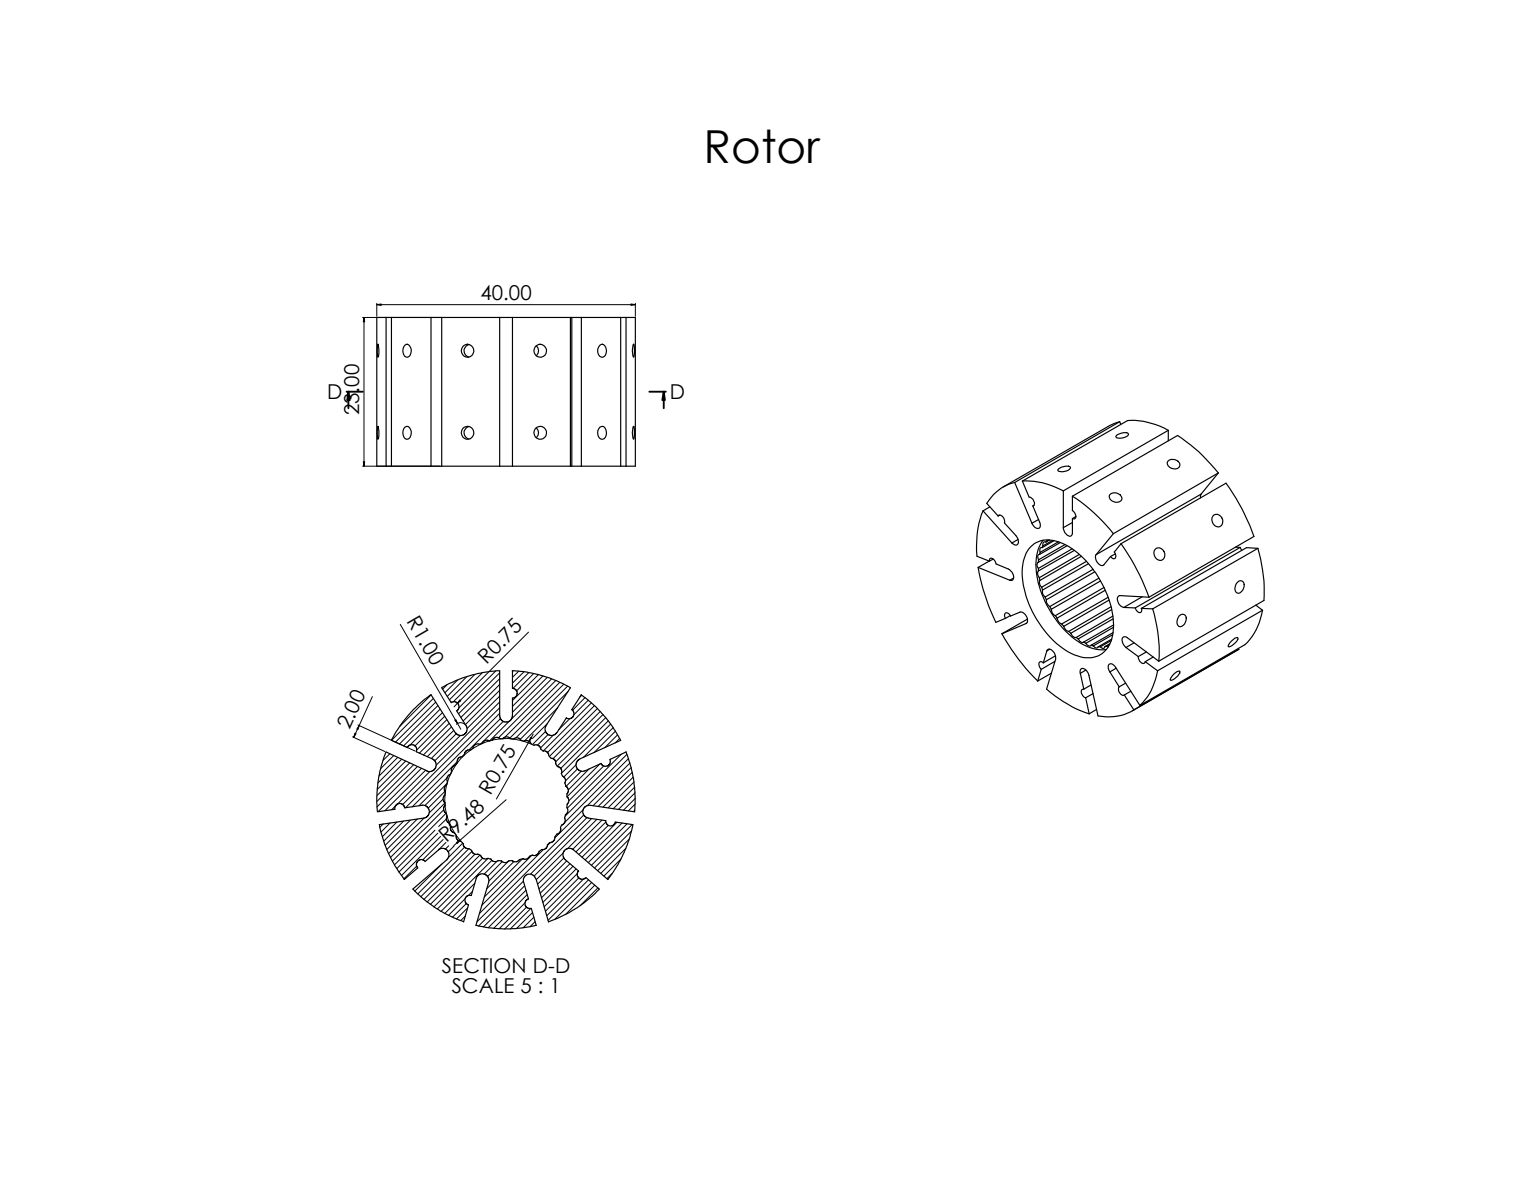
ISO-10303-21;
HEADER;
FILE_DESCRIPTION (('STEP AP214'),
    '1' );
FILE_NAME ('Rotor.step',
    '2026-10-18T20:16:25',
    ( '' ),
    ( '' ),
    'SwSTEP 2.0',
    'SolidWorks 2025',
    '' );
FILE_SCHEMA (( 'AUTOMOTIVE_DESIGN' ));
ENDSEC;

DATA;
#1=FACE_OUTER_BOUND ( 'NONE', #19385, .T. ) ;
#4=AXIS2_PLACEMENT_3D ( 'NONE', #28751, #28908, #7543 ) ;
#8=EDGE_LOOP ( 'NONE', ( #14143, #4167, #13185, #29281 ) ) ;
#11=AXIS2_PLACEMENT_3D ( 'NONE', #21550, #14547, #24043 ) ;
#13=EDGE_LOOP ( 'NONE', ( #16874, #3981 ) ) ;
#16=CARTESIAN_POINT ( 'NONE',  ( 6.437793815610356241, -6.974883619896809606, 1.500000000000001332 ) ) ;
#29=ORIENTED_EDGE ( 'NONE', *, *, #10327, .T. ) ;
#33=CARTESIAN_POINT ( 'NONE',  ( -3.912171961292007616, -8.637616862297829101, 1.500000000000001332 ) ) ;
#37=CARTESIAN_POINT ( 'NONE',  ( -14.84326473672822821, -8.425446036094903945, 20.06253562465620632 ) ) ;
#38=CARTESIAN_POINT ( 'NONE',  ( 0.000000000000000000, 0.000000000000000000, 1.500000000000001332 ) ) ;
#39=EDGE_CURVE ( 'NONE', #26631, #4645, #16306, .T. ) ;
#40=CARTESIAN_POINT ( 'NONE',  ( 4.967306913940536361, 16.28142803850090203, 6.973843882838223429 ) ) ;
#43=ORIENTED_EDGE ( 'NONE', *, *, #8838, .F. ) ;
#45=EDGE_CURVE ( 'NONE', #5916, #3823, #10340, .T. ) ;
#48=CARTESIAN_POINT ( 'NONE',  ( -6.228680293130167911, 19.00574304797303782, 5.679672709359373073 ) ) ;
#49=ORIENTED_EDGE ( 'NONE', *, *, #24996, .T. ) ;
#53=DIRECTION ( 'NONE',  ( 0.8412535328311813165, -0.5406408174555974444, 0.000000000000000000 ) ) ;
#54=DIRECTION ( 'NONE',  ( 0.000000000000000000, 0.000000000000000000, 1.000000000000000000 ) ) ;
#55=ORIENTED_EDGE ( 'NONE', *, *, #18763, .T. ) ;
#56=ORIENTED_EDGE ( 'NONE', *, *, #27505, .T. ) ;
#60=ORIENTED_EDGE ( 'NONE', *, *, #10139, .T. ) ;
#61=CARTESIAN_POINT ( 'NONE',  ( -0.02177409673011774377, -17.02558975896787885, 19.96783386855779341 ) ) ;
#64=CARTESIAN_POINT ( 'NONE',  ( -9.983339604393949074, -17.35078046477759983, 7.441806358946449151 ) ) ;
#65=FACE_OUTER_BOUND ( 'NONE', #13496, .T. ) ;
#66=CARTESIAN_POINT ( 'NONE',  ( 1.363408835038997458, -19.97112866468682668, 19.47783254395485031 ) ) ;
#68=EDGE_CURVE ( 'NONE', #8257, #20089, #6832, .T. ) ;
#70=CARTESIAN_POINT ( 'NONE',  ( 0.000000000000000000, 13.00000000000001421, 1.500000000000001332 ) ) ;
#71=CARTESIAN_POINT ( 'NONE',  ( 14.24237608451263171, 14.06627278277045257, 19.69140814234746273 ) ) ;
#73=ORIENTED_EDGE ( 'NONE', *, *, #24989, .F. ) ;
#75=DIRECTION ( 'NONE',  ( 0.000000000000000000, 0.000000000000000000, 1.000000000000000000 ) ) ;
#76=CARTESIAN_POINT ( 'NONE',  ( -17.59891439103365585, -9.538503746949022144, 6.672349528511551497 ) ) ;
#77=CARTESIAN_POINT ( 'NONE',  ( -13.11527592942575282, -10.04126165406389326, 1.500000000000000000 ) ) ;
#80=EDGE_CURVE ( 'NONE', #24431, #1715, #12846, .T. ) ;
#84=ORIENTED_EDGE ( 'NONE', *, *, #27745, .T. ) ;
#86=DIRECTION ( 'NONE',  ( 0.000000000000000000, 0.000000000000000000, -1.000000000000000000 ) ) ;
#87=VECTOR ( 'NONE', #19138, 1000.000000000000000 ) ;
#90=CARTESIAN_POINT ( 'NONE',  ( 15.47797589786116923, -7.092492006142040673, 19.96783386855779341 ) ) ;
#91=CARTESIAN_POINT ( 'NONE',  ( 6.171684994647412381, 19.04275422834224685, 6.211014596808754007 ) ) ;
#95=CARTESIAN_POINT ( 'NONE',  ( 11.67645754117908830, 12.46194352177089293, 6.892848776733236704 ) ) ;
#96=EDGE_CURVE ( 'NONE', #21713, #6692, #24023, .T. ) ;
#97=FACE_OUTER_BOUND ( 'NONE', #28084, .T. ) ;
#100=CARTESIAN_POINT ( 'NONE',  ( 0.000000000000000000, 0.000000000000000000, 1.500000000000001332 ) ) ;
#104=CARTESIAN_POINT ( 'NONE',  ( -18.38748676655956515, -7.913428453147655084, 6.018569869498933578 ) ) ;
#105=CARTESIAN_POINT ( 'NONE',  ( 14.46116907065692736, 13.81605838820130394, 7.454606537396340826 ) ) ;
#106=CARTESIAN_POINT ( 'NONE',  ( 0.06889080212831104333, -17.02733034922398758, 5.940635272151477686 ) ) ;
#108=LINE ( 'NONE', #21001, #12544 ) ;
#109=CARTESIAN_POINT ( 'NONE',  ( -19.94989956810792009, 1.646935350084928418, 19.89182036555910571 ) ) ;
#112=CARTESIAN_POINT ( 'NONE',  ( 11.47892014274828654, -16.39977715623752275, 20.25542030744407640 ) ) ;
#113=CIRCLE ( 'NONE', #24448, 0.7500000000000007772 ) ;
#115=VERTEX_POINT ( 'NONE', #22003 ) ;
#116=EDGE_LOOP ( 'NONE', ( #16345, #15698, #26338, #11828 ) ) ;
#117=CARTESIAN_POINT ( 'NONE',  ( 4.695984468547702129, 19.44110619659980799, 20.15039051365864253 ) ) ;
#122=CARTESIAN_POINT ( 'NONE',  ( -10.72135862580927146, -16.90494006806149940, 7.632642797338977658 ) ) ;
#125=CARTESIAN_POINT ( 'NONE',  ( 18.71580048965418541, -7.100988023106708624, 19.03762469184452755 ) ) ;
#126=CARTESIAN_POINT ( 'NONE',  ( 16.55849529797290032, 4.179294809495488039, 19.14333282897057842 ) ) ;
#127=EDGE_CURVE ( 'NONE', #8705, #8129, #11228, .T. ) ;
#130=EDGE_CURVE ( 'NONE', #28271, #10764, #20221, .T. ) ;
#133=ORIENTED_EDGE ( 'NONE', *, *, #19082, .T. ) ;
#134=CARTESIAN_POINT ( 'NONE',  ( 7.706848733600953238, 5.524309650260795124, 1.500000000000001332 ) ) ;
#135=CARTESIAN_POINT ( 'NONE',  ( -12.90456292687989759, 11.10871050118981529, 20.05479082170252525 ) ) ;
#136=CARTESIAN_POINT ( 'NONE',  ( -9.972083266784119715, -17.35726207598482773, 18.56793045041961321 ) ) ;
#137=CARTESIAN_POINT ( 'NONE',  ( -15.05112753842527162, -8.020416455032004066, 20.34789198813115263 ) ) ;
#139=CARTESIAN_POINT ( 'NONE',  ( 1.767905995611233072, -16.98559759804142288, 19.61324152429826739 ) ) ;
#140=CARTESIAN_POINT ( 'NONE',  ( 16.82202058066696537, 2.664153601443035146, 18.49267272388512140 ) ) ;
#143=CARTESIAN_POINT ( 'NONE',  ( 11.01999061743883956, -16.71182566173002826, 7.652108011868850035 ) ) ;
#144=CARTESIAN_POINT ( 'NONE',  ( 8.480328572437745294, -4.608906612435629491, 21.50000000000000000 ) ) ;
#147=LINE ( 'NONE', #19489, #17289 ) ;
#149=CARTESIAN_POINT ( 'NONE',  ( 1.000000000000008438, 13.00000000000001421, 1.500000000000001332 ) ) ;
#150=CARTESIAN_POINT ( 'NONE',  ( 2.878478920843521749, -0.8451976705243363641, 24.50000000000000000 ) ) ;
#151=CARTESIAN_POINT ( 'NONE',  ( 12.00212711880201510, 12.12705342296112221, 7.545655578832108468 ) ) ;
#153=CARTESIAN_POINT ( 'NONE',  ( -5.488535287689156661, 19.23255048776057308, 5.775318986477953054 ) ) ;
#154=VERTEX_POINT ( 'NONE', #22460 ) ;
#160=VERTEX_POINT ( 'NONE', #4060 ) ;
#161=CARTESIAN_POINT ( 'NONE',  ( 16.17271416092067682, -5.480318835022405466, 6.995624166085161910 ) ) ;
#174=VECTOR ( 'NONE', #2091, 1000.000000000000000 ) ;
#178=DIRECTION ( 'NONE',  ( 1.000000000000000000, 0.000000000000000000, 0.000000000000000000 ) ) ;
#183=CARTESIAN_POINT ( 'NONE',  ( 4.641725321133337800, 16.38498716464899019, 5.848946451764561516 ) ) ;
#189=EDGE_CURVE ( 'NONE', #1099, #580, #18256, .T. ) ;
#194=VERTEX_POINT ( 'NONE', #13123 ) ;
#195=DIRECTION ( 'NONE',  ( 0.000000000000000000, 0.000000000000000000, 1.000000000000000000 ) ) ;
#197=ORIENTED_EDGE ( 'NONE', *, *, #29811, .T. ) ;
#198=ADVANCED_FACE ( 'NONE', ( #25436 ), #29650, .F. ) ;
#199=ORIENTED_EDGE ( 'NONE', *, *, #12643, .T. ) ;
#200=CARTESIAN_POINT ( 'NONE',  ( -9.658933677579515376, -17.51307076256854600, 6.392525840300335105 ) ) ;
#203=VERTEX_POINT ( 'NONE', #17802 ) ;
#205=CARTESIAN_POINT ( 'NONE',  ( -0.1973194101962232605, -20.01708124257648791, 20.19668224736330941 ) ) ;
#208=DIRECTION ( 'NONE',  ( 0.000000000000000000, 0.000000000000000000, -1.000000000000000000 ) ) ;
#209=CARTESIAN_POINT ( 'NONE',  ( 4.045242219987651211, 16.55840560649980731, 18.34798005863078885 ) ) ;
#211=CARTESIAN_POINT ( 'NONE',  ( 0.8978415369256412815, -19.99755156235223552, 18.50655187082627862 ) ) ;
#212=EDGE_LOOP ( 'NONE', ( #3421, #739, #13868, #11454 ) ) ;
#214=EDGE_CURVE ( 'NONE', #13827, #7727, #27159, .T. ) ;
#216=FACE_OUTER_BOUND ( 'NONE', #25286, .T. ) ;
#220=FACE_OUTER_BOUND ( 'NONE', #17515, .T. ) ;
#221=CARTESIAN_POINT ( 'NONE',  ( -6.449126838413862473, 15.81136745782587383, 6.995624166085161910 ) ) ;
#225=CARTESIAN_POINT ( 'NONE',  ( -18.38748676655957937, -7.913428453147655084, 18.71435384576123440 ) ) ;
#230=AXIS2_PLACEMENT_3D ( 'NONE', #30774, #53, #30611 ) ;
#235=CARTESIAN_POINT ( 'NONE',  ( 11.21631477658334042, -16.55933310271405645, 20.34789198813115618 ) ) ;
#239=CARTESIAN_POINT ( 'NONE',  ( 18.21588581002257001, -8.300927319590597264, 18.39701043959520987 ) ) ;
#240=CARTESIAN_POINT ( 'NONE',  ( 5.984782097461514461, 19.10229623552459088, 5.940635272151477686 ) ) ;
#242=DIRECTION ( 'NONE',  ( 0.000000000000000000, 0.000000000000000000, 1.000000000000000000 ) ) ;
#245=CARTESIAN_POINT ( 'NONE',  ( -0.4564504349075055867, 9.471281197126600659, 13.00000000000000178 ) ) ;
#249=EDGE_CURVE ( 'NONE', #25840, #22179, #829, .T. ) ;
#250=CARTESIAN_POINT ( 'NONE',  ( 0.000000000000000000, 0.000000000000000000, 21.50000000000000000 ) ) ;
#255=CARTESIAN_POINT ( 'NONE',  ( -18.32589276785170185, -8.054604467211150975, 7.429667576816606278 ) ) ;
#256=AXIS2_PLACEMENT_3D ( 'NONE', #17662, #8160, #8483 ) ;
#257=DIRECTION ( 'NONE',  ( 0.000000000000000000, 0.000000000000000000, 1.000000000000000000 ) ) ;
#266=EDGE_CURVE ( 'NONE', #6035, #4843, #28573, .T. ) ;
#267=DIRECTION ( 'NONE',  ( 1.000000000000000000, 0.000000000000000000, 0.000000000000000000 ) ) ;
#269=ORIENTED_EDGE ( 'NONE', *, *, #9974, .T. ) ;
#271=LINE ( 'NONE', #18686, #17607 ) ;
#277=ORIENTED_EDGE ( 'NONE', *, *, #12266, .F. ) ;
#278=CARTESIAN_POINT ( 'NONE',  ( 18.65245237681030588, -7.265846841151810231, 19.97651184436794125 ) ) ;
#279=CARTESIAN_POINT ( 'NONE',  ( 16.55484456677775640, 4.196195780087080607, 19.25672174529527325 ) ) ;
#283=VECTOR ( 'NONE', #6940, 1000.000000000000000 ) ;
#286=CARTESIAN_POINT ( 'NONE',  ( -14.75808792347767628, 13.52460813173914467, 18.90679857307105749 ) ) ;
#287=CARTESIAN_POINT ( 'NONE',  ( -7.919226493207297324, -15.11997014267743289, 18.64703902303423178 ) ) ;
#290=CYLINDRICAL_SURFACE ( 'NONE', #21952, 0.7500000000000006661 ) ;
#294=CARTESIAN_POINT ( 'NONE',  ( -19.73562743738982306, 3.350138464993962284, 18.80699882434806369 ) ) ;
#296=VECTOR ( 'NONE', #25590, 1000.000000000000000 ) ;
#297=CARTESIAN_POINT ( 'NONE',  ( 14.88222593340886668, 13.36111339922579866, 20.34789198813115263 ) ) ;
#298=CYLINDRICAL_SURFACE ( 'NONE', #9820, 0.7500000000000004441 ) ;
#302=DIRECTION ( 'NONE',  ( -0.8412535328311813165, 0.5406408174555974444, 0.000000000000000000 ) ) ;
#304=CARTESIAN_POINT ( 'NONE',  ( -5.119216485953539397, 16.24645747311530641, 7.557577766377196582 ) ) ;
#305=CARTESIAN_POINT ( 'NONE',  ( -6.437683520590124608, 6.962021646281596254, 21.50000000000000000 ) ) ;
#308=ORIENTED_EDGE ( 'NONE', *, *, #27638, .F. ) ;
#310=CARTESIAN_POINT ( 'NONE',  ( -4.668110441710642711, -19.44758969394387194, 24.50000000000000000 ) ) ;
#311=CARTESIAN_POINT ( 'NONE',  ( 7.028330626922776325, 10.93629592680536966, 24.50000000000000000 ) ) ;
#312=ORIENTED_EDGE ( 'NONE', *, *, #28685, .F. ) ;
#314=CARTESIAN_POINT ( 'NONE',  ( 8.637616862297841536, -3.912171961291982747, 13.00000000000000178 ) ) ;
#315=VERTEX_POINT ( 'NONE', #30412 ) ;
#316=CARTESIAN_POINT ( 'NONE',  ( 16.17688602565676348, -5.469326772727310271, 6.341840715582230281 ) ) ;
#318=CARTESIAN_POINT ( 'NONE',  ( 0.7836604620899298990, -17.02735026737547841, 18.34798005863078885 ) ) ;
#321=VERTEX_POINT ( 'NONE', #30556 ) ;
#324=DIRECTION ( 'NONE',  ( 1.000000000000000000, 0.000000000000000000, 0.000000000000000000 ) ) ;
#328=CYLINDRICAL_SURFACE ( 'NONE', #23812, 9.482273699623480212 ) ;
#332=EDGE_CURVE ( 'NONE', #21638, #2008, #29122, .T. ) ;
#336=CARTESIAN_POINT ( 'NONE',  ( 16.91972452348793610, -3.442972353390052920, 1.500000000000000000 ) ) ;
#337=VECTOR ( 'NONE', #30659, 1000.000000000000000 ) ;
#339=FACE_OUTER_BOUND ( 'NONE', #26193, .T. ) ;
#341=CARTESIAN_POINT ( 'NONE',  ( 5.015798959889809616, 16.26549279019889127, 6.519181285484532573 ) ) ;
#343=DIRECTION ( 'NONE',  ( -0.000000000000000000, -0.000000000000000000, 1.000000000000000000 ) ) ;
#345=CARTESIAN_POINT ( 'NONE',  ( 19.63503467057051566, 3.804509661152916333, 7.454606537396342603 ) ) ;
#348=ORIENTED_EDGE ( 'NONE', *, *, #25359, .F. ) ;
#351=FACE_OUTER_BOUND ( 'NONE', #19038, .T. ) ;
#354=CARTESIAN_POINT ( 'NONE',  ( -10.51513057463695233, -17.01270198993486460, 7.652108011868850035 ) ) ;
#357=VERTEX_POINT ( 'NONE', #453 ) ;
#359=CARTESIAN_POINT ( 'NONE',  ( -0.2073672225646059353, -17.02047435233534145, 19.56050940960062690 ) ) ;
#362=CARTESIAN_POINT ( 'NONE',  ( -7.796062812047482637, -15.18940472835275202, 6.131018562779544823 ) ) ;
#363=DIRECTION ( 'NONE',  ( -0.000000000000000000, -0.000000000000000000, 1.000000000000000000 ) ) ;
#364=CARTESIAN_POINT ( 'NONE',  ( 1.771654956907828593, -16.98531529776322202, 19.58863275299554019 ) ) ;
#366=EDGE_CURVE ( 'NONE', #13283, #3383, #19165, .T. ) ;
#367=CARTESIAN_POINT ( 'NONE',  ( 18.44250036706182883, -7.738792361249056562, 5.679672709359370408 ) ) ;
#368=FACE_OUTER_BOUND ( 'NONE', #3082, .T. ) ;
#369=CARTESIAN_POINT ( 'NONE',  ( 12.30438418247798538, 11.79938075381829066, 18.34838970509067479 ) ) ;
#370=FACE_OUTER_BOUND ( 'NONE', #17110, .T. ) ;
#372=EDGE_LOOP ( 'NONE', ( #10343, #19396, #30364, #16527 ) ) ;
#373=CIRCLE ( 'NONE', #4356, 0.9999999999999983347 ) ;
#377=CARTESIAN_POINT ( 'NONE',  ( -18.02600256144196322, -8.705149951716492751, 5.652605728828375753 ) ) ;
#378=CARTESIAN_POINT ( 'NONE',  ( -6.670428619809865900, 18.87372120578243795, 5.951255046771932733 ) ) ;
#379=CARTESIAN_POINT ( 'NONE',  ( -19.93457197822652205, 1.617270501065028565, 7.161525567826883432 ) ) ;
#382=CARTESIAN_POINT ( 'NONE',  ( -5.544451647051928944, 16.11829164193971664, 20.34789198813115263 ) ) ;
#383=LINE ( 'NONE', #24396, #15077 ) ;
#387=AXIS2_PLACEMENT_3D ( 'NONE', #10424, #20235, #11043 ) ;
#389=CARTESIAN_POINT ( 'NONE',  ( -5.000852292258041842, 19.36469665082833913, 19.47728749465736797 ) ) ;
#397=ADVANCED_FACE ( 'NONE', ( #26495 ), #10383, .T. ) ;
#399=CARTESIAN_POINT ( 'NONE',  ( 5.016833900951455760, 16.26516650762552629, 19.45164628100866722 ) ) ;
#400=AXIS2_PLACEMENT_3D ( 'NONE', #13486, #9091, #27970 ) ;
#402=VECTOR ( 'NONE', #2368, 1000.000000000000114 ) ;
#410=CARTESIAN_POINT ( 'NONE',  ( -18.36135251343596764, -7.973951480934441172, 7.359006845440219102 ) ) ;
#413=CARTESIAN_POINT ( 'NONE',  ( 14.20332585465778941, 14.08077620357340720, 6.919864475265769421 ) ) ;
#414=EDGE_CURVE ( 'NONE', #2072, #12805, #10900, .T. ) ;
#415=CARTESIAN_POINT ( 'NONE',  ( -0.08542884365699662808, -20.01766063302414622, 5.749228751562096562 ) ) ;
#420=ORIENTED_EDGE ( 'NONE', *, *, #14601, .T. ) ;
#424=CARTESIAN_POINT ( 'NONE',  ( -7.869584159753960861, 10.39565510934976977, 1.500000000000001332 ) ) ;
#425=CARTESIAN_POINT ( 'NONE',  ( 5.041560023644209743, 19.35451993181656860, 7.626218077512944227 ) ) ;
#428=ORIENTED_EDGE ( 'NONE', *, *, #24835, .F. ) ;
#435=CARTESIAN_POINT ( 'NONE',  ( 15.37106698384762993, 12.82394120857654052, 20.05479082170252525 ) ) ;
#437=CARTESIAN_POINT ( 'NONE',  ( -11.28665222577991578, -16.53262428680031704, 6.211014596808754007 ) ) ;
#439=CARTESIAN_POINT ( 'NONE',  ( 18.73437065802030332, -7.051821425362959417, 19.25672174529527325 ) ) ;
#440=CARTESIAN_POINT ( 'NONE',  ( -15.42727847259664564, 12.72856271945105178, 20.34789198813115263 ) ) ;
#446=AXIS2_PLACEMENT_3D ( 'NONE', #2104, #16459, #7100 ) ;
#452=CARTESIAN_POINT ( 'NONE',  ( -6.485206790418931888, 15.79815780198024910, 19.58863275299554019 ) ) ;
#453=CARTESIAN_POINT ( 'NONE',  ( -10.51100883930069863, -17.01524884273342053, 5.652196082369965069 ) ) ;
#456=CARTESIAN_POINT ( 'NONE',  ( -7.857295329535767259, -15.15488436941561368, 18.73743063545763121 ) ) ;
#458=CARTESIAN_POINT ( 'NONE',  ( 11.23874228076938664, -11.06161525231356713, 24.50000000000000000 ) ) ;
#459=CYLINDRICAL_SURFACE ( 'NONE', #7899, 0.7499999999999988898 ) ;
#461=CARTESIAN_POINT ( 'NONE',  ( 9.833055564703258256, -13.92194044488497440, 5.651989602109218858 ) ) ;
#464=CARTESIAN_POINT ( 'NONE',  ( -13.42620032052775692, 10.50496109755573748, 7.652108011868850035 ) ) ;
#466=VERTEX_POINT ( 'NONE', #10733 ) ;
#467=ORIENTED_EDGE ( 'NONE', *, *, #5596, .F. ) ;
#470=CARTESIAN_POINT ( 'NONE',  ( 18.71829317531096137, -7.044536951825319804, 19.48477075383301482 ) ) ;
#476=CARTESIAN_POINT ( 'NONE',  ( 19.74251403343738076, 3.198927889078825970, 18.34798005863226678 ) ) ;
#485=LINE ( 'NONE', #28719, #30455 ) ;
#487=CARTESIAN_POINT ( 'NONE',  ( 0.7220001660362483920, 9.454746441592963180, 21.50000000000000000 ) ) ;
#493=ORIENTED_EDGE ( 'NONE', *, *, #4835, .T. ) ;
#497=CARTESIAN_POINT ( 'NONE',  ( -1.000000000000008438, 19.97498435543819539, 24.50000000000000000 ) ) ;
#499=CARTESIAN_POINT ( 'NONE',  ( -15.13309390500916862, -7.848982836665745921, 20.34789198813115263 ) ) ;
#500=FACE_OUTER_BOUND ( 'NONE', #7541, .T. ) ;
#515=CIRCLE ( 'NONE', #3019, 9.482273699623480212 ) ;
#516=ORIENTED_EDGE ( 'NONE', *, *, #6379, .T. ) ;
#524=CARTESIAN_POINT ( 'NONE',  ( 14.19872765237045442, 14.11031447301239972, 19.36813350477385143 ) ) ;
#529=CARTESIAN_POINT ( 'NONE',  ( -6.227270323482350101, 15.89124769393590952, 7.366751648393900176 ) ) ;
#530=CARTESIAN_POINT ( 'NONE',  ( -19.85983307072121917, 2.367331911061644867, 7.652108011868850923 ) ) ;
#531=CARTESIAN_POINT ( 'NONE',  ( -18.41388790264795361, -7.851569931599773788, 18.80699882434806369 ) ) ;
#536=CARTESIAN_POINT ( 'NONE',  ( 7.856594496258195726, 4.390207617113981442, 21.50000000000000000 ) ) ;
#537=CARTESIAN_POINT ( 'NONE',  ( -5.971396161871752817, 19.08775596758252036, 20.34789198813115263 ) ) ;
#538=CARTESIAN_POINT ( 'NONE',  ( -14.93957691572895818, 13.32381478560234456, 7.429667576816606278 ) ) ;
#539=CARTESIAN_POINT ( 'NONE',  ( 0.7788148816922453310, -17.02744011591805062, 7.652108011868850923 ) ) ;
#540=VERTEX_POINT ( 'NONE', #28613 ) ;
#542=CARTESIAN_POINT ( 'NONE',  ( 18.26182835180409825, -8.199456719779961489, 18.36582235739946611 ) ) ;
#550=CARTESIAN_POINT ( 'NONE',  ( -18.04156136322729864, -8.631457789788587576, 5.652196082369963293 ) ) ;
#553=CIRCLE ( 'NONE', #9509, 9.482273699623480212 ) ;
#554=CARTESIAN_POINT ( 'NONE',  ( 4.608906612435600181, 7.730328572437758616, 1.500000000000001332 ) ) ;
#555=FACE_OUTER_BOUND ( 'NONE', #28008, .T. ) ;
#560=CARTESIAN_POINT ( 'NONE',  ( -0.2365265214052943432, -17.01953242238517916, 6.641371103590088865 ) ) ;
#561=CARTESIAN_POINT ( 'NONE',  ( -17.20435420003449423, -1.463329469628170898, -0.6213203435596476032 ) ) ;
#562=DIRECTION ( 'NONE',  ( 0.000000000000000000, 0.000000000000000000, 1.000000000000000000 ) ) ;
#565=ORIENTED_EDGE ( 'NONE', *, *, #7868, .T. ) ;
#567=DIRECTION ( 'NONE',  ( -0.000000000000000000, -0.000000000000000000, -1.000000000000000000 ) ) ;
#573=ORIENTED_EDGE ( 'NONE', *, *, #29979, .F. ) ;
#575=EDGE_CURVE ( 'NONE', #3557, #18473, #9892, .T. ) ;
#576=CIRCLE ( 'NONE', #3574, 0.7500000000000006661 ) ;
#577=CARTESIAN_POINT ( 'NONE',  ( 12.83215063165194891, 11.19227874472585782, 20.05479082170252525 ) ) ;
#578=EDGE_CURVE ( 'NONE', #11969, #7607, #20097, .T. ) ;
#579=CARTESIAN_POINT ( 'NONE',  ( -11.35279153858833112, -16.48728705952963480, 6.864725433338323413 ) ) ;
#580=VERTEX_POINT ( 'NONE', #9273 ) ;
#581=CARTESIAN_POINT ( 'NONE',  ( 18.72830449397920560, -7.068013160879066170, 19.14333282897057842 ) ) ;
#585=DIRECTION ( 'NONE',  ( 0.000000000000000000, 0.000000000000000000, -1.000000000000000000 ) ) ;
#586=ADVANCED_FACE ( 'NONE', ( #19241 ), #28765, .F. ) ;
#588=AXIS2_PLACEMENT_3D ( 'NONE', #26078, #13640, #11903 ) ;
#590=EDGE_CURVE ( 'NONE', #23467, #4066, #18123, .T. ) ;
#592=CARTESIAN_POINT ( 'NONE',  ( -6.227270323482350989, 15.89124769393590597, 20.06253562465620632 ) ) ;
#593=CARTESIAN_POINT ( 'NONE',  ( -14.83674576813424295, 13.43848929326658492, 18.71435384576123440 ) ) ;
#595=ADVANCED_FACE ( 'NONE', ( #370 ), #16451, .F. ) ;
#596=CARTESIAN_POINT ( 'NONE',  ( -13.00999358272542494, -0.8602714556717691030, 24.50000000000000000 ) ) ;
#599=CARTESIAN_POINT ( 'NONE',  ( -16.96556290498877573, 1.647560670993253540, 5.652196082368482699 ) ) ;
#602=CARTESIAN_POINT ( 'NONE',  ( 11.02326084422093189, -16.70928013427648651, 5.657991946698900598 ) ) ;
#605=CARTESIAN_POINT ( 'NONE',  ( 9.013259606643902799, -14.43917691233135869, 6.782064869129510676 ) ) ;
#606=VERTEX_POINT ( 'NONE', #11765 ) ;
#609=CARTESIAN_POINT ( 'NONE',  ( 10.58932223943305573, -16.96688107778387078, 5.849008070840548079 ) ) ;
#611=LINE ( 'NONE', #7792, #3910 ) ;
#612=CARTESIAN_POINT ( 'NONE',  ( -15.57738559309033022, -6.860713375568460393, 6.714907520933425467 ) ) ;
#615=CARTESIAN_POINT ( 'NONE',  ( 1.000000000000008438, 13.00000000000001421, 1.500000000000001332 ) ) ;
#619=CARTESIAN_POINT ( 'NONE',  ( -17.67829152986844932, -9.353438168054493573, 18.73377938172347612 ) ) ;
#621=CARTESIAN_POINT ( 'NONE',  ( 19.77852387640474419, 3.085824932809442700, 5.657991946698900598 ) ) ;
#622=ORIENTED_EDGE ( 'NONE', *, *, #14546, .F. ) ;
#623=CARTESIAN_POINT ( 'NONE',  ( 15.53918631077679002, 12.61944498292910488, 6.420335371522007506 ) ) ;
#624=VERTEX_POINT ( 'NONE', #8174 ) ;
#625=CARTESIAN_POINT ( 'NONE',  ( 16.02044690728356002, -5.868896442471958963, 7.500147780736496017 ) ) ;
#632=ADVANCED_FACE ( 'NONE', ( #17214 ), #5675, .F. ) ;
#633=LINE ( 'NONE', #12185, #27245 ) ;
#637=CARTESIAN_POINT ( 'NONE',  ( -0.9307681286967850465, 9.436481611552762772, 21.50000000000000000 ) ) ;
#638=B_SPLINE_CURVE_WITH_KNOTS ( 'NONE', 3,
 ( #10726, #17744, #5592, #22265, #17916, #1379, #29923, #19940, #29760, #20545, #30064, #27580, #15559, #5738, #25226, #3871, #15086, #13394, #22884, #24604 ),
 .UNSPECIFIED., .F., .F.,
 ( 4, 2, 2, 2, 2, 2, 2, 2, 2, 4 ),
 ( 0.000000000000000000, 0.06250000000000163758, 0.1250000000000032752, 0.1875000000000049127, 0.2187500000000050793, 0.2500000000000052180, 0.3125000000000038858, 0.3750000000000024980, 0.4375000000000011657, 0.4999999999999999445 ),
 .UNSPECIFIED. ) ;
#644=CARTESIAN_POINT ( 'NONE',  ( -13.66451197432776965, 10.21236830578559918, 18.44527579819791185 ) ) ;
#658=CIRCLE ( 'NONE', #6650, 0.7500000000000006661 ) ;
#659=ORIENTED_EDGE ( 'NONE', *, *, #21172, .T. ) ;
#668=ORIENTED_EDGE ( 'NONE', *, *, #12074, .F. ) ;
#669=EDGE_LOOP ( 'NONE', ( #23306, #14404 ) ) ;
#670=CARTESIAN_POINT ( 'NONE',  ( 0.7453234696411419336, -17.02803278171227674, 18.34777357837151968 ) ) ;
#675=DIRECTION ( 'NONE',  ( 0.000000000000000000, 0.000000000000000000, 1.000000000000000000 ) ) ;
#678=CARTESIAN_POINT ( 'NONE',  ( 8.884323311075775109, 1.438332125858202692, 1.500000000000001332 ) ) ;
#679=CARTESIAN_POINT ( 'NONE',  ( 14.74830145734719089, 13.53506178006322891, 20.32367522806703874 ) ) ;
#681=VERTEX_POINT ( 'NONE', #999 ) ;
#684=CARTESIAN_POINT ( 'NONE',  ( -6.938992678473721476, 18.77645360485809789, 6.560937769032974209 ) ) ;
#685=CARTESIAN_POINT ( 'NONE',  ( 11.39819190923272707, -16.45610177916887551, 5.704143890883081269 ) ) ;
#690=LINE ( 'NONE', #10519, #25476 ) ;
#692=CARTESIAN_POINT ( 'NONE',  ( -14.74940038399478581, 13.53421240139457815, 7.080843742048788414 ) ) ;
#694=EDGE_LOOP ( 'NONE', ( #14179, #5997 ) ) ;
#696=DIRECTION ( 'NONE',  ( -0.9096319953545185522, 0.4154150130018859355, 0.000000000000000000 ) ) ;
#697=CARTESIAN_POINT ( 'NONE',  ( 4.045241160018716364, 16.55840174602107595, 5.652196082367002106 ) ) ;
#700=B_SPLINE_CURVE_WITH_KNOTS ( 'NONE', 3,
 ( #539, #9908, #28941, #10375, #29405, #8043, #19573, #24706, #22379, #17544, #10211, #12880, #15348, #17078, #3348, #1015, #7576, #26756, #29090, #24878 ),
 .UNSPECIFIED., .F., .F.,
 ( 4, 2, 2, 2, 2, 2, 2, 2, 2, 4 ),
 ( 0.000000000000000000, 0.06249999999999977102, 0.1249999999999995420, 0.1874999999999993061, 0.2187499999999992228, 0.2499999999999990841, 0.3124999999999992228, 0.3749999999999993894, 0.4374999999999995559, 0.4999999999999997224 ),
 .UNSPECIFIED. ) ;
#714=LINE ( 'NONE', #29114, #23280 ) ;
#720=CARTESIAN_POINT ( 'NONE',  ( 5.296161872597630271, 19.28602264385381204, 7.652108011868850035 ) ) ;
#723=ORIENTED_EDGE ( 'NONE', *, *, #19288, .F. ) ;
#725=CARTESIAN_POINT ( 'NONE',  ( -1.687027447297492211, -8.840471615930066918, 1.500000000000001332 ) ) ;
#728=CARTESIAN_POINT ( 'NONE',  ( 15.04472583903954153, 13.20536594261729491, 18.36582235739946611 ) ) ;
#735=CARTESIAN_POINT ( 'NONE',  ( -4.163336342344337027E-14, 1.387778780781445676E-14, 24.50000000000000000 ) ) ;
#736=AXIS2_PLACEMENT_3D ( 'NONE', #3166, #5043, #14695 ) ;
#739=ORIENTED_EDGE ( 'NONE', *, *, #127, .T. ) ;
#741=CARTESIAN_POINT ( 'NONE',  ( 16.55484456677776706, 4.196195780087079719, 6.560937769032974209 ) ) ;
#746=FACE_OUTER_BOUND ( 'NONE', #4867, .T. ) ;
#748=CARTESIAN_POINT ( 'NONE',  ( 9.027514758752763768, -14.43064536408543219, 6.864725433338323413 ) ) ;
#755=DIRECTION ( 'NONE',  ( -0.9096319953545185522, 0.4154150130018859355, 0.000000000000000000 ) ) ;
#758=DIRECTION ( 'NONE',  ( 0.000000000000000000, 0.000000000000000000, -1.000000000000000000 ) ) ;
#759=ORIENTED_EDGE ( 'NONE', *, *, #25056, .T. ) ;
#760=CARTESIAN_POINT ( 'NONE',  ( 12.35846533491531041, 11.73919094685904696, 7.652108011868850923 ) ) ;
#764=CARTESIAN_POINT ( 'NONE',  ( -9.636724589035640776, -17.52522580332708557, 19.48477075383299706 ) ) ;
#768=FACE_OUTER_BOUND ( 'NONE', #4197, .T. ) ;
#770=EDGE_CURVE ( 'NONE', #13440, #321, #29228, .T. ) ;
#771=CARTESIAN_POINT ( 'NONE',  ( 12.95659581195171484, 11.04149104205339782, 7.080843742048788414 ) ) ;
#773=CARTESIAN_POINT ( 'NONE',  ( 18.72830449397920560, -7.068013160879066170, 6.447548852708279377 ) ) ;
#777=ORIENTED_EDGE ( 'NONE', *, *, #17280, .T. ) ;
#778=VECTOR ( 'NONE', #21130, 1000.000000000000000 ) ;
#780=CARTESIAN_POINT ( 'NONE',  ( -8.743977807160097981, -3.668292057955969021, 1.500000000000001332 ) ) ;
#785=CARTESIAN_POINT ( 'NONE',  ( 9.085188746210622668, -14.39608436040015960, 19.77662771831109367 ) ) ;
#788=EDGE_LOOP ( 'NONE', ( #7005, #12290, #10451, #7760 ) ) ;
#803=EDGE_CURVE ( 'NONE', #26662, #24952, #7407, .T. ) ;
#805=AXIS2_PLACEMENT_3D ( 'NONE', #19527, #29041, #19830 ) ;
#809=ORIENTED_EDGE ( 'NONE', *, *, #12803, .T. ) ;
#810=AXIS2_PLACEMENT_3D ( 'NONE', #29533, #8170, #12389 ) ;
#811=VECTOR ( 'NONE', #29749, 1000.000000000000000 ) ;
#825=CARTESIAN_POINT ( 'NONE',  ( 0.000000000000000000, 0.000000000000000000, 21.50000000000000000 ) ) ;
#829=B_SPLINE_CURVE_WITH_KNOTS ( 'NONE', 3,
 ( #14168, #27929, #2173, #18565, #16516, #23839, #2018, #21343, #6847, #30856, #9500, #11688, #18868, #16207, #16370, #4814, #25727, #4355, #28382, #13880 ),
 .UNSPECIFIED., .F., .F.,
 ( 4, 2, 2, 2, 2, 2, 2, 2, 2, 4 ),
 ( 0.000000000000000000, 0.06250000000000092981, 0.1250000000000018596, 0.1875000000000027756, 0.2187500000000024980, 0.2500000000000022204, 0.3125000000000016653, 0.3750000000000010547, 0.4375000000000004996, 0.4999999999999998890 ),
 .UNSPECIFIED. ) ;
#830=EDGE_LOOP ( 'NONE', ( #15023, #29937 ) ) ;
#832=CARTESIAN_POINT ( 'NONE',  ( 10.50506478158603230, 13.32952022457704544, -0.6213203435596476032 ) ) ;
#834=CARTESIAN_POINT ( 'NONE',  ( 12.35846532919128116, 11.73919094318043221, 20.34789198813115263 ) ) ;
#836=EDGE_CURVE ( 'NONE', #12567, #28720, #7238, .T. ) ;
#837=EDGE_LOOP ( 'NONE', ( #26502, #26520, #16395, #29491 ) ) ;
#840=AXIS2_PLACEMENT_3D ( 'NONE', #28772, #2576, #21589 ) ;
#841=CARTESIAN_POINT ( 'NONE',  ( -17.99620775894062064, -8.766556869501982874, 7.643931100913408550 ) ) ;
#843=CARTESIAN_POINT ( 'NONE',  ( 10.52132926683980685, -13.44281371605820752, 6.041646659195333058 ) ) ;
#850=CARTESIAN_POINT ( 'NONE',  ( -1.438332125858111432, 8.884323311075791096, 1.500000000000001332 ) ) ;
#851=CARTESIAN_POINT ( 'NONE',  ( -14.94322542805485554, 13.31996107294430765, 5.862424720655265098 ) ) ;
#852=PLANE ( 'NONE',  #17635 ) ;
#856=CYLINDRICAL_SURFACE ( 'NONE', #7221, 0.7499999999999997780 ) ;
#860=VECTOR ( 'NONE', #3364, 1000.000000000000000 ) ;
#863=VERTEX_POINT ( 'NONE', #2675 ) ;
#866=CARTESIAN_POINT ( 'NONE',  ( 0.3518703668723790479, -19.99690444156084013, 20.34789198813115263 ) ) ;
#870=CARTESIAN_POINT ( 'NONE',  ( -19.71440049134194084, 3.368233808196385404, 18.84056766331481825 ) ) ;
#873=DIRECTION ( 'NONE',  ( 0.000000000000000000, 0.000000000000000000, 1.000000000000000000 ) ) ;
#875=VECTOR ( 'NONE', #3921, 1000.000000000000000 ) ;
#879=PLANE ( 'NONE',  #17324 ) ;
#881=DIRECTION ( 'NONE',  ( -1.000000000000000000, 0.000000000000000000, 0.000000000000000000 ) ) ;
#882=ORIENTED_EDGE ( 'NONE', *, *, #25559, .F. ) ;
#883=CARTESIAN_POINT ( 'NONE',  ( 7.730328572437743517, -4.608906612435629491, 1.500000000000001332 ) ) ;
#884=AXIS2_PLACEMENT_3D ( 'NONE', #30746, #18912, #29927 ) ;
#885=DIRECTION ( 'NONE',  ( -0.8412535328311804284, 0.5406408174555987767, 0.000000000000000000 ) ) ;
#887=EDGE_LOOP ( 'NONE', ( #3868, #22327 ) ) ;
#891=( LENGTH_UNIT ( ) NAMED_UNIT ( * ) SI_UNIT ( .MILLI., .METRE. ) );
#893=CARTESIAN_POINT ( 'NONE',  ( 9.634323311075775109, 1.438332125858202692, 1.500000000000001332 ) ) ;
#894=CIRCLE ( 'NONE', #1872, 0.7500000000000006661 ) ;
#895=CARTESIAN_POINT ( 'NONE',  ( 14.97043017101258577, 13.28903844302880266, 18.35377592296120497 ) ) ;
#896=B_SPLINE_CURVE_WITH_KNOTS ( 'NONE', 3,
 ( #27424, #24449, #15392, #24916, #17910, #27106, #10419, #1219, #17442, #15223, #5729, #19935, #10719, #3089, #7769, #29600, #22103, #29450 ),
 .UNSPECIFIED., .F., .F.,
 ( 4, 2, 2, 2, 2, 2, 2, 2, 4 ),
 ( 0.003174295595554312618, 0.003570702171545548417, 0.003967108747536783782, 0.004363515323528019581, 0.004759921899519255380, 0.005156328475510491179, 0.005552735051501726977, 0.005949141627492962776, 0.006345548203484198575 ),
 .UNSPECIFIED. ) ;
#899=CARTESIAN_POINT ( 'NONE',  ( 15.98415658701446773, -5.958736450466529000, 20.25542030744407640 ) ) ;
#900=CARTESIAN_POINT ( 'NONE',  ( 16.68770897235364714, 3.522277800415037685, 20.29915277494337644 ) ) ;
#904=CIRCLE ( 'NONE', #7825, 9.482273699623480212 ) ;
#908=ORIENTED_EDGE ( 'NONE', *, *, #23214, .F. ) ;
#912=B_SPLINE_SURFACE_WITH_KNOTS ( 'NONE', 3, 1, ( 
 ( #20892, #1721 ),
 ( #25123, #18111 ),
 ( #30417, #8743 ),
 ( #8909, #16074 ),
 ( #27626, #4067 ),
 ( #9055, #4210 ),
 ( #8463, #13733 ),
 ( #23223, #11236 ),
 ( #22779, #13284 ),
 ( #18433, #10949 ),
 ( #17965, #27323 ),
 ( #6250, #1583 ),
 ( #15450, #27934 ),
 ( #27474, #6562 ),
 ( #1877, #13128 ),
 ( #2491, #21500 ),
 ( #14491, #28223 ),
 ( #28389, #7014 ),
 ( #30705, #26190 ),
 ( #294, #21040 ),
 ( #9355, #7330 ),
 ( #6855, #16840 ),
 ( #2640, #30562 ),
 ( #25890, #19171 ),
 ( #23680, #21832 ),
 ( #16216, #18713 ),
 ( #28692, #2023 ),
 ( #12159, #28538 ),
 ( #6701, #11852 ),
 ( #4821, #23533 ),
 ( #16375, #4519 ) ),
 .UNSPECIFIED., .F., .F., .F.,
 ( 4, 3, 3, 3, 3, 3, 3, 3, 3, 3, 4 ),
 ( 2, 2 ),
 ( 0.000000000000000000, 0.05425176834609614362, 0.1085332949128348518, 0.1623767749169379715, 0.2157504826133058717, 0.2688657508888169789, 0.3218907763505471364, 0.3749548578363334772, 0.4282048033836237666, 0.4818374082110496448, 0.4999999999131650164 ),
 ( 0.000000000000000000, 1.000000000000000000 ),
 .UNSPECIFIED. ) ;
#913=CARTESIAN_POINT ( 'NONE',  ( 19.59419491516168321, 4.095680178559270246, 7.098451512883313441 ) ) ;
#914=CARTESIAN_POINT ( 'NONE',  ( -15.07239450771860056, 13.17334274624126422, 18.44501272782439827 ) ) ;
#915=AXIS2_PLACEMENT_3D ( 'NONE', #16296, #11613, #18792 ) ;
#916=AXIS2_PLACEMENT_3D ( 'NONE', #10436, #27126, #12313 ) ;
#917=CARTESIAN_POINT ( 'NONE',  ( -7.809214384344184801, -15.18204291278971496, 19.89182036555910571 ) ) ;
#920=FACE_OUTER_BOUND ( 'NONE', #25459, .T. ) ;
#922=CARTESIAN_POINT ( 'NONE',  ( 9.054000795813635705, -14.41483084819681615, 6.310736198168394928 ) ) ;
#925=CARTESIAN_POINT ( 'NONE',  ( 12.86767874445214055, -1.850092897552706894, 1.500000000000001332 ) ) ;
#929=LINE ( 'NONE', #17619, #19604 ) ;
#930=DIRECTION ( 'NONE',  ( -0.000000000000000000, -0.000000000000000000, -1.000000000000000000 ) ) ;
#933=DIRECTION ( 'NONE',  ( 1.000000000000000000, 0.000000000000000000, 0.000000000000000000 ) ) ;
#934=CARTESIAN_POINT ( 'NONE',  ( 6.237549684377459158, 19.00251437819605371, 6.913388067999410858 ) ) ;
#936=EDGE_LOOP ( 'NONE', ( #6511, #6269, #30437, #7742 ) ) ;
#940=CARTESIAN_POINT ( 'NONE',  ( -5.881244434206279514, -6.812559277181949646, 1.500000000000001332 ) ) ;
#943=CARTESIAN_POINT ( 'NONE',  ( 19.84141769772507402, 2.653416696629036675, 7.500898271101006820 ) ) ;
#950=VERTEX_POINT ( 'NONE', #12191 ) ;
#951=ADVANCED_FACE ( 'NONE', ( #21689 ), #328, .F. ) ;
#952=CARTESIAN_POINT ( 'NONE',  ( 4.316117848019423775, 19.54676362458759087, 6.672349528511551497 ) ) ;
#957=B_SPLINE_CURVE_WITH_KNOTS ( 'NONE', 3,
 ( #20118, #27608, #5770, #27144, #14969, #24482, #12648, #27299, #19967, #764, #10288, #19803, #8121, #29331, #15263, #7972, #17476, #17627 ),
 .UNSPECIFIED., .F., .F.,
 ( 4, 2, 2, 2, 2, 2, 2, 2, 4 ),
 ( 0.000000000000000000, 0.0003967869494442840357, 0.0007935738988885680713, 0.001190360848332851999, 0.001587147797777136143, 0.001983934747221420287, 0.002380721696665703997, 0.002777508646109988141, 0.003174295595554272285 ),
 .UNSPECIFIED. ) ;
#959=CARTESIAN_POINT ( 'NONE',  ( 10.26079415706018771, -17.18817258638080148, 19.45164628100866722 ) ) ;
#964=CARTESIAN_POINT ( 'NONE',  ( -13.78503626495110446, 10.05991541429405522, 18.56793045041961321 ) ) ;
#966=CARTESIAN_POINT ( 'NONE',  ( -13.00999358272542494, -0.8602714556717691030, 24.50000000000000000 ) ) ;
#970=CARTESIAN_POINT ( 'NONE',  ( -16.96496224101209194, 1.652369717150043549, 20.34789198813115263 ) ) ;
#971=CARTESIAN_POINT ( 'NONE',  ( 12.69259498021937382, 11.35795912679306063, 7.526951045817046548 ) ) ;
#972=DIRECTION ( 'NONE',  ( 0.000000000000000000, 0.000000000000000000, 1.000000000000000000 ) ) ;
#974=VECTOR ( 'NONE', #27914, 1000.000000000000000 ) ;
#982=ORIENTED_EDGE ( 'NONE', *, *, #8425, .T. ) ;
#983=EDGE_CURVE ( 'NONE', #14509, #24952, #16713, .T. ) ;
#984=VERTEX_POINT ( 'NONE', #21071 ) ;
#985=EDGE_CURVE ( 'NONE', #23990, #4772, #30594, .T. ) ;
#990=EDGE_CURVE ( 'NONE', #6958, #27304, #16554, .T. ) ;
#998=CARTESIAN_POINT ( 'NONE',  ( 1.121436987360518778, -17.01878714021720285, 5.704143890883081269 ) ) ;
#999=CARTESIAN_POINT ( 'NONE',  ( -5.971396161871753705, 19.08775596758252391, 7.652108011868850035 ) ) ;
#1000=EDGE_CURVE ( 'NONE', #203, #4677, #25923, .T. ) ;
#1001=VERTEX_POINT ( 'NONE', #4552 ) ;
#1002=EDGE_CURVE ( 'NONE', #25635, #16019, #6828, .T. ) ;
#1003=CARTESIAN_POINT ( 'NONE',  ( -9.310272263096074141, -14.25176022191445036, 18.90679857307105749 ) ) ;
#1005=CARTESIAN_POINT ( 'NONE',  ( -5.615427697021304176, 16.09608755218563303, 7.652108011868850035 ) ) ;
#1007=CARTESIAN_POINT ( 'NONE',  ( 10.65192122195201740, -13.34697535456212236, 6.341840715582230281 ) ) ;
#1009=CARTESIAN_POINT ( 'NONE',  ( -15.34307810681595896, 12.82926163924266660, 20.34789198813115263 ) ) ;
#1010=ORIENTED_EDGE ( 'NONE', *, *, #24861, .F. ) ;
#1012=CARTESIAN_POINT ( 'NONE',  ( -4.622016212553093695, -12.19167610014704906, 1.500000000000001332 ) ) ;
#1014=CARTESIAN_POINT ( 'NONE',  ( -13.30790957887532677, 10.64596135573641789, 5.657991946698900598 ) ) ;
#1015=CARTESIAN_POINT ( 'NONE',  ( 0.1624814966347698231, -17.02900520012292773, 5.848946451764563292 ) ) ;
#1018=CYLINDRICAL_SURFACE ( 'NONE', #7276, 9.482273699623480212 ) ;
#1020=ADVANCED_FACE ( 'NONE', ( #2831 ), #21857, .F. ) ;
#1027=ORIENTED_EDGE ( 'NONE', *, *, #5345, .F. ) ;
#1040=B_SPLINE_CURVE_WITH_KNOTS ( 'NONE', 3,
 ( #16024, #18829, #21137, #6657, #4166, #1985, #30215, #28346, #16174, #11647, #6973, #9156, #11797, #18669, #13992, #27731, #11507, #18382 ),
 .UNSPECIFIED., .F., .F.,
 ( 4, 2, 2, 2, 2, 2, 2, 2, 4 ),
 ( 0.003174295595554314786, 0.003570702171545546248, 0.003967108747536777710, 0.004363515323528009172, 0.004759921899519240635, 0.005156328475510472097, 0.005552735051501703559, 0.005949141627492935021, 0.006345548203484166483 ),
 .UNSPECIFIED. ) ;
#1047=CARTESIAN_POINT ( 'NONE',  ( 4.307942169702170254, 19.53053083060024164, 6.523620417364449864 ) ) ;
#1050=CARTESIAN_POINT ( 'NONE',  ( 0.3567158762617958501, -19.99681059701335073, 5.652196082369963293 ) ) ;
#1055=ADVANCED_FACE ( 'NONE', ( #7822 ), #17334, .F. ) ;
#1057=CARTESIAN_POINT ( 'NONE',  ( 15.43499236066653779, -3.229500095980124996, -0.6213203435596476032 ) ) ;
#1060=CARTESIAN_POINT ( 'NONE',  ( -16.88948989945504664, 2.193765388987378717, 7.500898271101006820 ) ) ;
#1064=LINE ( 'NONE', #19936, #27451 ) ;
#1066=CARTESIAN_POINT ( 'NONE',  ( -5.419526071899103847, 16.15737324489262150, 20.34789198813115974 ) ) ;
#1069=ORIENTED_EDGE ( 'NONE', *, *, #15299, .F. ) ;
#1072=CARTESIAN_POINT ( 'NONE',  ( 19.66823596311669675, 3.724077645907917677, 7.500147780736496017 ) ) ;
#1075=CARTESIAN_POINT ( 'NONE',  ( -9.228184491630887720, -14.30775539772383098, 7.267659094423555288 ) ) ;
#1079=CARTESIAN_POINT ( 'NONE',  ( 11.83189508704695392, -16.14673651688228873, 18.82680253904184298 ) ) ;
#1083=ORIENTED_EDGE ( 'NONE', *, *, #14308, .T. ) ;
#1087=ORIENTED_EDGE ( 'NONE', *, *, #30330, .F. ) ;
#1088=CYLINDRICAL_SURFACE ( 'NONE', #4116, 1.000000000000007772 ) ;
#1089=EDGE_CURVE ( 'NONE', #3823, #5916, #13380, .T. ) ;
#1090=DIRECTION ( 'NONE',  ( -0.000000000000000000, -0.000000000000000000, -1.000000000000000000 ) ) ;
#1092=CARTESIAN_POINT ( 'NONE',  ( 6.236311564447694522, 19.00292092786887110, 6.386539667786099272 ) ) ;
#1093=ORIENTED_EDGE ( 'NONE', *, *, #990, .F. ) ;
#1097=CARTESIAN_POINT ( 'NONE',  ( 14.29853178503251954, 14.00938365128603280, 6.131018562779544823 ) ) ;
#1098=CARTESIAN_POINT ( 'NONE',  ( 16.87995935610571507, 2.188012981718273853, 6.641371103590088865 ) ) ;
#1099=VERTEX_POINT ( 'NONE', #8461 ) ;
#1100=CARTESIAN_POINT ( 'NONE',  ( 16.09518941752841670, 6.251081041772567737, -0.6213203435596476032 ) ) ;
#1102=CARTESIAN_POINT ( 'NONE',  ( -13.38160118231794371, 10.55829203257429860, 18.34798005863078885 ) ) ;
#1107=DIRECTION ( 'NONE',  ( 0.000000000000000000, 0.000000000000000000, -1.000000000000000000 ) ) ;
#1121=CARTESIAN_POINT ( 'NONE',  ( -14.93932203929705871, 13.29757777824903897, 20.14992337338002670 ) ) ;
#1126=ORIENTED_EDGE ( 'NONE', *, *, #17165, .T. ) ;
#1128=DIRECTION ( 'NONE',  ( -0.000000000000000000, -0.000000000000000000, 1.000000000000000000 ) ) ;
#1130=VERTEX_POINT ( 'NONE', #6559 ) ;
#1136=CARTESIAN_POINT ( 'NONE',  ( -19.94474618696874302, 1.485631111656367853, 19.48477075383299706 ) ) ;
#1137=EDGE_LOOP ( 'NONE', ( #14626, #9572, #10175, #26189 ) ) ;
#1142=DIRECTION ( 'NONE',  ( 0.000000000000000000, 0.000000000000000000, 1.000000000000000000 ) ) ;
#1145=CARTESIAN_POINT ( 'NONE',  ( 14.84769773172387985, 13.42619037096054591, 20.34789198813115263 ) ) ;
#1147=VERTEX_POINT ( 'NONE', #6092 ) ;
#1148=CARTESIAN_POINT ( 'NONE',  ( -11.13550902248300467, -16.63501148641496030, 20.05479082170252525 ) ) ;
#1149=CARTESIAN_POINT ( 'NONE',  ( -17.77905984561984098, -9.199004478715986366, 7.441806358946449151 ) ) ;
#1150=CARTESIAN_POINT ( 'NONE',  ( -5.423201226159623189, 16.15625638772824502, 5.651492010659114662 ) ) ;
#1152=CARTESIAN_POINT ( 'NONE',  ( 11.93399590641349306, -16.07127689286907213, 6.447548852708279377 ) ) ;
#1164=CARTESIAN_POINT ( 'NONE',  ( -14.72475726066618407, 13.56098618572340442, 6.310736198168394928 ) ) ;
#1165=ADVANCED_FACE ( 'NONE', ( #8741 ), #16133, .T. ) ;
#1171=CARTESIAN_POINT ( 'NONE',  ( -9.356685943497543789, -14.22000274044912160, 6.974106381145714018 ) ) ;
#1173=ORIENTED_EDGE ( 'NONE', *, *, #8480, .F. ) ;
#1174=CARTESIAN_POINT ( 'NONE',  ( -10.82521593960875528, 5.400395169024524655, 1.500000000000001332 ) ) ;
#1175=B_SPLINE_SURFACE_WITH_KNOTS ( 'NONE', 3, 1, ( 
 ( #26290, #11788 ),
 ( #9611, #5083 ),
 ( #21293, #28788 ),
 ( #7428, #21129 ),
 ( #7116, #16935 ),
 ( #16774, #4761 ),
 ( #21451, #26453 ),
 ( #16628, #14594 ),
 ( #28338, #9915 ),
 ( #12256, #12109 ),
 ( #19428, #24098 ),
 ( #25990, #4926 ),
 ( #21759, #2119 ),
 ( #26133, #399 ),
 ( #14443, #17084 ),
 ( #26611, #2439 ),
 ( #5238, #23945 ),
 ( #30648, #16474 ),
 ( #4619, #14268 ),
 ( #23787, #11960 ),
 ( #2591, #10382 ),
 ( #12886, #2903 ),
 ( #17403, #13035 ),
 ( #12725, #22065 ),
 ( #22525, #19727 ),
 ( #20039, #19896 ),
 ( #12421, #29097 ),
 ( #5542, #24409 ),
 ( #15044, #18287 ),
 ( #10531, #27808 ),
 ( #29413, #17551 ) ),
 .UNSPECIFIED., .F., .F., .F.,
 ( 4, 3, 3, 3, 3, 3, 3, 3, 3, 3, 4 ),
 ( 2, 2 ),
 ( 0.000000000000000000, 0.05425176834609614362, 0.1085332949128348518, 0.1623767749169379715, 0.2157504826133058717, 0.2688657508888169789, 0.3218907763505471364, 0.3749548578363334772, 0.4282048033836237666, 0.4818374082110496448, 0.4999999999131652384 ),
 ( 0.000000000000000000, 1.000000000000000000 ),
 .UNSPECIFIED. ) ;
#1178=CARTESIAN_POINT ( 'NONE',  ( 0.000000000000000000, 0.000000000000000000, 1.500000000000001332 ) ) ;
#1180=ORIENTED_EDGE ( 'NONE', *, *, #8394, .T. ) ;
#1182=EDGE_CURVE ( 'NONE', #25305, #3669, #9352, .T. ) ;
#1186=CARTESIAN_POINT ( 'NONE',  ( 16.74250988114177474, 3.198928528055117404, 18.34798005863078885 ) ) ;
#1188=VERTEX_POINT ( 'NONE', #2021 ) ;
#1190=DIRECTION ( 'NONE',  ( 0.000000000000000000, 0.000000000000000000, 1.000000000000000000 ) ) ;
#1198=ADVANCED_FACE ( 'NONE', ( #30415 ), #16212, .F. ) ;
#1204=ADVANCED_FACE ( 'NONE', ( #746 ), #459, .F. ) ;
#1206=FACE_OUTER_BOUND ( 'NONE', #15379, .T. ) ;
#1207=CIRCLE ( 'NONE', #5672, 0.7500000000000011102 ) ;
#1211=ORIENTED_EDGE ( 'NONE', *, *, #13206, .F. ) ;
#1213=CARTESIAN_POINT ( 'NONE',  ( 9.031466002702407181, -14.42835478804157390, 19.08155846658118904 ) ) ;
#1216=ORIENTED_EDGE ( 'NONE', *, *, #25747, .F. ) ;
#1217=ORIENTED_EDGE ( 'NONE', *, *, #11109, .T. ) ;
#1219=CARTESIAN_POINT ( 'NONE',  ( 17.92140030663551187, -8.878400182913017247, 6.913388067999403752 ) ) ;
#1223=CARTESIAN_POINT ( 'NONE',  ( -4.573988094335678767, 16.39521158297133852, 19.41069149716888020 ) ) ;
#1224=EDGE_LOOP ( 'NONE', ( #18742, #29323, #2067, #24627 ) ) ;
#1227=LINE ( 'NONE', #6051, #29164 ) ;
#1230=CARTESIAN_POINT ( 'NONE',  ( 16.70510464924394967, 3.421819763545496773, 5.678370764302467677 ) ) ;
#1235=DIRECTION ( 'NONE',  ( 1.000000000000000000, 0.000000000000000000, 0.000000000000000000 ) ) ;
#1239=FACE_OUTER_BOUND ( 'NONE', #5088, .T. ) ;
#1240=DIRECTION ( 'NONE',  ( 0.000000000000000000, 0.000000000000000000, 1.000000000000000000 ) ) ;
#1242=VERTEX_POINT ( 'NONE', #7485 ) ;
#1245=CARTESIAN_POINT ( 'NONE',  ( -4.718303904200451981, 16.35736724179926682, 7.176035686813569292 ) ) ;
#1251=EDGE_LOOP ( 'NONE', ( #20084, #3933, #13079, #18206 ) ) ;
#1253=CARTESIAN_POINT ( 'NONE',  ( 11.67039530559479843, 12.46804495696167692, 6.447548852708279377 ) ) ;
#1254=CARTESIAN_POINT ( 'NONE',  ( 16.82340201860978368, 2.653416696629036675, 7.500898271101006820 ) ) ;
#1255=VERTEX_POINT ( 'NONE', #2637 ) ;
#1256=CARTESIAN_POINT ( 'NONE',  ( 15.31102578509455903, 12.89549683364648835, 5.862424720655265098 ) ) ;
#1258=CYLINDRICAL_SURFACE ( 'NONE', #28879, 9.482273699623480212 ) ;
#1259=AXIS2_PLACEMENT_3D ( 'NONE', #19682, #29205, #29053 ) ;
#1263=CARTESIAN_POINT ( 'NONE',  ( 5.159688198573268991, 19.34150021954530274, 7.643931100913408550 ) ) ;
#1266=CARTESIAN_POINT ( 'NONE',  ( 6.262045289545328686, 18.99438835075423881, 19.21471108562414543 ) ) ;
#1270=CARTESIAN_POINT ( 'NONE',  ( 16.86926274317444552, 2.283828795636141162, 19.77662771831109367 ) ) ;
#1273=CARTESIAN_POINT ( 'NONE',  ( 15.54925513364909939, -6.943479002078030149, 7.429667576816606278 ) ) ;
#1274=CARTESIAN_POINT ( 'NONE',  ( -13.97362136398187538, 9.814707526993059261, 19.69140814234746273 ) ) ;
#1279=CARTESIAN_POINT ( 'NONE',  ( 9.864937699929955173, -13.90063973435163724, 5.652196082368482699 ) ) ;
#1281=CARTESIAN_POINT ( 'NONE',  ( -5.865338193562683600, 19.13956943172006220, 20.34789198813115263 ) ) ;
#1283=DIRECTION ( 'NONE',  ( 0.000000000000000000, 0.000000000000000000, -1.000000000000000000 ) ) ;
#1290=VERTEX_POINT ( 'NONE', #3249 ) ;
#1291=CIRCLE ( 'NONE', #19710, 1.000000000000008660 ) ;
#1292=VERTEX_POINT ( 'NONE', #17293 ) ;
#1303=DIRECTION ( 'NONE',  ( 1.000000000000000000, 0.000000000000000000, 0.000000000000000000 ) ) ;
#1305=CARTESIAN_POINT ( 'NONE',  ( -8.835414383224243551, -14.56605378991199196, 20.29090034784956131 ) ) ;
#1312=AXIS2_PLACEMENT_3D ( 'NONE', #15629, #1609, #6117 ) ;
#1313=DIRECTION ( 'NONE',  ( 1.000000000000000000, 0.000000000000000000, 0.000000000000000000 ) ) ;
#1318=FACE_OUTER_BOUND ( 'NONE', #10044, .T. ) ;
#1319=DIRECTION ( 'NONE',  ( 0.000000000000000000, 0.000000000000000000, -1.000000000000000000 ) ) ;
#1320=ORIENTED_EDGE ( 'NONE', *, *, #3335, .T. ) ;
#1323=CARTESIAN_POINT ( 'NONE',  ( -9.389232999038370053, -14.19758896559616979, 6.530762810602277924 ) ) ;
#1324=ORIENTED_EDGE ( 'NONE', *, *, #21960, .T. ) ;
#1325=CARTESIAN_POINT ( 'NONE',  ( -8.550548372801090480, -14.74545326687210434, 20.34789198813115263 ) ) ;
#1338=CARTESIAN_POINT ( 'NONE',  ( 12.98116905410817523, 11.01127998639621275, 19.66962785902261146 ) ) ;
#1339=CARTESIAN_POINT ( 'NONE',  ( 16.12178322344232129, -5.613588367463943740, 6.037360021877315575 ) ) ;
#1342=CARTESIAN_POINT ( 'NONE',  ( -17.05006382469673198, 0.8465830298419860789, 7.269896094239230777 ) ) ;
#1345=CARTESIAN_POINT ( 'NONE',  ( 4.608906612435600181, 7.730328572437758616, 1.500000000000001332 ) ) ;
#1347=LINE ( 'NONE', #3692, #2454 ) ;
#1348=CARTESIAN_POINT ( 'NONE',  ( 9.031466002689079176, -14.42835478804960303, 6.385774490351133537 ) ) ;
#1350=CARTESIAN_POINT ( 'NONE',  ( -8.978548835276082940, -14.47379921341572562, 20.22273502201483097 ) ) ;
#1354=VECTOR ( 'NONE', #16103, 1000.000000000000000 ) ;
#1355=ADVANCED_FACE ( 'NONE', ( #21970 ), #24617, .F. ) ;
#1363=CARTESIAN_POINT ( 'NONE',  ( 9.640932123821245980, -14.04859418178019759, 20.32222155561918697 ) ) ;
#1364=VERTEX_POINT ( 'NONE', #5132 ) ;
#1366=CARTESIAN_POINT ( 'NONE',  ( 15.94288127717318915, -6.058927977062414705, 20.29915277494337644 ) ) ;
#1367=CIRCLE ( 'NONE', #19785, 0.7500000000000006661 ) ;
#1368=CARTESIAN_POINT ( 'NONE',  ( 16.70665413472816496, 3.412884783584985815, 20.32367522806703874 ) ) ;
#1370=CARTESIAN_POINT ( 'NONE',  ( -10.62006778255435613, -16.96839658127461803, 18.35377592296120497 ) ) ;
#1373=CARTESIAN_POINT ( 'NONE',  ( -5.544451647051928944, 16.11829164193971664, 20.34789198813115263 ) ) ;
#1374=ADVANCED_FACE ( 'NONE', ( #920 ), #26827, .T. ) ;
#1377=EDGE_CURVE ( 'NONE', #14465, #15390, #21818, .T. ) ;
#1379=CARTESIAN_POINT ( 'NONE',  ( -16.84831847207179223, 2.450595477917709264, 19.96344307082652492 ) ) ;
#1381=AXIS2_PLACEMENT_3D ( 'NONE', #28177, #18216, #23028 ) ;
#1382=EDGE_CURVE ( 'NONE', #4772, #14537, #29775, .T. ) ;
#1385=CARTESIAN_POINT ( 'NONE',  ( 19.57830992477560272, 4.170884463583997892, 6.892848776733236704 ) ) ;
#1386=CARTESIAN_POINT ( 'NONE',  ( -13.16299300229363567, 10.81582545713520638, 18.39701043959520987 ) ) ;
#1387=AXIS2_PLACEMENT_3D ( 'NONE', #12324, #3117, #21827 ) ;
#1388=CARTESIAN_POINT ( 'NONE',  ( 1.307979816591920308, -17.01201364160250051, 5.759928666072750225 ) ) ;
#1389=EDGE_CURVE ( 'NONE', #6566, #2038, #8416, .T. ) ;
#1390=CARTESIAN_POINT ( 'NONE',  ( 16.74328841314636662, 3.194145055459935545, 20.34789198813115263 ) ) ;
#1391=DIRECTION ( 'NONE',  ( 0.000000000000000000, 0.000000000000000000, 1.000000000000000000 ) ) ;
#1392=CARTESIAN_POINT ( 'NONE',  ( 9.749114229549594057, -0.1262659238204522361, 1.500000000000001332 ) ) ;
#1395=EDGE_CURVE ( 'NONE', #29287, #2154, #4898, .T. ) ;
#1396=CIRCLE ( 'NONE', #28285, 1.000000000000004441 ) ;
#1399=AXIS2_PLACEMENT_3D ( 'NONE', #12089, #14577, #5219 ) ;
#1402=ADVANCED_FACE ( 'NONE', ( #8251, #17927, #1686 ), #10739, .T. ) ;
#1405=CARTESIAN_POINT ( 'NONE',  ( -5.147812317479952604, 19.34466387292043876, 7.176035686813569292 ) ) ;
#1406=ORIENTED_EDGE ( 'NONE', *, *, #6377, .F. ) ;
#1417=EDGE_CURVE ( 'NONE', #22306, #24939, #17759, .T. ) ;
#1425=EDGE_CURVE ( 'NONE', #11023, #8165, #6059, .T. ) ;
#1430=ORIENTED_EDGE ( 'NONE', *, *, #26299, .F. ) ;
#1431=CARTESIAN_POINT ( 'NONE',  ( 9.676137610658589239, -14.02562811695956313, 18.36582235739946611 ) ) ;
#1432=CARTESIAN_POINT ( 'NONE',  ( 19.76130408545751749, 3.194145055459935101, 20.34789198813115263 ) ) ;
#1435=CARTESIAN_POINT ( 'NONE',  ( 17.97060409579513163, -8.818932628521070072, 6.211014596808754007 ) ) ;
#1437=CARTESIAN_POINT ( 'NONE',  ( 4.982076346116049770, 19.38816267120398962, 20.29915277494337644 ) ) ;
#1441=B_SPLINE_SURFACE_WITH_KNOTS ( 'NONE', 3, 1, ( 
 ( #29652, #10011 ),
 ( #10154, #29183 ),
 ( #7990, #8289 ),
 ( #26541, #17333 ),
 ( #14675, #24179 ),
 ( #5642, #19983 ),
 ( #7669, #5485 ),
 ( #17171, #19826 ),
 ( #14987, #24499 ),
 ( #26692, #3145 ),
 ( #22161, #785 ),
 ( #22317, #17493 ),
 ( #24654, #3289 ),
 ( #959, #14833 ),
 ( #29501, #17645 ),
 ( #5789, #27780 ),
 ( #6247, #6091 ),
 ( #25439, #15602 ),
 ( #15756, #20444 ),
 ( #10777, #25277 ),
 ( #6558, #20889 ),
 ( #20291, #30414 ),
 ( #17805, #15927 ),
 ( #13281, #23220 ),
 ( #22775, #30259 ),
 ( #3603, #18430 ),
 ( #6409, #1431 ),
 ( #3925, #18108 ),
 ( #27623, #25120 ),
 ( #16070, #3762 ),
 ( #1874, #15445 ) ),
 .UNSPECIFIED., .F., .F., .F.,
 ( 4, 3, 3, 3, 3, 3, 3, 3, 3, 3, 4 ),
 ( 2, 2 ),
 ( 0.000000000000000000, 0.05425176834609614362, 0.1085332949128348518, 0.1623767749169379715, 0.2157504826133058717, 0.2688657508888169789, 0.3218907763505471364, 0.3749548578363334772, 0.4282048033836237666, 0.4818374082110496448, 0.4999999999131654604 ),
 ( 0.000000000000000000, 1.000000000000000000 ),
 .UNSPECIFIED. ) ;
#1445=FACE_OUTER_BOUND ( 'NONE', #22621, .T. ) ;
#1457=EDGE_LOOP ( 'NONE', ( #8273, #15549, #9451, #27302 ) ) ;
#1459=CARTESIAN_POINT ( 'NONE',  ( -19.72672318758257148, 3.296256974645884075, 7.267242832833948007 ) ) ;
#1461=DIRECTION ( 'NONE',  ( -0.000000000000000000, -0.000000000000000000, 1.000000000000000000 ) ) ;
#1465=DIRECTION ( 'NONE',  ( 1.000000000000000000, 0.000000000000000000, 0.000000000000000000 ) ) ;
#1467=DIRECTION ( 'NONE',  ( -1.000000000000000000, 0.000000000000000000, 0.000000000000000000 ) ) ;
#1470=CARTESIAN_POINT ( 'NONE',  ( 1.082887659287353754, -19.98847979319445756, 5.951255046771932733 ) ) ;
#1476=CARTESIAN_POINT ( 'NONE',  ( 10.22519205257000863, -13.65449557370669176, 7.559636331181775581 ) ) ;
#1486=FACE_OUTER_BOUND ( 'NONE', #16197, .T. ) ;
#1487=EDGE_CURVE ( 'NONE', #29934, #18617, #5750, .T. ) ;
#1491=ADVANCED_FACE ( 'NONE', ( #27743 ), #18226, .T. ) ;
#1495=CARTESIAN_POINT ( 'NONE',  ( 19.58194293052861212, 4.068188588073703649, 18.84486140012300126 ) ) ;
#1498=CIRCLE ( 'NONE', #2484, 0.7500000000000011102 ) ;
#1502=CARTESIAN_POINT ( 'NONE',  ( 12.00027744594693324, 12.12900492880153891, 18.45571264222803975 ) ) ;
#1503=DIRECTION ( 'NONE',  ( 0.000000000000000000, 0.000000000000000000, -1.000000000000000000 ) ) ;
#1504=CARTESIAN_POINT ( 'NONE',  ( 0.8643805006890388221, -19.98168094404549322, 18.47531940416305929 ) ) ;
#1506=CARTESIAN_POINT ( 'NONE',  ( -16.99797872337272153, 1.390050218453713349, 7.652108011868849147 ) ) ;
#1520=CARTESIAN_POINT ( 'NONE',  ( 9.184330860358528525, -14.33603326865607741, 18.72771030977186868 ) ) ;
#1525=CARTESIAN_POINT ( 'NONE',  ( -11.25351117620539121, -16.53363456493219985, 18.84056766331481825 ) ) ;
#1527=CARTESIAN_POINT ( 'NONE',  ( 15.05691039802739084, 13.16451011206821242, 7.626647697317575414 ) ) ;
#1532=CARTESIAN_POINT ( 'NONE',  ( -14.93131746129344961, -8.256826158564470219, 5.759928666072747561 ) ) ;
#1538=CARTESIAN_POINT ( 'NONE',  ( 0.01267125088587631523, -20.01782649599895691, 7.595116371587256054 ) ) ;
#1539=CARTESIAN_POINT ( 'NONE',  ( -9.908187358984028137, -17.39367339311968053, 20.06253562465620632 ) ) ;
#1540=CARTESIAN_POINT ( 'NONE',  ( -17.02473723647801052, 1.129071356443817065, 20.24143955528809258 ) ) ;
#1541=CARTESIAN_POINT ( 'NONE',  ( -17.04940614979727798, 0.8516807413325224729, 18.73743063545763121 ) ) ;
#1546=ORIENTED_EDGE ( 'NONE', *, *, #14387, .F. ) ;
#1550=CARTESIAN_POINT ( 'NONE',  ( -15.34618562042307310, 12.82554431217321245, 5.652196082369965069 ) ) ;
#1552=CARTESIAN_POINT ( 'NONE',  ( -5.103338407348687156, 19.35644909001343450, 6.211014596808754007 ) ) ;
#1556=EDGE_CURVE ( 'NONE', #15672, #2241, #10408, .T. ) ;
#1557=CARTESIAN_POINT ( 'NONE',  ( -13.29701885124480576, 10.65950381936556113, 5.651492010659111997 ) ) ;
#1561=DIRECTION ( 'NONE',  ( -0.000000000000000000, -0.000000000000000000, -1.000000000000000000 ) ) ;
#1562=CARTESIAN_POINT ( 'NONE',  ( 2.094186647214742347, -9.248129367672074608, 1.500000000000001332 ) ) ;
#1564=VERTEX_POINT ( 'NONE', #23356 ) ;
#1567=EDGE_CURVE ( 'NONE', #23779, #9215, #4782, .T. ) ;
#1573=CARTESIAN_POINT ( 'NONE',  ( 3.215610563331066540, 16.76717343535964844, 7.196036389296800451 ) ) ;
#1576=CARTESIAN_POINT ( 'NONE',  ( 5.545588074468605022, 19.21617731956021302, 18.37250658438899009 ) ) ;
#1580=DIRECTION ( 'NONE',  ( 1.000000000000000000, 0.000000000000000000, 0.000000000000000000 ) ) ;
#1581=CARTESIAN_POINT ( 'NONE',  ( 19.89498243266959676, 2.215034284604904702, 19.11611934778430921 ) ) ;
#1583=CARTESIAN_POINT ( 'NONE',  ( -16.82187727961403922, 2.603938281378752162, 19.66989035740801839 ) ) ;
#1585=CARTESIAN_POINT ( 'NONE',  ( -14.01239083805804597, 9.763392886517387126, 6.560937769032974209 ) ) ;
#1586=CARTESIAN_POINT ( 'NONE',  ( 5.298969250677085796, 19.30368332842023094, 18.34798005862662507 ) ) ;
#1594=CARTESIAN_POINT ( 'NONE',  ( -5.023839636758346217, 19.37724795171757819, 19.11611934778430921 ) ) ;
#1595=FACE_OUTER_BOUND ( 'NONE', #5843, .T. ) ;
#1599=CARTESIAN_POINT ( 'NONE',  ( -5.846240454020377619, 19.12690956503888629, 7.652108011868849147 ) ) ;
#1600=VERTEX_POINT ( 'NONE', #6818 ) ;
#1603=CARTESIAN_POINT ( 'NONE',  ( -19.87001189204712759, 2.428856360474549447, 7.652108011868850035 ) ) ;
#1609=DIRECTION ( 'NONE',  ( -0.000000000000000000, -0.000000000000000000, -1.000000000000000000 ) ) ;
#1610=CARTESIAN_POINT ( 'NONE',  ( -19.85983307072122628, 2.367331911061644423, 20.34789198813115618 ) ) ;
#1612=CARTESIAN_POINT ( 'NONE',  ( 0.2238118478526182897, -19.99918941848005360, 5.651480102388688032 ) ) ;
#1613=CARTESIAN_POINT ( 'NONE',  ( -5.881244434206279514, -6.812559277181949646, 1.500000000000001332 ) ) ;
#1614=AXIS2_PLACEMENT_3D ( 'NONE', #4560, #28279, #9547 ) ;
#1617=LINE ( 'NONE', #20922, #5360 ) ;
#1618=LINE ( 'NONE', #23264, #22771 ) ;
#1619=CARTESIAN_POINT ( 'NONE',  ( 1.265447379378153769, -19.97763032565216079, 7.098451512883313441 ) ) ;
#1620=CARTESIAN_POINT ( 'NONE',  ( -16.87879800889955106, 2.262652451732489745, 5.848946451764560628 ) ) ;
#1622=EDGE_CURVE ( 'NONE', #10771, #1929, #26341, .T. ) ;
#1626=DIRECTION ( 'NONE',  ( -0.000000000000000000, -0.000000000000000000, 1.000000000000000000 ) ) ;
#1635=CARTESIAN_POINT ( 'NONE',  ( 0.000000000000000000, 0.000000000000000000, 21.50000000000000000 ) ) ;
#1637=VERTEX_POINT ( 'NONE', #16344 ) ;
#1640=CARTESIAN_POINT ( 'NONE',  ( -8.478038329015333829, 15.04174200911163517, -0.6213203435596476032 ) ) ;
#1642=DIRECTION ( 'NONE',  ( 1.000000000000000000, 0.000000000000000000, 0.000000000000000000 ) ) ;
#1643=CARTESIAN_POINT ( 'NONE',  ( 19.63396244889326425, 3.810028285208275634, 18.54958172136248606 ) ) ;
#1645=CARTESIAN_POINT ( 'NONE',  ( 17.75446986341059841, 9.207540381081344094, 24.50000000000000000 ) ) ;
#1648=CARTESIAN_POINT ( 'NONE',  ( 11.80522207443771521, 12.33118449403810146, 19.96568007040469084 ) ) ;
#1649=AXIS2_PLACEMENT_3D ( 'NONE', #27433, #3724, #22886 ) ;
#1650=CARTESIAN_POINT ( 'NONE',  ( 16.65271093596605922, 3.715728438117816168, 5.759928666072751113 ) ) ;
#1652=AXIS2_PLACEMENT_3D ( 'NONE', #29084, #17072, #7725 ) ;
#1656=CARTESIAN_POINT ( 'NONE',  ( 0.000000000000000000, 0.000000000000000000, 1.500000000000001332 ) ) ;
#1658=PLANE ( 'NONE',  #446 ) ;
#1659=CARTESIAN_POINT ( 'NONE',  ( -8.774062813931127636, -14.60569725955141962, 20.32222155561919053 ) ) ;
#1664=FACE_OUTER_BOUND ( 'NONE', #28593, .T. ) ;
#1666=CARTESIAN_POINT ( 'NONE',  ( -6.028330626922774549, 10.93629592680536788, 1.500000000000001332 ) ) ;
#1668=EDGE_LOOP ( 'NONE', ( #30066, #14694, #18967, #7612 ) ) ;
#1670=DIRECTION ( 'NONE',  ( 0.000000000000000000, 0.000000000000000000, 1.000000000000000000 ) ) ;
#1671=B_SPLINE_CURVE_WITH_KNOTS ( 'NONE', 3,
 ( #9802, #19468, #7618, #11837, #2626, #7157, #23979, #21647, #19014, #19160, #17281, #14316, #21487, #9496, #28526, #21806, #28983, #17123, #28679, #24301 ),
 .UNSPECIFIED., .F., .F.,
 ( 4, 2, 2, 2, 2, 2, 2, 2, 2, 4 ),
 ( 0.000000000000000000, 0.06250000000000160982, 0.1250000000000035527, 0.1875000000000054956, 0.2187500000000055789, 0.2500000000000056621, 0.3125000000000041633, 0.3750000000000026645, 0.4375000000000011657, 0.5000000000000000000 ),
 .UNSPECIFIED. ) ;
#1672=CARTESIAN_POINT ( 'NONE',  ( -10.71492722147446308, -16.90904491356049633, 18.36582235739946611 ) ) ;
#1674=EDGE_LOOP ( 'NONE', ( #10641, #9379, #25960, #27802 ) ) ;
#1676=ORIENTED_EDGE ( 'NONE', *, *, #17163, .T. ) ;
#1677=DIRECTION ( 'NONE',  ( 0.000000000000000000, 0.000000000000000000, 1.000000000000000000 ) ) ;
#1678=ORIENTED_EDGE ( 'NONE', *, *, #16623, .T. ) ;
#1685=CARTESIAN_POINT ( 'NONE',  ( -17.05973338880502155, 0.7261025713186424202, 18.92976555901915603 ) ) ;
#1686=FACE_BOUND ( 'NONE', #30371, .T. ) ;
#1687=ORIENTED_EDGE ( 'NONE', *, *, #3333, .T. ) ;
#1689=B_SPLINE_CURVE_WITH_KNOTS ( 'NONE', 3,
 ( #23857, #12017, #9671, #7339, #16849, #26363, #7964, #9827, #14963, #470, #29322, #7642, #22287, #26515, #21981, #29006, #10129, #19634 ),
 .UNSPECIFIED., .F., .F.,
 ( 4, 2, 2, 2, 2, 2, 2, 2, 4 ),
 ( 0.000000000000000000, 0.0003967869494442956908, 0.0007935738988885913817, 0.001190360848332887127, 0.001587147797777182763, 0.001983934747221478400, 0.002380721696665774254, 0.002777508646110069673, 0.003174295595554365527 ),
 .UNSPECIFIED. ) ;
#1691=DIRECTION ( 'NONE',  ( 0.9594929736144952592, -0.2817325568414371095, 0.000000000000000000 ) ) ;
#1693=ORIENTED_EDGE ( 'NONE', *, *, #24644, .F. ) ;
#1695=CARTESIAN_POINT ( 'NONE',  ( -4.940218127011007709, 16.29708528951389113, 5.862424720655265098 ) ) ;
#1701=DIRECTION ( 'NONE',  ( -1.000000000000000000, 0.000000000000000000, 0.000000000000000000 ) ) ;
#1710=EDGE_CURVE ( 'NONE', #17660, #12655, #26844, .T. ) ;
#1711=CARTESIAN_POINT ( 'NONE',  ( -15.57772019539775776, -6.859948791675931190, 6.755862304746362845 ) ) ;
#1713=DIRECTION ( 'NONE',  ( -1.000000000000000000, 0.000000000000000000, 0.000000000000000000 ) ) ;
#1715=VERTEX_POINT ( 'NONE', #4492 ) ;
#1721=CARTESIAN_POINT ( 'NONE',  ( -16.96496223448354712, 1.652369715233090286, 20.34789198813115263 ) ) ;
#1722=CARTESIAN_POINT ( 'NONE',  ( 15.39622458953738082, -7.259188434806188361, 6.864725433338323413 ) ) ;
#1724=CARTESIAN_POINT ( 'NONE',  ( 4.316117848019421999, 19.54676362458759087, 19.36813350477385143 ) ) ;
#1730=CARTESIAN_POINT ( 'NONE',  ( -4.673829994069182980, 16.36915245889225545, 18.90679857307105749 ) ) ;
#1731=DIRECTION ( 'NONE',  ( 1.000000000000000000, 0.000000000000000000, 0.000000000000000000 ) ) ;
#1732=CARTESIAN_POINT ( 'NONE',  ( 11.80353037517518366, 12.33292095755542483, 6.037360021877313798 ) ) ;
#1737=ORIENTED_EDGE ( 'NONE', *, *, #20599, .T. ) ;
#1738=CARTESIAN_POINT ( 'NONE',  ( 0.6218383925729503714, -19.99069893758407446, 5.679672709359372185 ) ) ;
#1739=CARTESIAN_POINT ( 'NONE',  ( 14.79007711409980175, 13.46370387462956586, 18.34869673959212122 ) ) ;
#1745=UNCERTAINTY_MEASURE_WITH_UNIT (LENGTH_MEASURE( 1.000000000000000082E-05 ), #891, 'distance_accuracy_value', 'NONE');
#1748=CARTESIAN_POINT ( 'NONE',  ( 0.000000000000000000, 0.000000000000000000, 21.50000000000000000 ) ) ;
#1749=VECTOR ( 'NONE', #19643, 1000.000000000000000 ) ;
#1758=CARTESIAN_POINT ( 'NONE',  ( 1.411528516173250924, -17.00651183856732374, 7.441806358946449151 ) ) ;
#1760=VERTEX_POINT ( 'NONE', #7755 ) ;
#1768=CARTESIAN_POINT ( 'NONE',  ( -14.83655028254229258, -8.438271213925730763, 18.64703902303423178 ) ) ;
#1769=ADVANCED_FACE ( 'NONE', ( #26470 ), #29276, .F. ) ;
#1772=DIRECTION ( 'NONE',  ( 1.000000000000000000, 0.000000000000000000, 0.000000000000000000 ) ) ;
#1774=CARTESIAN_POINT ( 'NONE',  ( -12.72536390617885260, -2.839914339433650348, 1.500000000000001332 ) ) ;
#1783=EDGE_CURVE ( 'NONE', #27228, #19294, #6425, .T. ) ;
#1791=DIRECTION ( 'NONE',  ( 1.000000000000000000, 0.000000000000000000, 0.000000000000000000 ) ) ;
#1792=DIRECTION ( 'NONE',  ( 1.000000000000000000, 0.000000000000000000, 0.000000000000000000 ) ) ;
#1793=ORIENTED_EDGE ( 'NONE', *, *, #14566, .T. ) ;
#1794=EDGE_CURVE ( 'NONE', #13443, #12232, #13404, .T. ) ;
#1797=CARTESIAN_POINT ( 'NONE',  ( 16.56110944985980282, 4.167213836802830862, 6.917457548096560771 ) ) ;
#1798=EDGE_CURVE ( 'NONE', #23467, #17274, #12906, .T. ) ;
#1801=AXIS2_PLACEMENT_3D ( 'NONE', #26371, #16999, #2977 ) ;
#1803=CYLINDRICAL_SURFACE ( 'NONE', #7872, 9.482273699623480212 ) ;
#1805=CARTESIAN_POINT ( 'NONE',  ( 3.264443110924797331, 16.75603743217150310, 19.96568007040468373 ) ) ;
#1814=CARTESIAN_POINT ( 'NONE',  ( -7.717362503659074058, -15.23305454438620110, 6.329955581934034292 ) ) ;
#1816=AXIS2_PLACEMENT_3D ( 'NONE', #15642, #22653, #25154 ) ;
#1819=CARTESIAN_POINT ( 'NONE',  ( 15.38930515692758405, -7.273136567754734827, 19.22654678686458141 ) ) ;
#1820=CARTESIAN_POINT ( 'NONE',  ( 9.181265711014134467, -14.33790826712539079, 19.96344307082652492 ) ) ;
#1822=ADVANCED_FACE ( 'NONE', ( #6024 ), #8376, .F. ) ;
#1824=CARTESIAN_POINT ( 'NONE',  ( -19.83214989528428163, 2.722369515932092643, 5.670038381137163519 ) ) ;
#1826=CIRCLE ( 'NONE', #1312, 0.7499999999999997780 ) ;
#1829=ORIENTED_EDGE ( 'NONE', *, *, #16466, .T. ) ;
#1835=CARTESIAN_POINT ( 'NONE',  ( 19.74328841314636307, 3.194145055459935101, 7.652108011868850035 ) ) ;
#1842=CARTESIAN_POINT ( 'NONE',  ( -7.028330626922778990, 10.93629592680536788, 1.500000000000001332 ) ) ;
#1843=DIRECTION ( 'NONE',  ( 1.000000000000000000, 0.000000000000000000, 0.000000000000000000 ) ) ;
#1844=DIRECTION ( 'NONE',  ( 0.000000000000000000, 0.000000000000000000, 1.000000000000000000 ) ) ;
#1850=ORIENTED_EDGE ( 'NONE', *, *, #14891, .F. ) ;
#1852=CARTESIAN_POINT ( 'NONE',  ( -7.856594496258223259, -4.390207617113929039, 21.50000000000000000 ) ) ;
#1853=VERTEX_POINT ( 'NONE', #25363 ) ;
#1855=CARTESIAN_POINT ( 'NONE',  ( 15.75094665830062723, -12.32508334119354032, 24.50000000000000000 ) ) ;
#1866=ORIENTED_EDGE ( 'NONE', *, *, #5959, .F. ) ;
#1872=AXIS2_PLACEMENT_3D ( 'NONE', #24898, #18348, #27700 ) ;
#1874=CARTESIAN_POINT ( 'NONE',  ( 11.11866449908641208, -16.64592002940951687, 18.34798005862930736 ) ) ;
#1875=CARTESIAN_POINT ( 'NONE',  ( 19.76052160831509852, 3.198927888535952668, 18.34798005862930736 ) ) ;
#1877=CARTESIAN_POINT ( 'NONE',  ( -19.70840172719294969, 3.506524300503917502, 19.33715507985239412 ) ) ;
#1878=CARTESIAN_POINT ( 'NONE',  ( 15.67696945782692453, -6.669264855739881703, 5.701226463332907279 ) ) ;
#1880=CARTESIAN_POINT ( 'NONE',  ( -14.00200865723716781, 9.777219707070196719, 6.447548852708279377 ) ) ;
#1881=CARTESIAN_POINT ( 'NONE',  ( 3.338654329031695678, 16.73860904129763938, 18.64703902303423178 ) ) ;
#1882=VERTEX_POINT ( 'NONE', #22858 ) ;
#1883=ORIENTED_EDGE ( 'NONE', *, *, #17006, .T. ) ;
#1886=CARTESIAN_POINT ( 'NONE',  ( 10.52561254559630655, -13.43997246249538513, 7.269896094239229001 ) ) ;
#1887=CARTESIAN_POINT ( 'NONE',  ( 12.93287820108835007, 11.07039438038045454, 7.156916968540299351 ) ) ;
#1893=CARTESIAN_POINT ( 'NONE',  ( -17.06158983937615403, 0.7019473037495110868, 6.995624166085161910 ) ) ;
#1894=CARTESIAN_POINT ( 'NONE',  ( 14.18379620663259644, 14.10035196125401846, 19.48477075383298285 ) ) ;
#1899=CARTESIAN_POINT ( 'NONE',  ( 15.90320373664001075, -6.152843468454366693, 5.678370764302467677 ) ) ;
#1900=ADVANCED_FACE ( 'NONE', ( #10701 ), #18192, .F. ) ;
#1901=AXIS2_PLACEMENT_3D ( 'NONE', #16865, #26382, #29171 ) ;
#1904=DIRECTION ( 'NONE',  ( -1.000000000000000000, 0.000000000000000000, 0.000000000000000000 ) ) ;
#1905=LINE ( 'NONE', #18458, #3825 ) ;
#1906=FACE_OUTER_BOUND ( 'NONE', #6700, .T. ) ;
#1913=CIRCLE ( 'NONE', #915, 20.00000000000000000 ) ;
#1918=CARTESIAN_POINT ( 'NONE',  ( -17.62281152098609738, -9.494300025206934279, 19.03762469184452755 ) ) ;
#1919=DIRECTION ( 'NONE',  ( 0.000000000000000000, 0.000000000000000000, 1.000000000000000000 ) ) ;
#1923=DIRECTION ( 'NONE',  ( 0.000000000000000000, 0.000000000000000000, 1.000000000000000000 ) ) ;
#1924=LINE ( 'NONE', #1774, #18634 ) ;
#1929=VERTEX_POINT ( 'NONE', #15682 ) ;
#1930=EDGE_CURVE ( 'NONE', #5916, #2507, #1347, .T. ) ;
#1931=DIRECTION ( 'NONE',  ( 1.000000000000000000, 0.000000000000000000, -0.000000000000000000 ) ) ;
#1935=ORIENTED_EDGE ( 'NONE', *, *, #16710, .F. ) ;
#1937=B_SPLINE_SURFACE_WITH_KNOTS ( 'NONE', 3, 1, ( 
 ( #25467, #21206 ),
 ( #4234, #9079 ),
 ( #6729, #4540 ),
 ( #25759, #1899 ),
 ( #11261, #20757 ),
 ( #14197, #14048 ),
 ( #20915, #21379 ),
 ( #6586, #16099 ),
 ( #30438, #16240 ),
 ( #11568, #21060 ),
 ( #9224, #18740 ),
 ( #28253, #14821 ),
 ( #26380, #316 ),
 ( #773, #21844 ),
 ( #10144, #26851 ),
 ( #19356, #5310 ),
 ( #19811, #5474 ),
 ( #2518, #14975 ),
 ( #12181, #161 ),
 ( #10296, #19191 ),
 ( #9840, #29170 ),
 ( #9681, #7191 ),
 ( #16702, #24336 ),
 ( #5155, #24488 ),
 ( #3133, #625 ),
 ( #28877, #10001 ),
 ( #21995, #19649 ),
 ( #12656, #16864 ),
 ( #17007, #26529 ),
 ( #7509, #2983 ),
 ( #26211, #28715 ) ),
 .UNSPECIFIED., .F., .F., .F.,
 ( 4, 3, 3, 3, 3, 3, 3, 3, 3, 3, 4 ),
 ( 2, 2 ),
 ( 0.4999999998345681651, 0.5360336730431942698, 0.5907651151589017324, 0.6456034593241839481, 0.6998270958050443191, 0.7529536536315944995, 0.8052385063053264513, 0.8575343587103996246, 0.9106564858195047574, 0.9648414833209688624, 1.000000006602610014 ),
 ( 0.000000000000000000, 1.000000000000000000 ),
 .UNSPECIFIED. ) ;
#1942=B_SPLINE_CURVE_WITH_KNOTS ( 'NONE', 3,
 ( #9420, #2073, #9257, #28295, #25496, #27983, #18623, #28443, #11297, #6920, #21409, #16430, #2228, #15977, #25945, #6614 ),
 .UNSPECIFIED., .F., .F.,
 ( 4, 2, 2, 2, 2, 2, 2, 4 ),
 ( 0.5000000000000000000, 0.6250000000000004441, 0.6875000000000008882, 0.7187500000000008882, 0.7500000000000008882, 0.8125000000000006661, 0.8750000000000002220, 1.000000000000000000 ),
 .UNSPECIFIED. ) ;
#1955=VECTOR ( 'NONE', #22976, 1000.000000000000000 ) ;
#1957=DIRECTION ( 'NONE',  ( 0.4154150130018864906, -0.9096319953545183301, 0.000000000000000000 ) ) ;
#1959=FACE_OUTER_BOUND ( 'NONE', #10569, .T. ) ;
#1967=EDGE_CURVE ( 'NONE', #23890, #24237, #17649, .T. ) ;
#1971=CARTESIAN_POINT ( 'NONE',  ( 15.55167013926946140, -6.938753487154069255, 18.55820869691756769 ) ) ;
#1973=CARTESIAN_POINT ( 'NONE',  ( 4.575061044035273028, 16.40537387836875993, 7.500898271101006820 ) ) ;
#1974=VERTEX_POINT ( 'NONE', #23609 ) ;
#1975=CARTESIAN_POINT ( 'NONE',  ( -11.19315777850258620, -16.57474394094692371, 19.96302680909623462 ) ) ;
#1977=CARTESIAN_POINT ( 'NONE',  ( 11.80864398233535795, 12.32734916534602654, 6.041646659195333058 ) ) ;
#1978=VECTOR ( 'NONE', #13755, 1000.000000000000114 ) ;
#1979=CARTESIAN_POINT ( 'NONE',  ( 9.590471615930072247, -1.687027447297460236, 1.500000000000001332 ) ) ;
#1981=ORIENTED_EDGE ( 'NONE', *, *, #21356, .F. ) ;
#1985=CARTESIAN_POINT ( 'NONE',  ( -14.81308450742032967, 13.43805957489523095, 7.267242832833945343 ) ) ;
#1987=CARTESIAN_POINT ( 'NONE',  ( 16.81826667486039639, 2.692788315295377988, 20.22273502201483453 ) ) ;
#1991=AXIS2_PLACEMENT_3D ( 'NONE', #27841, #25338, #23290 ) ;
#1994=CARTESIAN_POINT ( 'NONE',  ( -19.86072491926578110, 2.502642356747510899, 20.34789198813115263 ) ) ;
#1995=DIRECTION ( 'NONE',  ( 1.000000000000000000, 0.000000000000000000, 0.000000000000000000 ) ) ;
#2000=VECTOR ( 'NONE', #21282, 1000.000000000000000 ) ;
#2001=CARTESIAN_POINT ( 'NONE',  ( -5.549075634136967139, 16.11684027513961226, 5.652196082368482699 ) ) ;
#2005=CARTESIAN_POINT ( 'NONE',  ( -15.96020336975123577, 12.05298949301765887, 6.392525840300344875 ) ) ;
#2008=VERTEX_POINT ( 'NONE', #4457 ) ;
#2010=CARTESIAN_POINT ( 'NONE',  ( -15.43151021478632501, 12.72345061513107112, 18.34869673959212477 ) ) ;
#2011=AXIS2_PLACEMENT_3D ( 'NONE', #26375, #24332, #9996 ) ;
#2018=CARTESIAN_POINT ( 'NONE',  ( -0.1027882698221962710, -17.02358378464945687, 19.85270094495842130 ) ) ;
#2019=CARTESIAN_POINT ( 'NONE',  ( -5.352643706120520761, -7.827050521741861999, 13.00000000000000178 ) ) ;
#2021=CARTESIAN_POINT ( 'NONE',  ( -9.185733585337898077, 2.352830851074200869, 1.500000000000001332 ) ) ;
#2023=CARTESIAN_POINT ( 'NONE',  ( -16.93638505691475160, 1.872096242067391225, 18.36582235739946611 ) ) ;
#2027=CARTESIAN_POINT ( 'NONE',  ( -13.47895127716181207, 10.44112259311556379, 5.661398277488802755 ) ) ;
#2028=CARTESIAN_POINT ( 'NONE',  ( 3.085425824774455261, 16.79642356368104927, 19.58863275299554019 ) ) ;
#2029=ORIENTED_EDGE ( 'NONE', *, *, #8765, .F. ) ;
#2034=CARTESIAN_POINT ( 'NONE',  ( -5.292761969338718231, 19.30549167878804440, 18.63641924841378028 ) ) ;
#2038=VERTEX_POINT ( 'NONE', #30190 ) ;
#2039=CARTESIAN_POINT ( 'NONE',  ( -19.96032475228488323, 1.513912977174407981, 6.892848776733236704 ) ) ;
#2040=DIRECTION ( 'NONE',  ( 1.000000000000000000, 0.000000000000000000, 0.000000000000000000 ) ) ;
#2041=CARTESIAN_POINT ( 'NONE',  ( 3.668292057955996555, -8.743977807160087323, 1.500000000000001332 ) ) ;
#2045=FACE_OUTER_BOUND ( 'NONE', #13773, .T. ) ;
#2048=ORIENTED_EDGE ( 'NONE', *, *, #29042, .T. ) ;
#2053=CARTESIAN_POINT ( 'NONE',  ( -6.878634932266925794, 18.79866186728735400, 19.69140814234746273 ) ) ;
#2057=AXIS2_PLACEMENT_3D ( 'NONE', #1842, #13702, #11200 ) ;
#2058=CARTESIAN_POINT ( 'NONE',  ( 15.47699552843811155, -7.094814489843902727, 6.031926333436656407 ) ) ;
#2059=DIRECTION ( 'NONE',  ( 1.000000000000000000, 0.000000000000000000, 0.000000000000000000 ) ) ;
#2063=CARTESIAN_POINT ( 'NONE',  ( 11.29839223038184670, -16.52442514205455026, 7.627891251804737927 ) ) ;
#2064=CARTESIAN_POINT ( 'NONE',  ( 9.999999999999959144, 1.510243460696181139E-14, 21.50000000000000000 ) ) ;
#2066=CARTESIAN_POINT ( 'NONE',  ( 0.000000000000000000, 0.000000000000000000, 1.500000000000001332 ) ) ;
#2067=ORIENTED_EDGE ( 'NONE', *, *, #17202, .T. ) ;
#2069=DIRECTION ( 'NONE',  ( -0.000000000000000000, -0.000000000000000000, 1.000000000000000000 ) ) ;
#2071=DIRECTION ( 'NONE',  ( -1.000000000000000000, 0.000000000000000000, 0.000000000000000000 ) ) ;
#2072=VERTEX_POINT ( 'NONE', #8828 ) ;
#2073=CARTESIAN_POINT ( 'NONE',  ( -13.55077504496076557, 10.35587614721247718, 5.653604225791663218 ) ) ;
#2077=ORIENTED_EDGE ( 'NONE', *, *, #24044, .F. ) ;
#2078=ORIENTED_EDGE ( 'NONE', *, *, #10320, .F. ) ;
#2083=CARTESIAN_POINT ( 'NONE',  ( -7.669844488642331370, -15.25924058316908827, 6.560937769032974209 ) ) ;
#2086=CARTESIAN_POINT ( 'NONE',  ( 1.694955473231259058, -16.99033591619068773, 19.79423548914561692 ) ) ;
#2087=ORIENTED_EDGE ( 'NONE', *, *, #20649, .F. ) ;
#2091=DIRECTION ( 'NONE',  ( -1.000000000000000000, 0.000000000000000000, 0.000000000000000000 ) ) ;
#2092=VERTEX_POINT ( 'NONE', #18350 ) ;
#2097=CARTESIAN_POINT ( 'NONE',  ( -15.16517293421788537, -7.781889191988407006, 20.34789198813115263 ) ) ;
#2104=CARTESIAN_POINT ( 'NONE',  ( 9.169883732660084164, -9.268939115642975679, 1.500000000000001332 ) ) ;
#2106=VERTEX_POINT ( 'NONE', #966 ) ;
#2112=EDGE_LOOP ( 'NONE', ( #6991, #27206 ) ) ;
#2114=CARTESIAN_POINT ( 'NONE',  ( 15.45190528822775633, -7.145941350103554690, 19.87181966307587544 ) ) ;
#2115=EDGE_CURVE ( 'NONE', #12148, #22258, #12417, .T. ) ;
#2116=CARTESIAN_POINT ( 'NONE',  ( 5.524396280439209939, 19.24072699314231727, 7.632642797338977658 ) ) ;
#2119=CARTESIAN_POINT ( 'NONE',  ( 4.994189150946232836, 16.27260345083323756, 19.56050940960062690 ) ) ;
#2136=CARTESIAN_POINT ( 'NONE',  ( 0.2355109517537151975, -20.01673911375432624, 7.652108011868850035 ) ) ;
#2137=EDGE_CURVE ( 'NONE', #22258, #26398, #30829, .T. ) ;
#2141=CARTESIAN_POINT ( 'NONE',  ( -17.01545599012840526, 1.214108451629964058, 20.25542030744407640 ) ) ;
#2143=ORIENTED_EDGE ( 'NONE', *, *, #25575, .T. ) ;
#2144=EDGE_CURVE ( 'NONE', #30466, #1099, #21366, .T. ) ;
#2145=FACE_OUTER_BOUND ( 'NONE', #28041, .T. ) ;
#2151=CARTESIAN_POINT ( 'NONE',  ( 5.163176754322200246, 19.32250783072323586, 18.34869673959212122 ) ) ;
#2154=VERTEX_POINT ( 'NONE', #5221 ) ;
#2155=FACE_OUTER_BOUND ( 'NONE', #1137, .T. ) ;
#2160=ORIENTED_EDGE ( 'NONE', *, *, #16829, .T. ) ;
#2165=EDGE_CURVE ( 'NONE', #28271, #28669, #8297, .T. ) ;
#2168=ORIENTED_EDGE ( 'NONE', *, *, #26325, .T. ) ;
#2169=CIRCLE ( 'NONE', #23573, 1.000000000000008438 ) ;
#2173=CARTESIAN_POINT ( 'NONE',  ( 0.5152247664106277547, -17.03071091119081615, 20.32222155561919053 ) ) ;
#2177=ORIENTED_EDGE ( 'NONE', *, *, #2506, .T. ) ;
#2178=CARTESIAN_POINT ( 'NONE',  ( 9.669732009941352402, -14.02977311367123647, 7.632642797338977658 ) ) ;
#2180=CARTESIAN_POINT ( 'NONE',  ( 8.413215745754998309, -3.196529495465417980, 21.50000000000000000 ) ) ;
#2181=ORIENTED_EDGE ( 'NONE', *, *, #17821, .F. ) ;
#2182=ORIENTED_EDGE ( 'NONE', *, *, #12436, .F. ) ;
#2183=CARTESIAN_POINT ( 'NONE',  ( 18.33792385446292883, -7.982495159855863776, 18.34798005863227388 ) ) ;
#2185=CARTESIAN_POINT ( 'NONE',  ( 15.21635490854753847, 12.97988522761634655, 20.22277707861861984 ) ) ;
#2186=CARTESIAN_POINT ( 'NONE',  ( -5.460567910819448478, 19.25894470870317932, 18.49267272388512140 ) ) ;
#2188=DIRECTION ( 'NONE',  ( 0.000000000000000000, 0.000000000000000000, 1.000000000000000000 ) ) ;
#2191=CARTESIAN_POINT ( 'NONE',  ( -5.124412594240641106, 19.33243322302223532, 7.156831654632821227 ) ) ;
#2193=CARTESIAN_POINT ( 'NONE',  ( -17.04815991962220068, 0.8662532504481914586, 7.280727868105637768 ) ) ;
#2194=DIRECTION ( 'NONE',  ( 1.000000000000000000, 0.000000000000000000, 0.000000000000000000 ) ) ;
#2199=EDGE_CURVE ( 'NONE', #28757, #3557, #22108, .T. ) ;
#2200=FACE_OUTER_BOUND ( 'NONE', #9290, .T. ) ;
#2201=DIRECTION ( 'NONE',  ( -0.000000000000000000, -0.000000000000000000, 1.000000000000000000 ) ) ;
#2202=EDGE_LOOP ( 'NONE', ( #4000, #3710 ) ) ;
#2205=CARTESIAN_POINT ( 'NONE',  ( -16.96496224101209194, 1.652369717150044659, 7.652108011868850923 ) ) ;
#2207=CARTESIAN_POINT ( 'NONE',  ( -5.870757325077153865, 16.01346137069357312, 18.39992786714538298 ) ) ;
#2209=DIRECTION ( 'NONE',  ( 0.000000000000000000, 0.000000000000000000, 1.000000000000000000 ) ) ;
#2211=CARTESIAN_POINT ( 'NONE',  ( 0.000000000000000000, 0.000000000000000000, 1.500000000000001332 ) ) ;
#2213=CARTESIAN_POINT ( 'NONE',  ( 5.291489565152559749, 19.28730510418394672, 18.34798005863226678 ) ) ;
#2216=ORIENTED_EDGE ( 'NONE', *, *, #26162, .F. ) ;
#2218=CARTESIAN_POINT ( 'NONE',  ( -17.77905984561984454, -9.199004478715989919, 20.13759033520874908 ) ) ;
#2219=DIRECTION ( 'NONE',  ( 1.000000000000000000, 0.000000000000000000, 0.000000000000000000 ) ) ;
#2223=CARTESIAN_POINT ( 'NONE',  ( 0.3518703668723784928, -19.99690444156084723, 20.34789198813115263 ) ) ;
#2226=FACE_BOUND ( 'NONE', #16094, .T. ) ;
#2228=CARTESIAN_POINT ( 'NONE',  ( -13.88572908622542812, 9.930151408543668623, 7.269896094239229889 ) ) ;
#2230=CYLINDRICAL_SURFACE ( 'NONE', #24903, 20.00000000000000000 ) ;
#2232=CIRCLE ( 'NONE', #25147, 1.000000000000011324 ) ;
#2237=CARTESIAN_POINT ( 'NONE',  ( -0.5073662589470785411, -20.01152162034081528, 18.80699882434806369 ) ) ;
#2238=CARTESIAN_POINT ( 'NONE',  ( -10.14924625765043587, -17.25430667454971356, 7.559636331181775581 ) ) ;
#2240=CARTESIAN_POINT ( 'NONE',  ( 0.5800982118606496929, -20.00934090639730201, 18.37415474056476938 ) ) ;
#2241=VERTEX_POINT ( 'NONE', #17140 ) ;
#2244=CARTESIAN_POINT ( 'NONE',  ( 0.9714284548196561175, -19.97661650614234929, 20.15039051365863543 ) ) ;
#2246=ORIENTED_EDGE ( 'NONE', *, *, #18754, .T. ) ;
#2247=DIRECTION ( 'NONE',  ( 0.6548607339452782172, -0.7557495743542642641, 0.000000000000000000 ) ) ;
#2248=CARTESIAN_POINT ( 'NONE',  ( -13.04869608149710558, 10.94699654838865222, 20.22273502201483453 ) ) ;
#2252=CARTESIAN_POINT ( 'NONE',  ( -18.04365185506139113, -8.627086862512678422, 20.34789198813115263 ) ) ;
#2253=CARTESIAN_POINT ( 'NONE',  ( -18.20359163036460615, -8.327231829331820379, 20.29090034784956131 ) ) ;
#2256=VERTEX_POINT ( 'NONE', #20520 ) ;
#2260=CARTESIAN_POINT ( 'NONE',  ( 11.83211694375101253, -16.12463123479446381, 19.85730954408919757 ) ) ;
#2263=CARTESIAN_POINT ( 'NONE',  ( 18.08817148584474310, -8.575141465928741269, 20.12545155307891065 ) ) ;
#2265=CARTESIAN_POINT ( 'NONE',  ( 6.127899591227619069, 19.05688428395638923, 7.176035686813569292 ) ) ;
#2266=EDGE_CURVE ( 'NONE', #580, #21713, #19371, .T. ) ;
#2268=CARTESIAN_POINT ( 'NONE',  ( 0.000000000000000000, 0.000000000000000000, 1.500000000000001332 ) ) ;
#2269=CARTESIAN_POINT ( 'NONE',  ( 5.687793815610356241, -6.974883619896809606, 1.500000000000001332 ) ) ;
#2273=CARTESIAN_POINT ( 'NONE',  ( 9.169883732660084164, -9.268939115642975679, 1.500000000000001332 ) ) ;
#2274=AXIS2_PLACEMENT_3D ( 'NONE', #940, #5771, #25682 ) ;
#2276=LINE ( 'NONE', #7270, #18049 ) ;
#2277=AXIS2_PLACEMENT_3D ( 'NONE', #21988, #27456, #22297 ) ;
#2279=ORIENTED_EDGE ( 'NONE', *, *, #15617, .F. ) ;
#2280=CARTESIAN_POINT ( 'NONE',  ( -18.20359163036459194, -8.327231829331816826, 7.595116371587256054 ) ) ;
#2281=CARTESIAN_POINT ( 'NONE',  ( -6.187077094091591789, 11.47693674426096955, 24.50000000000000000 ) ) ;
#2284=CARTESIAN_POINT ( 'NONE',  ( -9.958038337755704461, 17.34466697471556884, 1.500000000000001332 ) ) ;
#2285=EDGE_CURVE ( 'NONE', #15211, #1760, #19789, .T. ) ;
#2286=LINE ( 'NONE', #18678, #87 ) ;
#2287=CARTESIAN_POINT ( 'NONE',  ( -17.05861610865857259, 0.7402736376837835142, 19.79423548914561692 ) ) ;
#2289=ORIENTED_EDGE ( 'NONE', *, *, #8671, .F. ) ;
#2290=CARTESIAN_POINT ( 'NONE',  ( 10.69045173577873697, -13.31838649416133080, 19.47783254395485031 ) ) ;
#2293=EDGE_LOOP ( 'NONE', ( #27478, #25017 ) ) ;
#2296=CIRCLE ( 'NONE', #18331, 1.000000000000007772 ) ;
#2300=CARTESIAN_POINT ( 'NONE',  ( 15.04974025769138990, 13.19961543621590749, 20.32842677360128292 ) ) ;
#2304=EDGE_CURVE ( 'NONE', #4693, #15666, #15040, .T. ) ;
#2306=CARTESIAN_POINT ( 'NONE',  ( -15.96020336975123577, 12.05298949301765177, 19.08830981656265635 ) ) ;
#2314=ADVANCED_FACE ( 'NONE', ( #28155 ), #1658, .F. ) ;
#2315=CIRCLE ( 'NONE', #19756, 9.482273699623480212 ) ;
#2319=CARTESIAN_POINT ( 'NONE',  ( 1.497940275966470614, -17.00196529467652340, 7.366751648393900176 ) ) ;
#2322=DIRECTION ( 'NONE',  ( 1.000000000000000000, 0.000000000000000000, 0.000000000000000000 ) ) ;
#2323=CARTESIAN_POINT ( 'NONE',  ( 19.84003625978226637, 2.664153601443035146, 18.49267272388512140 ) ) ;
#2325=CARTESIAN_POINT ( 'NONE',  ( 9.489008252200360261, -14.14611184196831495, 7.557577766377196582 ) ) ;
#2334=CARTESIAN_POINT ( 'NONE',  ( 9.755064781586030520, 13.32952022457704544, -0.6213203435596476032 ) ) ;
#2338=CIRCLE ( 'NONE', #13823, 9.482273699623480212 ) ;
#2339=ADVANCED_FACE ( 'NONE', ( #4289 ), #25973, .F. ) ;
#2340=CARTESIAN_POINT ( 'NONE',  ( -5.026174198947135352, 19.35820631361449884, 6.913388067999415298 ) ) ;
#2342=ADVANCED_FACE ( 'NONE', ( #18805 ), #23083, .T. ) ;
#2343=CIRCLE ( 'NONE', #12833, 9.482273699623480212 ) ;
#2344=DIRECTION ( 'NONE',  ( 1.000000000000000000, 0.000000000000000000, 0.000000000000000000 ) ) ;
#2348=ORIENTED_EDGE ( 'NONE', *, *, #30410, .T. ) ;
#2356=VECTOR ( 'NONE', #14992, 1000.000000000000114 ) ;
#2362=CARTESIAN_POINT ( 'NONE',  ( 10.68714603011733288, -13.32085008214098210, 19.21769074125273491 ) ) ;
#2368=DIRECTION ( 'NONE',  ( -0.5406408174555976665, 0.8412535328311812055, 0.000000000000000000 ) ) ;
#2376=AXIS2_PLACEMENT_3D ( 'NONE', #26555, #24830, #5183 ) ;
#2379=LINE ( 'NONE', #26705, #18270 ) ;
#2380=VECTOR ( 'NONE', #13548, 1000.000000000000000 ) ;
#2383=CIRCLE ( 'NONE', #10361, 0.7500000000000024425 ) ;
#2388=CARTESIAN_POINT ( 'NONE',  ( -6.560142022084716196, 18.89374015187017264, 7.454606537396340826 ) ) ;
#2392=VERTEX_POINT ( 'NONE', #382 ) ;
#2394=DIRECTION ( 'NONE',  ( -0.000000000000000000, -0.000000000000000000, 1.000000000000000000 ) ) ;
#2395=AXIS2_PLACEMENT_3D ( 'NONE', #18603, #30445, #25477 ) ;
#2397=VERTEX_POINT ( 'NONE', #9900 ) ;
#2400=ORIENTED_EDGE ( 'NONE', *, *, #26325, .F. ) ;
#2401=CARTESIAN_POINT ( 'NONE',  ( -0.4512825100096619080, -20.01288639008904369, 19.96783386855779341 ) ) ;
#2403=CARTESIAN_POINT ( 'NONE',  ( -7.715867830805696492, -15.23386229593461216, 6.341840715582230281 ) ) ;
#2406=CARTESIAN_POINT ( 'NONE',  ( 1.121436987360517445, -17.01878714021719929, 18.39992786714538298 ) ) ;
#2408=EDGE_LOOP ( 'NONE', ( #16575, #6312, #23919, #7160 ) ) ;
#2409=CARTESIAN_POINT ( 'NONE',  ( 18.38841581631819366, -7.866599884335185422, 7.652108011868850923 ) ) ;
#2411=CARTESIAN_POINT ( 'NONE',  ( 11.85823002435686035, 12.27640118502220545, 18.64703902303423178 ) ) ;
#2418=CARTESIAN_POINT ( 'NONE',  ( -12.73056545648133131, 11.29944703097526748, 19.08155846658118904 ) ) ;
#2419=CARTESIAN_POINT ( 'NONE',  ( -19.94274101607341976, 1.513210029880958984, 6.919864475265770309 ) ) ;
#2426=CARTESIAN_POINT ( 'NONE',  ( 15.81223572262637589, -6.365019322297389870, 7.652108011868850923 ) ) ;
#2427=EDGE_CURVE ( 'NONE', #25701, #23467, #2974, .T. ) ;
#2429=CARTESIAN_POINT ( 'NONE',  ( -12.90456292687989759, 11.10871050118981529, 7.359006845440219102 ) ) ;
#2430=DIRECTION ( 'NONE',  ( -0.000000000000000000, -0.000000000000000000, 1.000000000000000000 ) ) ;
#2434=CARTESIAN_POINT ( 'NONE',  ( 15.39534585122290267, -7.260971684546492000, 19.11611934778430921 ) ) ;
#2435=AXIS2_PLACEMENT_3D ( 'NONE', #26630, #22244, #881 ) ;
#2438=ORIENTED_EDGE ( 'NONE', *, *, #30578, .F. ) ;
#2439=CARTESIAN_POINT ( 'NONE',  ( 5.008980049945718882, 16.26773947435520284, 19.22654678686458141 ) ) ;
#2448=AXIS2_PLACEMENT_3D ( 'NONE', #30312, #20786, #16123 ) ;
#2450=ORIENTED_EDGE ( 'NONE', *, *, #5383, .T. ) ;
#2451=CARTESIAN_POINT ( 'NONE',  ( -15.21426671708081635, -7.679208962302483066, 7.652108011868850035 ) ) ;
#2452=CARTESIAN_POINT ( 'NONE',  ( 14.32702845807335734, 13.95510847468387539, 6.037995405461177079 ) ) ;
#2454=VECTOR ( 'NONE', #22694, 1000.000000000000000 ) ;
#2457=CARTESIAN_POINT ( 'NONE',  ( -16.98316914218901275, 1.504314895146018127, 20.33971507717571114 ) ) ;
#2459=ORIENTED_EDGE ( 'NONE', *, *, #2894, .T. ) ;
#2460=CARTESIAN_POINT ( 'NONE',  ( 11.70583205457081988, -16.23839729645240126, 20.06253562465620632 ) ) ;
#2465=CARTESIAN_POINT ( 'NONE',  ( 4.308942857043133401, 19.53031007734547941, 19.48477075383299706 ) ) ;
#2471=LINE ( 'NONE', #26482, #12697 ) ;
#2472=CARTESIAN_POINT ( 'NONE',  ( -10.62374177707235035, -16.96647932868177122, 7.652108011868850035 ) ) ;
#2473=VERTEX_POINT ( 'NONE', #29396 ) ;
#2474=CARTESIAN_POINT ( 'NONE',  ( 16.06085112851923924, -5.768724642094689159, 18.56793045041961321 ) ) ;
#2475=CARTESIAN_POINT ( 'NONE',  ( 19.61965483366450513, 3.971857776421114483, 19.97651184436794125 ) ) ;
#2477=ORIENTED_EDGE ( 'NONE', *, *, #27904, .T. ) ;
#2483=CARTESIAN_POINT ( 'NONE',  ( -17.81689967073718250, -9.086958408757460859, 5.779535427900762912 ) ) ;
#2484=AXIS2_PLACEMENT_3D ( 'NONE', #7571, #28780, #26752 ) ;
#2487=CARTESIAN_POINT ( 'NONE',  ( 1.795426799894649594, -16.98366215210793584, 19.28454053338349183 ) ) ;
#2490=ORIENTED_EDGE ( 'NONE', *, *, #12020, .F. ) ;
#2491=CARTESIAN_POINT ( 'NONE',  ( -19.71077436674131533, 3.493128416889933252, 19.22654678686458141 ) ) ;
#2501=CARTESIAN_POINT ( 'NONE',  ( 11.65972768484890665, 12.47873923859707190, 6.783738457429052460 ) ) ;
#2502=AXIS2_PLACEMENT_3D ( 'NONE', #6433, #16235, #16093 ) ;
#2506=EDGE_CURVE ( 'NONE', #8832, #12097, #26221, .T. ) ;
#2507=VERTEX_POINT ( 'NONE', #2064 ) ;
#2508=MANIFOLD_SOLID_BREP ( 'Cut-Extrude26', #11827 ) ;
#2511=CARTESIAN_POINT ( 'NONE',  ( -18.04365185506139113, -8.627086862512678422, 20.34789198813115263 ) ) ;
#2513=DIRECTION ( 'NONE',  ( -1.000000000000000000, 0.000000000000000000, 0.000000000000000000 ) ) ;
#2516=CARTESIAN_POINT ( 'NONE',  ( 13.00882613046785607, 10.97723423515713215, 6.530762810602277924 ) ) ;
#2518=CARTESIAN_POINT ( 'NONE',  ( 18.72527277698615578, -7.076062192109023208, 6.892848776733236704 ) ) ;
#2523=CARTESIAN_POINT ( 'NONE',  ( 10.08077896146697761, -13.75650449133559405, 20.34789198813114908 ) ) ;
#2526=DIRECTION ( 'NONE',  ( -0.000000000000000000, -0.000000000000000000, 1.000000000000000000 ) ) ;
#2530=ORIENTED_EDGE ( 'NONE', *, *, #7260, .T. ) ;
#2531=EDGE_CURVE ( 'NONE', #24218, #18940, #30664, .T. ) ;
#2533=CARTESIAN_POINT ( 'NONE',  ( -7.827050521741844236, 5.352643706120543854, 1.500000000000001332 ) ) ;
#2534=EDGE_CURVE ( 'NONE', #5487, #3669, #15769, .T. ) ;
#2537=CARTESIAN_POINT ( 'NONE',  ( -15.16517292768934233, -7.781889190071453299, 20.34789198813115263 ) ) ;
#2538=DIRECTION ( 'NONE',  ( 0.000000000000000000, 0.000000000000000000, 1.000000000000000000 ) ) ;
#2540=CARTESIAN_POINT ( 'NONE',  ( 4.985742441154983773, 16.27537970825923352, 6.910395520694541993 ) ) ;
#2542=EDGE_LOOP ( 'NONE', ( #9887, #6401 ) ) ;
#2543=FACE_OUTER_BOUND ( 'NONE', #28543, .T. ) ;
#2546=CARTESIAN_POINT ( 'NONE',  ( -6.565451881449787308, 18.89189346177362694, 5.853797745100183469 ) ) ;
#2548=AXIS2_PLACEMENT_3D ( 'NONE', #29065, #5668, #12386 ) ;
#2555=ORIENTED_EDGE ( 'NONE', *, *, #18538, .T. ) ;
#2556=DIRECTION ( 'NONE',  ( 0.000000000000000000, 0.000000000000000000, -1.000000000000000000 ) ) ;
#2559=ORIENTED_EDGE ( 'NONE', *, *, #1389, .F. ) ;
#2560=CARTESIAN_POINT ( 'NONE',  ( -0.09481216811183737492, -20.01790837231453324, 20.25336174263950184 ) ) ;
#2561=EDGE_CURVE ( 'NONE', #10914, #19471, #2379, .T. ) ;
#2562=CARTESIAN_POINT ( 'NONE',  ( -9.169883732660077058, -9.268939115642981008, 1.500000000000001332 ) ) ;
#2565=CARTESIAN_POINT ( 'NONE',  ( 0.6919288935074129343, -20.00608154967867947, 18.39992786714538298 ) ) ;
#2568=CARTESIAN_POINT ( 'NONE',  ( -15.75094665830067697, -12.32508334119358828, 24.50000000000000000 ) ) ;
#2569=CARTESIAN_POINT ( 'NONE',  ( 14.46722394715956916, 13.83532015011946292, 20.13759033520874908 ) ) ;
#2576=DIRECTION ( 'NONE',  ( 0.000000000000000000, 0.000000000000000000, 1.000000000000000000 ) ) ;
#2578=CARTESIAN_POINT ( 'NONE',  ( -15.39003174319561218, -7.295547530644703293, 18.49267272388512140 ) ) ;
#2579=LINE ( 'NONE', #28156, #30018 ) ;
#2581=ORIENTED_EDGE ( 'NONE', *, *, #17459, .F. ) ;
#2582=DIRECTION ( 'NONE',  ( 1.000000000000000000, 0.000000000000000000, 0.000000000000000000 ) ) ;
#2585=AXIS2_PLACEMENT_3D ( 'NONE', #25823, #4142, #25090 ) ;
#2588=CARTESIAN_POINT ( 'NONE',  ( 16.19472973927114268, -5.422090571236379830, 19.28454053338348473 ) ) ;
#2589=CARTESIAN_POINT ( 'NONE',  ( 6.071284049926377158, 19.07508289763275400, 7.272049892295485485 ) ) ;
#2590=ORIENTED_EDGE ( 'NONE', *, *, #25566, .F. ) ;
#2591=CARTESIAN_POINT ( 'NONE',  ( 6.060672894209299777, 19.07852886212369370, 18.71435384576123440 ) ) ;
#2592=CARTESIAN_POINT ( 'NONE',  ( 14.59923040764597779, 13.69601292063888920, 7.559636331181775581 ) ) ;
#2596=ORIENTED_EDGE ( 'NONE', *, *, #25773, .F. ) ;
#2605=DIRECTION ( 'NONE',  ( 1.000000000000000000, 0.000000000000000000, 0.000000000000000000 ) ) ;
#2612=DIRECTION ( 'NONE',  ( 0.000000000000000000, 0.000000000000000000, -1.000000000000000000 ) ) ;
#2613=ORIENTED_EDGE ( 'NONE', *, *, #2747, .F. ) ;
#2617=ORIENTED_EDGE ( 'NONE', *, *, #17280, .F. ) ;
#2619=AXIS2_PLACEMENT_3D ( 'NONE', #23778, #2430, #11212 ) ;
#2622=CARTESIAN_POINT ( 'NONE',  ( 16.15906311113806382, -5.516254886378318290, 19.79423548914561692 ) ) ;
#2623=CARTESIAN_POINT ( 'NONE',  ( 16.64821571380337772, 3.734651121118245154, 18.50655187082627862 ) ) ;
#2626=CARTESIAN_POINT ( 'NONE',  ( 15.55638214359055205, -6.928938690483699148, 20.14907003336613656 ) ) ;
#2633=B_SPLINE_CURVE_WITH_KNOTS ( 'NONE', 3,
 ( #2001, #18845, #19145, #9170, #13706, #18539, #28189, #6986, #16496, #26015, #11522, #21006, #30526, #28817, #14760, #24433 ),
 .UNSPECIFIED., .F., .F.,
 ( 4, 2, 2, 2, 2, 2, 2, 4 ),
 ( 0.5000000000000000000, 0.6250000000000001110, 0.6875000000000001110, 0.7187500000000002220, 0.7500000000000004441, 0.8125000000000002220, 0.8750000000000000000, 1.000000000000000000 ),
 .UNSPECIFIED. ) ;
#2636=DIRECTION ( 'NONE',  ( -0.000000000000000000, -0.000000000000000000, 1.000000000000000000 ) ) ;
#2637=CARTESIAN_POINT ( 'NONE',  ( 8.743977807160073112, 3.668292057956029861, 21.50000000000000000 ) ) ;
#2640=CARTESIAN_POINT ( 'NONE',  ( -19.77235582619724497, 3.126546698941336189, 18.55820869691756769 ) ) ;
#2644=ORIENTED_EDGE ( 'NONE', *, *, #19672, .T. ) ;
#2648=DIRECTION ( 'NONE',  ( 1.000000000000000000, 0.000000000000000000, 0.000000000000000000 ) ) ;
#2651=DIRECTION ( 'NONE',  ( -0.7557495743542581579, -0.6548607339452852116, 0.000000000000000000 ) ) ;
#2657=CARTESIAN_POINT ( 'NONE',  ( 0.000000000000000000, 0.000000000000000000, 1.500000000000001332 ) ) ;
#2674=CARTESIAN_POINT ( 'NONE',  ( -9.169883732660077058, -9.268939115642981008, 24.50000000000000000 ) ) ;
#2675=CARTESIAN_POINT ( 'NONE',  ( 0.3518703668723784928, -19.99690444156084723, 20.34789198813115263 ) ) ;
#2677=CARTESIAN_POINT ( 'NONE',  ( 15.60425753239542956, -6.827323759751870114, 7.526951045817046548 ) ) ;
#2680=CARTESIAN_POINT ( 'NONE',  ( -3.668292057955944152, 8.743977807160112192, 1.500000000000001332 ) ) ;
#2681=EDGE_LOOP ( 'NONE', ( #7169, #22145, #23971, #18570 ) ) ;
#2686=CARTESIAN_POINT ( 'NONE',  ( -6.587096388939656322, -18.88412458026101248, 24.50000000000000000 ) ) ;
#2689=CARTESIAN_POINT ( 'NONE',  ( 4.049916833591940879, 16.55712665779027049, 7.652108011868850923 ) ) ;
#2693=DIRECTION ( 'NONE',  ( 0.1423148382732746797, -0.9898214418809342385, 0.000000000000000000 ) ) ;
#2696=ORIENTED_EDGE ( 'NONE', *, *, #29078, .T. ) ;
#2700=EDGE_CURVE ( 'NONE', #8580, #3764, #11300, .T. ) ;
#2701=VERTEX_POINT ( 'NONE', #22173 ) ;
#2703=LINE ( 'NONE', #19225, #6778 ) ;
#2712=CARTESIAN_POINT ( 'NONE',  ( 0.000000000000000000, 0.000000000000000000, 1.500000000000001332 ) ) ;
#2714=CARTESIAN_POINT ( 'NONE',  ( -8.079801766074020009, -15.02755831366981099, 5.810767894563978686 ) ) ;
#2715=CARTESIAN_POINT ( 'NONE',  ( 4.894722408918116940, 16.30505022503850299, 19.85270094495842130 ) ) ;
#2716=CARTESIAN_POINT ( 'NONE',  ( 0.8008512464130190800, -20.00192252186467812, 18.44527579819791185 ) ) ;
#2717=ORIENTED_EDGE ( 'NONE', *, *, #29979, .T. ) ;
#2719=DIRECTION ( 'NONE',  ( -0.000000000000000000, -0.000000000000000000, -1.000000000000000000 ) ) ;
#2720=DIRECTION ( 'NONE',  ( -0.000000000000000000, -0.000000000000000000, 1.000000000000000000 ) ) ;
#2722=CARTESIAN_POINT ( 'NONE',  ( 12.20325286834225054, 11.91007939804258164, 18.37415474056476938 ) ) ;
#2723=DIRECTION ( 'NONE',  ( 0.000000000000000000, 0.000000000000000000, 1.000000000000000000 ) ) ;
#2728=CARTESIAN_POINT ( 'NONE',  ( -5.978582532085230383, 19.10413086404602723, 5.652196082364320695 ) ) ;
#2730=CARTESIAN_POINT ( 'NONE',  ( -19.93487782419341059, 1.613472484145544117, 6.149077423860693337 ) ) ;
#2734=EDGE_LOOP ( 'NONE', ( #21039, #4845, #11777, #25394 ) ) ;
#2735=ORIENTED_EDGE ( 'NONE', *, *, #27082, .T. ) ;
#2736=CARTESIAN_POINT ( 'NONE',  ( -11.82521593960875528, 5.400395169024524655, 1.500000000000001332 ) ) ;
#2739=CARTESIAN_POINT ( 'NONE',  ( -13.02230393242516371, 10.97666050933785975, 7.500898271101006820 ) ) ;
#2740=CARTESIAN_POINT ( 'NONE',  ( 11.52514311384751089, -16.34582042812247238, 20.22386025856690139 ) ) ;
#2747=EDGE_CURVE ( 'NONE', #1188, #20273, #17259, .T. ) ;
#2748=CARTESIAN_POINT ( 'NONE',  ( 12.30878326772641884, 11.79452912058117775, 7.652108011868850035 ) ) ;
#2754=ADVANCED_FACE ( 'NONE', ( #1595 ), #8922, .F. ) ;
#2757=ORIENTED_EDGE ( 'NONE', *, *, #10591, .F. ) ;
#2758=CARTESIAN_POINT ( 'NONE',  ( -15.39438215884103656, -7.285634741961049876, 7.500898271101006820 ) ) ;
#2759=CIRCLE ( 'NONE', #12737, 0.7500000000000006661 ) ;
#2762=DIRECTION ( 'NONE',  ( 0.000000000000000000, 0.000000000000000000, 1.000000000000000000 ) ) ;
#2763=LINE ( 'NONE', #7914, #10783 ) ;
#2770=CARTESIAN_POINT ( 'NONE',  ( 5.291489565152560637, 19.28730510418394317, 5.652196082369965069 ) ) ;
#2776=ORIENTED_EDGE ( 'NONE', *, *, #7868, .F. ) ;
#2777=EDGE_CURVE ( 'NONE', #16205, #30019, #23085, .T. ) ;
#2779=CARTESIAN_POINT ( 'NONE',  ( -10.71492722147446131, -16.90904491356049988, 5.670038381137163519 ) ) ;
#2781=CARTESIAN_POINT ( 'NONE',  ( 16.02447511960549775, -5.858916503155148447, 18.50655187082627862 ) ) ;
#2782=CARTESIAN_POINT ( 'NONE',  ( 19.57334175050933567, 4.193940174973931789, 19.36813350477385143 ) ) ;
#2786=FACE_OUTER_BOUND ( 'NONE', #9152, .T. ) ;
#2787=VERTEX_POINT ( 'NONE', #26971 ) ;
#2788=EDGE_LOOP ( 'NONE', ( #2617, #20175, #12784, #1406 ) ) ;
#2789=CARTESIAN_POINT ( 'NONE',  ( -6.934698339095106689, 18.77804097180239751, 19.47783254395485031 ) ) ;
#2796=EDGE_LOOP ( 'NONE', ( #17529, #23908, #24244, #26508 ) ) ;
#2797=CARTESIAN_POINT ( 'NONE',  ( 9.007065134480614077, -14.44288896217592821, 6.755862304746362845 ) ) ;
#2799=VECTOR ( 'NONE', #4047, 1000.000000000000000 ) ;
#2800=CARTESIAN_POINT ( 'NONE',  ( 2.703030265324084080, -12.75514121382991384, 1.500000000000001332 ) ) ;
#2802=ORIENTED_EDGE ( 'NONE', *, *, #2700, .T. ) ;
#2803=CYLINDRICAL_SURFACE ( 'NONE', #1387, 0.7499999999999988898 ) ;
#2804=CARTESIAN_POINT ( 'NONE',  ( -8.637616862297813114, 3.912171961292039590, 21.50000000000000000 ) ) ;
#2806=DIRECTION ( 'NONE',  ( 1.000000000000000000, 0.000000000000000000, 0.000000000000000000 ) ) ;
#2810=VERTEX_POINT ( 'NONE', #10580 ) ;
#2814=CARTESIAN_POINT ( 'NONE',  ( -17.81689967073718961, -9.086958408757471517, 18.47531940416305929 ) ) ;
#2818=CARTESIAN_POINT ( 'NONE',  ( 12.77540468287706155, 11.25967455357098856, 7.429667576816606278 ) ) ;
#2820=FACE_BOUND ( 'NONE', #5046, .T. ) ;
#2821=AXIS2_PLACEMENT_3D ( 'NONE', #13960, #27697, #20956 ) ;
#2822=CARTESIAN_POINT ( 'NONE',  ( 16.70106355290392486, 3.455140589318408395, 20.34789198813114197 ) ) ;
#2829=AXIS2_PLACEMENT_3D ( 'NONE', #27971, #11280, #16257 ) ;
#2831=FACE_OUTER_BOUND ( 'NONE', #19525, .T. ) ;
#2832=ORIENTED_EDGE ( 'NONE', *, *, #5159, .T. ) ;
#2839=CARTESIAN_POINT ( 'NONE',  ( -17.59891439103366295, -9.538503746949027473, 19.36813350477385143 ) ) ;
#2840=CARTESIAN_POINT ( 'NONE',  ( 0.000000000000000000, 0.000000000000000000, 1.500000000000001332 ) ) ;
#2848=EDGE_CURVE ( 'NONE', #24160, #16362, #1227, .T. ) ;
#2850=ORIENTED_EDGE ( 'NONE', *, *, #13038, .F. ) ;
#2858=AXIS2_PLACEMENT_3D ( 'NONE', #17489, #27011, #324 ) ;
#2860=AXIS2_PLACEMENT_3D ( 'NONE', #5277, #28834, #7311 ) ;
#2862=ORIENTED_EDGE ( 'NONE', *, *, #24030, .F. ) ;
#2863=CARTESIAN_POINT ( 'NONE',  ( 0.06889080212830860084, -17.02733034922398758, 18.63641924841378028 ) ) ;
#2866=FACE_OUTER_BOUND ( 'NONE', #24748, .T. ) ;
#2868=ORIENTED_EDGE ( 'NONE', *, *, #15299, .T. ) ;
#2871=CARTESIAN_POINT ( 'NONE',  ( 14.74216733233971866, 13.54174064842195691, 18.37415474056476938 ) ) ;
#2879=CARTESIAN_POINT ( 'NONE',  ( -6.656778417335411646, 18.87854210339738970, 7.366751648393900176 ) ) ;
#2881=CARTESIAN_POINT ( 'NONE',  ( -8.413215745754975217, 3.196529495465474380, 1.500000000000001332 ) ) ;
#2885=CARTESIAN_POINT ( 'NONE',  ( -18.15569024355516703, -8.431866758338669499, 18.36582235739946611 ) ) ;
#2887=AXIS2_PLACEMENT_3D ( 'NONE', #100, #12263, #26458 ) ;
#2889=ORIENTED_EDGE ( 'NONE', *, *, #11376, .T. ) ;
#2893=CARTESIAN_POINT ( 'NONE',  ( -12.81275022540756581, 11.20978530020977004, 7.176035686813569292 ) ) ;
#2894=EDGE_CURVE ( 'NONE', #27397, #4887, #20563, .T. ) ;
#2895=CARTESIAN_POINT ( 'NONE',  ( 13.00999358272542850, -0.8602714556717643291, 24.50000000000000000 ) ) ;
#2899=CARTESIAN_POINT ( 'NONE',  ( 4.082218581380957723, 16.54825969530613961, 5.651989602109218858 ) ) ;
#2903=CARTESIAN_POINT ( 'NONE',  ( 4.731053074881896414, 16.35701261131971407, 18.63641924841378028 ) ) ;
#2904=CIRCLE ( 'NONE', #400, 9.482273699623480212 ) ;
#2906=ADVANCED_FACE ( 'NONE', ( #15089 ), #21142, .F. ) ;
#2907=VECTOR ( 'NONE', #22583, 1000.000000000000000 ) ;
#2914=VECTOR ( 'NONE', #7549, 1000.000000000000227 ) ;
#2916=CARTESIAN_POINT ( 'NONE',  ( -15.34842816977634428, -7.387654668753818932, 5.749228751562096562 ) ) ;
#2918=CARTESIAN_POINT ( 'NONE',  ( 8.413215745754998309, -3.196529495465417980, 21.50000000000000000 ) ) ;
#2926=EDGE_CURVE ( 'NONE', #13104, #10035, #23491, .T. ) ;
#2931=AXIS2_PLACEMENT_3D ( 'NONE', #27902, #7138, #23498 ) ;
#2933=CIRCLE ( 'NONE', #7924, 0.7500000000000006661 ) ;
#2941=CARTESIAN_POINT ( 'NONE',  ( 12.88134121443596847, 11.13293444107316610, 19.96783386855779341 ) ) ;
#2942=CARTESIAN_POINT ( 'NONE',  ( -9.272241372864392872, -14.27765368465080265, 7.176035686813569292 ) ) ;
#2945=CARTESIAN_POINT ( 'NONE',  ( 16.19384365167807971, -5.424445124423259657, 19.47783254395485031 ) ) ;
#2946=CARTESIAN_POINT ( 'NONE',  ( -15.34307810681595186, 12.82926163924265950, 20.34789198813115263 ) ) ;
#2952=AXIS2_PLACEMENT_3D ( 'NONE', #29409, #14440, #696 ) ;
#2954=ADVANCED_FACE ( 'NONE', ( #25692 ), #28180, .F. ) ;
#2956=CARTESIAN_POINT ( 'NONE',  ( -6.449126838413864249, 15.81136745782586672, 19.69140814234746273 ) ) ;
#2957=CARTESIAN_POINT ( 'NONE',  ( -17.98703099176684006, -8.745510052321849415, 7.652108011868850923 ) ) ;
#2959=VECTOR ( 'NONE', #26841, 1000.000000000000000 ) ;
#2960=CARTESIAN_POINT ( 'NONE',  ( -7.669844488642329594, -15.25924058316908649, 19.25672174529527325 ) ) ;
#2962=CARTESIAN_POINT ( 'NONE',  ( 19.74328841314636307, 3.194145055459935101, 20.34789198813115263 ) ) ;
#2963=DIRECTION ( 'NONE',  ( -0.000000000000000000, -0.000000000000000000, 1.000000000000000000 ) ) ;
#2964=CARTESIAN_POINT ( 'NONE',  ( -19.87987511945007313, 2.346632672767392958, 5.661398277488801867 ) ) ;
#2965=AXIS2_PLACEMENT_3D ( 'NONE', #4053, #13580, #23058 ) ;
#2968=ORIENTED_EDGE ( 'NONE', *, *, #8843, .T. ) ;
#2973=CARTESIAN_POINT ( 'NONE',  ( -15.27764744547075182, -7.543477926807485190, 7.626437579292365321 ) ) ;
#2974=CIRCLE ( 'NONE', #24375, 20.00000000000000000 ) ;
#2975=LINE ( 'NONE', #615, #6934 ) ;
#2976=ORIENTED_EDGE ( 'NONE', *, *, #14850, .T. ) ;
#2977=DIRECTION ( 'NONE',  ( 1.000000000000000000, 0.000000000000000000, 0.000000000000000000 ) ) ;
#2978=FACE_BOUND ( 'NONE', #6436, .T. ) ;
#2979=CARTESIAN_POINT ( 'NONE',  ( 19.88003893156456670, 2.345734461008499583, 6.111214848085761986 ) ) ;
#2981=CARTESIAN_POINT ( 'NONE',  ( 15.31432103507273546, 12.89133701742166771, 7.429667576816606278 ) ) ;
#2983=CARTESIAN_POINT ( 'NONE',  ( 15.84193441942129077, -6.296838616230743924, 7.652108011868850035 ) ) ;
#2986=DIRECTION ( 'NONE',  ( 0.000000000000000000, 0.000000000000000000, 1.000000000000000000 ) ) ;
#2987=ORIENTED_EDGE ( 'NONE', *, *, #2137, .F. ) ;
#2988=CARTESIAN_POINT ( 'NONE',  ( 4.772488686130579971, 19.44046140540703504, 5.810767894563978686 ) ) ;
#2990=CARTESIAN_POINT ( 'NONE',  ( -4.622016212553093695, -12.19167610014704906, 24.50000000000000000 ) ) ;
#2999=CARTESIAN_POINT ( 'NONE',  ( -13.83904721019128381, 9.990416291640222823, 18.64703902303423178 ) ) ;
#3000=CYLINDRICAL_SURFACE ( 'NONE', #14301, 0.7500000000000006661 ) ;
#3005=DIRECTION ( 'NONE',  ( 0.000000000000000000, 0.000000000000000000, 1.000000000000000000 ) ) ;
#3008=CARTESIAN_POINT ( 'NONE',  ( 16.87575838019271757, 2.225846228045831321, 6.910395520694542881 ) ) ;
#3014=CARTESIAN_POINT ( 'NONE',  ( 0.000000000000000000, 0.000000000000000000, 1.500000000000001332 ) ) ;
#3017=CARTESIAN_POINT ( 'NONE',  ( -9.660978277356432997, -17.51194513905169714, 6.919864475265763204 ) ) ;
#3019=AXIS2_PLACEMENT_3D ( 'NONE', #14015, #30689, #7469 ) ;
#3021=ORIENTED_EDGE ( 'NONE', *, *, #16237, .F. ) ;
#3024=CARTESIAN_POINT ( 'NONE',  ( 0.7836604620899301210, -17.02735026737548552, 5.652196082368483587 ) ) ;
#3027=ORIENTED_EDGE ( 'NONE', *, *, #6894, .F. ) ;
#3028=CARTESIAN_POINT ( 'NONE',  ( -10.62668044795002942, -16.94375577056505122, 7.652108011868850035 ) ) ;
#3029=CARTESIAN_POINT ( 'NONE',  ( 0.000000000000000000, 0.000000000000000000, 1.500000000000001332 ) ) ;
#3036=CARTESIAN_POINT ( 'NONE',  ( 11.64616783614240880, -16.28139325077859212, 5.872146474157316831 ) ) ;
#3037=CIRCLE ( 'NONE', #15993, 9.482273699623480212 ) ;
#3043=LINE ( 'NONE', #10373, #10161 ) ;
#3044=CARTESIAN_POINT ( 'NONE',  ( -15.13676175850366512, 13.09931225869579308, 7.595116371587256054 ) ) ;
#3049=LINE ( 'NONE', #12418, #16687 ) ;
#3051=DIRECTION ( 'NONE',  ( -0.000000000000000000, -0.000000000000000000, -1.000000000000000000 ) ) ;
#3052=CARTESIAN_POINT ( 'NONE',  ( 3.662523238938590442, -12.47340865698848056, 1.500000000000001332 ) ) ;
#3059=CIRCLE ( 'NONE', #7036, 0.7500000000000004441 ) ;
#3061=CARTESIAN_POINT ( 'NONE',  ( -19.69679205574297498, 3.469720661875630885, 19.60917204426171168 ) ) ;
#3062=VERTEX_POINT ( 'NONE', #14915 ) ;
#3063=FACE_OUTER_BOUND ( 'NONE', #14383, .T. ) ;
#3065=EDGE_CURVE ( 'NONE', #15686, #4883, #21170, .T. ) ;
#3076=ORIENTED_EDGE ( 'NONE', *, *, #19874, .T. ) ;
#3082=EDGE_LOOP ( 'NONE', ( #30567, #28647, #13272, #27650 ) ) ;
#3085=CARTESIAN_POINT ( 'NONE',  ( 15.53918631077679180, 12.61944498292910488, 19.11611934778430921 ) ) ;
#3086=CARTESIAN_POINT ( 'NONE',  ( -11.29739510359497245, -16.52539200402570785, 7.080843742048788414 ) ) ;
#3088=CARTESIAN_POINT ( 'NONE',  ( -16.90489691178406062, 2.092419235659074506, 7.557577766377196582 ) ) ;
#3089=CARTESIAN_POINT ( 'NONE',  ( 18.08129319977582838, -8.548428815984333795, 5.849008070840543638 ) ) ;
#3090=DIRECTION ( 'NONE',  ( -0.8412535328311804284, 0.5406408174555987767, 0.000000000000000000 ) ) ;
#3091=ORIENTED_EDGE ( 'NONE', *, *, #11882, .T. ) ;
#3093=EDGE_CURVE ( 'NONE', #23779, #12979, #11296, .T. ) ;
#3102=CARTESIAN_POINT ( 'NONE',  ( -6.938992678473724141, 18.77645360485810144, 19.25672174529527325 ) ) ;
#3103=CARTESIAN_POINT ( 'NONE',  ( -14.82920317518825293, 13.44671003463071735, 19.96783386855779341 ) ) ;
#3104=CIRCLE ( 'NONE', #29941, 9.482273699623480212 ) ;
#3106=EDGE_CURVE ( 'NONE', #15032, #27003, #14455, .T. ) ;
#3110=VERTEX_POINT ( 'NONE', #12273 ) ;
#3112=CARTESIAN_POINT ( 'NONE',  ( -19.90092023446657521, 2.162276205174161081, 5.704143890883081269 ) ) ;
#3114=CARTESIAN_POINT ( 'NONE',  ( 19.87928744571104289, 2.194067154482769677, 6.781503518395076036 ) ) ;
#3117=DIRECTION ( 'NONE',  ( -0.000000000000000000, -0.000000000000000000, 1.000000000000000000 ) ) ;
#3119=CARTESIAN_POINT ( 'NONE',  ( -4.163336342344337027E-14, 1.387778780781445676E-14, 1.500000000000000000 ) ) ;
#3120=ORIENTED_EDGE ( 'NONE', *, *, #18921, .F. ) ;
#3121=DIRECTION ( 'NONE',  ( 0.000000000000000000, 0.000000000000000000, 1.000000000000000000 ) ) ;
#3122=DIRECTION ( 'NONE',  ( 1.000000000000000000, 0.000000000000000000, 0.000000000000000000 ) ) ;
#3128=CARTESIAN_POINT ( 'NONE',  ( 16.86769344895232337, 2.296683858978091575, 6.211014596808754007 ) ) ;
#3130=CARTESIAN_POINT ( 'NONE',  ( 15.55295851173241672, 12.60248606922869463, 6.755862304746362845 ) ) ;
#3133=CARTESIAN_POINT ( 'NONE',  ( 18.55936137128098196, -7.500557692851355540, 7.500147780736496017 ) ) ;
#3137=ORIENTED_EDGE ( 'NONE', *, *, #11882, .F. ) ;
#3145=CARTESIAN_POINT ( 'NONE',  ( 9.135582339684646058, -14.36547911245297549, 19.87181966307587544 ) ) ;
#3146=VERTEX_POINT ( 'NONE', #3687 ) ;
#3149=DIRECTION ( 'NONE',  ( 1.000000000000000000, 0.000000000000000000, 0.000000000000000000 ) ) ;
#3152=CARTESIAN_POINT ( 'NONE',  ( 0.000000000000000000, 0.000000000000000000, 1.500000000000001332 ) ) ;
#3153=B_SPLINE_SURFACE_WITH_KNOTS ( 'NONE', 3, 1, ( 
 ( #24341, #3283 ),
 ( #19362, #19197 ),
 ( #5012, #7362 ),
 ( #24019, #28883 ),
 ( #5163, #24173 ),
 ( #12348, #10005 ),
 ( #2988, #27773 ),
 ( #8595, #22925 ),
 ( #5942, #19976 ),
 ( #20440, #29813 ),
 ( #24808, #3755 ),
 ( #3919, #3598 ),
 ( #13275, #15440 ),
 ( #10941, #6086 ),
 ( #8455, #18100 ),
 ( #952, #22615 ),
 ( #13121, #20286 ),
 ( #8284, #6402 ),
 ( #10617, #29496 ),
 ( #27618, #6241 ),
 ( #17800, #1573 ),
 ( #27465, #11080 ),
 ( #5783, #15749 ),
 ( #3445, #20577 ),
 ( #8131, #30103 ),
 ( #18253, #22767 ),
 ( #15922, #13586 ),
 ( #12966, #27314 ),
 ( #1263, #10463 ),
 ( #17640, #24961 ),
 ( #20130, #27157 ) ),
 .UNSPECIFIED., .F., .F., .F.,
 ( 4, 3, 3, 3, 3, 3, 3, 3, 3, 3, 4 ),
 ( 2, 2 ),
 ( 0.4999999998345677765, 0.5360336730431942698, 0.5907651151589017324, 0.6456034593241839481, 0.6998270958050443191, 0.7529536536315944995, 0.8052385063053264513, 0.8575343587103996246, 0.9106564858195047574, 0.9648414833209688624, 1.000000006602610014 ),
 ( 0.000000000000000000, 1.000000000000000000 ),
 .UNSPECIFIED. ) ;
#3154=CARTESIAN_POINT ( 'NONE',  ( -14.67655575066035567, 13.58671083542089164, 19.21471108562413832 ) ) ;
#3161=CARTESIAN_POINT ( 'NONE',  ( 19.72123249184183180, 3.330269068327012416, 5.652912763329821288 ) ) ;
#3164=EDGE_CURVE ( 'NONE', #7313, #12572, #3448, .T. ) ;
#3166=CARTESIAN_POINT ( 'NONE',  ( -1.438332125858111432, 8.884323311075791096, 1.500000000000001332 ) ) ;
#3170=DIRECTION ( 'NONE',  ( 0.5406408174555974444, 0.8412535328311813165, 0.000000000000000000 ) ) ;
#3171=EDGE_LOOP ( 'NONE', ( #8120, #8402, #16204, #20861 ) ) ;
#3172=ORIENTED_EDGE ( 'NONE', *, *, #29040, .T. ) ;
#3174=LINE ( 'NONE', #15164, #5307 ) ;
#3180=VECTOR ( 'NONE', #5263, 1000.000000000000114 ) ;
#3183=DIRECTION ( 'NONE',  ( 0.6548607339452889864, 0.7557495743542548272, 0.000000000000000000 ) ) ;
#3186=VECTOR ( 'NONE', #22517, 1000.000000000000000 ) ;
#3187=CARTESIAN_POINT ( 'NONE',  ( -9.272241372864389319, -14.27765368465079554, 19.87181966307587544 ) ) ;
#3189=CARTESIAN_POINT ( 'NONE',  ( -6.889674169070709731, 18.79461648230378046, 6.341840715582230281 ) ) ;
#3190=CARTESIAN_POINT ( 'NONE',  ( 11.94417982595701488, -16.06366807669216357, 6.782048567692550378 ) ) ;
#3193=ORIENTED_EDGE ( 'NONE', *, *, #21172, .F. ) ;
#3194=ORIENTED_EDGE ( 'NONE', *, *, #11481, .T. ) ;
#3196=CARTESIAN_POINT ( 'NONE',  ( -14.69323076807464723, 13.59505578765952549, 6.530762810602277924 ) ) ;
#3198=EDGE_LOOP ( 'NONE', ( #19255, #16334, #11393, #10706 ) ) ;
#3199=CARTESIAN_POINT ( 'NONE',  ( 15.79886199502268695, -6.395730384537282376, 18.34777357837152323 ) ) ;
#3203=DIRECTION ( 'NONE',  ( -0.000000000000000000, -0.000000000000000000, 1.000000000000000000 ) ) ;
#3205=CARTESIAN_POINT ( 'NONE',  ( -7.671759676023388153, -15.25818751172876553, 19.47952243369110192 ) ) ;
#3209=DIRECTION ( 'NONE',  ( 0.000000000000000000, 0.000000000000000000, 1.000000000000000000 ) ) ;
#3210=CYLINDRICAL_SURFACE ( 'NONE', #17248, 20.00000000000000355 ) ;
#3224=CARTESIAN_POINT ( 'NONE',  ( 4.507962051892418387, 19.48556068265256513, 6.037995405461189513 ) ) ;
#3231=CARTESIAN_POINT ( 'NONE',  ( 12.91913032519423865, 11.08701612049549823, 19.87181966307587544 ) ) ;
#3232=ORIENTED_EDGE ( 'NONE', *, *, #68, .T. ) ;
#3235=CARTESIAN_POINT ( 'NONE',  ( 16.73141127408299411, 3.267558643021993614, 20.34789198813115263 ) ) ;
#3237=ORIENTED_EDGE ( 'NONE', *, *, #12204, .T. ) ;
#3238=CARTESIAN_POINT ( 'NONE',  ( -4.950721362025076289, 16.29421905982281871, 20.14907003336613300 ) ) ;
#3239=CIRCLE ( 'NONE', #17169, 0.7499999999999997780 ) ;
#3244=CARTESIAN_POINT ( 'NONE',  ( 19.70397673731431709, 3.532048315275338357, 5.704143890883081269 ) ) ;
#3246=CARTESIAN_POINT ( 'NONE',  ( -10.14013680258725891, -17.25966085745527678, 18.44527579819791185 ) ) ;
#3249=CARTESIAN_POINT ( 'NONE',  ( -8.546423435383418976, -14.74799740001549786, 18.34798005863078885 ) ) ;
#3255=ORIENTED_EDGE ( 'NONE', *, *, #18875, .T. ) ;
#3257=CARTESIAN_POINT ( 'NONE',  ( 18.23136487193858102, -8.223889151411999165, 18.37250658438899009 ) ) ;
#3258=EDGE_CURVE ( 'NONE', #4676, #624, #19205, .T. ) ;
#3259=CARTESIAN_POINT ( 'NONE',  ( 10.27753383451899438, -17.15735655630021128, 6.386539667786106378 ) ) ;
#3261=CARTESIAN_POINT ( 'NONE',  ( -4.163336342344337027E-14, 1.387778780781445676E-14, 24.50000000000000000 ) ) ;
#3262=ORIENTED_EDGE ( 'NONE', *, *, #23694, .T. ) ;
#3263=DIRECTION ( 'NONE',  ( 0.000000000000000000, 0.000000000000000000, 1.000000000000000000 ) ) ;
#3271=CARTESIAN_POINT ( 'NONE',  ( 16.87335920545514867, 2.247671665613723668, 6.310736198168394928 ) ) ;
#3272=ORIENTED_EDGE ( 'NONE', *, *, #23873, .T. ) ;
#3273=B_SPLINE_CURVE_WITH_KNOTS ( 'NONE', 3,
 ( #14912, #25036, #22395, #24416, #26933, #15052, #5862, #3061, #12582, #10075, #12734, #870, #3529, #27396, #27227, #17559, #7907, #13046 ),
 .UNSPECIFIED., .F., .F.,
 ( 4, 2, 2, 2, 2, 2, 2, 2, 4 ),
 ( 0.003174295595554305679, 0.003570702171545538008, 0.003967108747536769904, 0.004363515323528002234, 0.004759921899519234563, 0.005156328475510466025, 0.005552735051501698355, 0.005949141627492930684, 0.006345548203484163013 ),
 .UNSPECIFIED. ) ;
#3275=EDGE_LOOP ( 'NONE', ( #23322, #11740, #13472, #3657 ) ) ;
#3281=CIRCLE ( 'NONE', #15728, 9.482273699623480212 ) ;
#3283=CARTESIAN_POINT ( 'NONE',  ( 4.045241160498771471, 16.55840174588941238, 5.652196082364323360 ) ) ;
#3285=DIRECTION ( 'NONE',  ( 1.000000000000000000, 0.000000000000000000, 0.000000000000000000 ) ) ;
#3289=CARTESIAN_POINT ( 'NONE',  ( 9.027514758752761992, -14.43064536408542509, 19.56050940960062690 ) ) ;
#3291=ORIENTED_EDGE ( 'NONE', *, *, #14151, .T. ) ;
#3293=CARTESIAN_POINT ( 'NONE',  ( -13.43037651602831950, 10.49991632925268625, 18.34838970509067479 ) ) ;
#3311=CIRCLE ( 'NONE', #16750, 0.7500000000000006661 ) ;
#3315=EDGE_LOOP ( 'NONE', ( #23654, #10716, #18880, #14033 ) ) ;
#3318=VECTOR ( 'NONE', #2247, 1000.000000000000000 ) ;
#3326=VECTOR ( 'NONE', #3203, 1000.000000000000000 ) ;
#3329=CARTESIAN_POINT ( 'NONE',  ( 0.000000000000000000, 0.000000000000000000, 1.500000000000001332 ) ) ;
#3330=CARTESIAN_POINT ( 'NONE',  ( 1.009606305713755203, -17.02204649693582539, 5.678370764302467677 ) ) ;
#3332=ORIENTED_EDGE ( 'NONE', *, *, #3333, .F. ) ;
#3333=EDGE_CURVE ( 'NONE', #540, #1715, #28315, .T. ) ;
#3335=EDGE_CURVE ( 'NONE', #17560, #863, #18380, .T. ) ;
#3336=CARTESIAN_POINT ( 'NONE',  ( -11.28665222577991756, -16.53262428680031704, 18.90679857307105749 ) ) ;
#3339=CARTESIAN_POINT ( 'NONE',  ( 11.83189508704695214, -16.14673651688228162, 6.131018562779544823 ) ) ;
#3342=VECTOR ( 'NONE', #12977, 1000.000000000000114 ) ;
#3344=ORIENTED_EDGE ( 'NONE', *, *, #7324, .F. ) ;
#3348=CARTESIAN_POINT ( 'NONE',  ( -0.02429396239064400553, -17.02566277817059159, 6.031926333436653742 ) ) ;
#3351=LINE ( 'NONE', #22381, #13193 ) ;
#3352=FACE_OUTER_BOUND ( 'NONE', #30849, .T. ) ;
#3362=CIRCLE ( 'NONE', #7356, 0.7500000000000006661 ) ;
#3364=DIRECTION ( 'NONE',  ( 0.000000000000000000, 0.000000000000000000, -1.000000000000000000 ) ) ;
#3367=CARTESIAN_POINT ( 'NONE',  ( -18.20229063954115034, -8.330696590476666330, 5.701226463332907279 ) ) ;
#3368=CARTESIAN_POINT ( 'NONE',  ( 12.69259498030721289, 11.35795912669135177, 20.22273502201483808 ) ) ;
#3372=VECTOR ( 'NONE', #28060, 1000.000000000000000 ) ;
#3373=DIRECTION ( 'NONE',  ( -0.000000000000000000, -0.000000000000000000, 1.000000000000000000 ) ) ;
#3377=ADVANCED_FACE ( 'NONE', ( #216 ), #20595, .T. ) ;
#3383=VERTEX_POINT ( 'NONE', #8173 ) ;
#3384=ORIENTED_EDGE ( 'NONE', *, *, #24867, .F. ) ;
#3392=CARTESIAN_POINT ( 'NONE',  ( 13.00026995858111079, 10.98778251907842218, 19.11611934778430921 ) ) ;
#3393=ORIENTED_EDGE ( 'NONE', *, *, #18153, .F. ) ;
#3395=CARTESIAN_POINT ( 'NONE',  ( -19.80066175015358354, 2.942692509523777922, 7.557577766377196582 ) ) ;
#3396=CARTESIAN_POINT ( 'NONE',  ( 19.72466756933792809, 3.412884783584985815, 20.32367522806703874 ) ) ;
#3400=VECTOR ( 'NONE', #29683, 1000.000000000000114 ) ;
#3407=CYLINDRICAL_SURFACE ( 'NONE', #1649, 0.7500000000000006661 ) ;
#3408=B_SPLINE_SURFACE_WITH_KNOTS ( 'NONE', 3, 1, ( 
 ( #23871, #28875 ),
 ( #22146, #17004 ),
 ( #26678, #16700 ),
 ( #7507, #26849 ),
 ( #26527, #5003 ),
 ( #5472, #12179 ),
 ( #2981, #2818 ),
 ( #7805, #26377 ),
 ( #12653, #21992 ),
 ( #19504, #16862 ),
 ( #12340, #771 ),
 ( #17157, #10294 ),
 ( #14663, #10141 ),
 ( #3130, #19189 ),
 ( #21842, #19808 ),
 ( #24486, #2516 ),
 ( #623, #19647 ),
 ( #29168, #26209 ),
 ( #4844, #14516 ),
 ( #14361, #21520 ),
 ( #7351, #17317 ),
 ( #24010, #22301 ),
 ( #1256, #10457 ),
 ( #20275, #29802 ),
 ( #22759, #13269 ),
 ( #24641, #25263 ),
 ( #15590, #8274 ),
 ( #5935, #10611 ),
 ( #8445, #11074 ),
 ( #13114, #20122 ),
 ( #27148, #17951 ) ),
 .UNSPECIFIED., .F., .F., .F.,
 ( 4, 3, 3, 3, 3, 3, 3, 3, 3, 3, 4 ),
 ( 2, 2 ),
 ( 0.000000000000000000, 0.05425176834609633791, 0.1085332949128352958, 0.1623767749169382768, 0.2157504826133063158, 0.2688657508888171455, 0.3218907763505476360, 0.3749548578363336993, 0.4282048033836242107, 0.4818374082110501444, 0.4999999999131656825 ),
 ( 0.000000000000000000, 1.000000000000000000 ),
 .UNSPECIFIED. ) ;
#3409=CARTESIAN_POINT ( 'NONE',  ( 19.66622914841314085, 3.734651121118246042, 5.810767894563978686 ) ) ;
#3411=AXIS2_PLACEMENT_3D ( 'NONE', #19597, #27554, #27238 ) ;
#3412=CARTESIAN_POINT ( 'NONE',  ( -10.46366670609033633, -17.06541516851461893, 20.34789198813115263 ) ) ;
#3414=CARTESIAN_POINT ( 'NONE',  ( 9.958038337755681368, 17.34466697471553331, 24.50000000000000000 ) ) ;
#3415=DIRECTION ( 'NONE',  ( 1.000000000000000000, 0.000000000000000000, 0.000000000000000000 ) ) ;
#3417=CARTESIAN_POINT ( 'NONE',  ( 10.25620417238948434, -17.19090129355371843, 6.641371103590088865 ) ) ;
#3418=CARTESIAN_POINT ( 'NONE',  ( 11.30587609449920272, -16.51930395566530407, 18.37415474056476938 ) ) ;
#3421=ORIENTED_EDGE ( 'NONE', *, *, #25207, .F. ) ;
#3423=CARTESIAN_POINT ( 'NONE',  ( 18.33599632111990374, -7.986941774664180649, 20.34789198813115263 ) ) ;
#3425=CARTESIAN_POINT ( 'NONE',  ( -12.86767874445213877, -1.850092897552710225, 1.500000000000001332 ) ) ;
#3429=DIRECTION ( 'NONE',  ( 0.000000000000000000, 0.000000000000000000, 1.000000000000000000 ) ) ;
#3435=FACE_OUTER_BOUND ( 'NONE', #2408, .T. ) ;
#3436=CARTESIAN_POINT ( 'NONE',  ( 19.86411046155384952, 2.477959627222518613, 7.359006845440219102 ) ) ;
#3445=CARTESIAN_POINT ( 'NONE',  ( 4.690664460087337950, 19.46058373524397922, 7.441806358946449151 ) ) ;
#3446=ADVANCED_FACE ( 'NONE', ( #22042 ), #5519, .T. ) ;
#3448=B_SPLINE_CURVE_WITH_KNOTS ( 'NONE', 3,
 ( #12587, #5706, #29268, #1339, #8061, #17565, #26938, #15366, #27548, #15056, #6174, #15201, #10857, #10397, #7911, #24727 ),
 .UNSPECIFIED., .F., .F.,
 ( 4, 2, 2, 2, 2, 2, 2, 4 ),
 ( 0.5000000000000000000, 0.6250000000000004441, 0.6875000000000007772, 0.7187500000000008882, 0.7500000000000009992, 0.8125000000000007772, 0.8750000000000005551, 1.000000000000000000 ),
 .UNSPECIFIED. ) ;
#3451=EDGE_CURVE ( 'NONE', #15220, #21044, #12860, .T. ) ;
#3457=ADVANCED_FACE ( 'NONE', ( #8025 ), #27584, .T. ) ;
#3460=CARTESIAN_POINT ( 'NONE',  ( -15.92677741484700071, 12.12620433921149399, 19.79423548914561692 ) ) ;
#3462=DIRECTION ( 'NONE',  ( 0.000000000000000000, 0.000000000000000000, 1.000000000000000000 ) ) ;
#3476=CARTESIAN_POINT ( 'NONE',  ( -3.662523238938586001, -12.47340865698848056, 1.500000000000001332 ) ) ;
#3477=ORIENTED_EDGE ( 'NONE', *, *, #25581, .T. ) ;
#3481=ORIENTED_EDGE ( 'NONE', *, *, #29812, .F. ) ;
#3484=EDGE_LOOP ( 'NONE', ( #27494, #3612, #15011, #16440 ) ) ;
#3487=CARTESIAN_POINT ( 'NONE',  ( 1.000000000000008438, 13.00000000000001421, 1.500000000000001332 ) ) ;
#3494=EDGE_CURVE ( 'NONE', #21278, #4066, #5448, .T. ) ;
#3495=CARTESIAN_POINT ( 'NONE',  ( -11.25351117620538943, -16.53363456493219630, 6.144783687052517429 ) ) ;
#3497=CARTESIAN_POINT ( 'NONE',  ( 11.99367014178016255, 12.13468339478709623, 20.19593175699879595 ) ) ;
#3501=AXIS2_PLACEMENT_3D ( 'NONE', #13064, #22553, #25054 ) ;
#3502=CARTESIAN_POINT ( 'NONE',  ( -9.011666854301582319, -14.45189732017202289, 20.19668224736330941 ) ) ;
#3505=CARTESIAN_POINT ( 'NONE',  ( -4.697473163530037077, 16.36296782919469806, 7.156916968540302904 ) ) ;
#3511=CARTESIAN_POINT ( 'NONE',  ( 14.88222593340885958, 13.36111339922579155, 7.652108011868850035 ) ) ;
#3513=CARTESIAN_POINT ( 'NONE',  ( -15.13937296497744356, 13.09668952202108905, 5.701226463332907279 ) ) ;
#3515=ORIENTED_EDGE ( 'NONE', *, *, #2115, .F. ) ;
#3518=CARTESIAN_POINT ( 'NONE',  ( 3.262081159888216675, 16.75658363656790328, 6.037360021877313798 ) ) ;
#3520=EDGE_CURVE ( 'NONE', #20845, #19924, #5128, .T. ) ;
#3522=DIRECTION ( 'NONE',  ( -0.000000000000000000, -0.000000000000000000, 1.000000000000000000 ) ) ;
#3524=FACE_OUTER_BOUND ( 'NONE', #10803, .T. ) ;
#3526=VERTEX_POINT ( 'NONE', #7325 ) ;
#3527=CARTESIAN_POINT ( 'NONE',  ( 11.83518757993566339, -16.12237520560631765, 6.149077423860702218 ) ) ;
#3529=CARTESIAN_POINT ( 'NONE',  ( -19.72722132040463094, 3.293256439147196790, 18.72886616302735163 ) ) ;
#3535=CIRCLE ( 'NONE', #10496, 1.000000000000004441 ) ;
#3536=CARTESIAN_POINT ( 'NONE',  ( -17.06581907267832321, 0.6464955982388042033, 6.521906765011496354 ) ) ;
#3537=CARTESIAN_POINT ( 'NONE',  ( 7.548823014270642950, -5.738360882149975417, 1.500000000000001332 ) ) ;
#3541=CARTESIAN_POINT ( 'NONE',  ( -8.661893131430954185, -14.67663382381789816, 20.34789198813115618 ) ) ;
#3545=CYLINDRICAL_SURFACE ( 'NONE', #26347, 0.7500000000000004441 ) ;
#3546=ORIENTED_EDGE ( 'NONE', *, *, #29235, .T. ) ;
#3549=ADVANCED_FACE ( 'NONE', ( #21815 ), #24829, .T. ) ;
#3552=CARTESIAN_POINT ( 'NONE',  ( -16.83923888061477925, 2.503175730361749896, 7.176035686813569292 ) ) ;
#3555=CARTESIAN_POINT ( 'NONE',  ( -8.579043560828049308, -14.72784502467622936, 18.34777357837151968 ) ) ;
#3557=VERTEX_POINT ( 'NONE', #13406 ) ;
#3558=FACE_OUTER_BOUND ( 'NONE', #4510, .T. ) ;
#3564=CARTESIAN_POINT ( 'NONE',  ( 19.68627777834516124, 3.628879393376895024, 7.559636331181775581 ) ) ;
#3566=CARTESIAN_POINT ( 'NONE',  ( 1.743352590880599795, -16.98718212385438520, 6.329955581934035180 ) ) ;
#3570=EDGE_LOOP ( 'NONE', ( #14317, #13434, #22569, #18053 ) ) ;
#3573=CARTESIAN_POINT ( 'NONE',  ( 10.31307689846358144, -13.59231953480259314, 18.50655187082627862 ) ) ;
#3574=AXIS2_PLACEMENT_3D ( 'NONE', #3838, #20518, #15205 ) ;
#3575=CARTESIAN_POINT ( 'NONE',  ( 0.7220001660362483920, 9.454746441592963180, 13.00000000000000178 ) ) ;
#3584=CARTESIAN_POINT ( 'NONE',  ( 6.262360769054548193, 18.99428434097457341, 6.781503518395073371 ) ) ;
#3585=ORIENTED_EDGE ( 'NONE', *, *, #24255, .F. ) ;
#3587=DIRECTION ( 'NONE',  ( 0.000000000000000000, 0.000000000000000000, -1.000000000000000000 ) ) ;
#3595=CIRCLE ( 'NONE', #10069, 1.000000000000007772 ) ;
#3596=ORIENTED_EDGE ( 'NONE', *, *, #7636, .F. ) ;
#3598=CARTESIAN_POINT ( 'NONE',  ( 3.146565092309296929, 16.78275473100424264, 6.233981582756856987 ) ) ;
#3600=CARTESIAN_POINT ( 'NONE',  ( 5.783356563690329466, 19.14595685992715346, 20.22277707861861984 ) ) ;
#3603=CARTESIAN_POINT ( 'NONE',  ( 10.83635815962788129, -16.83143582838889074, 18.39701043959520987 ) ) ;
#3608=CARTESIAN_POINT ( 'NONE',  ( 17.94577521512061580, -8.869393445417760091, 6.974106381145714018 ) ) ;
#3609=CARTESIAN_POINT ( 'NONE',  ( -15.70110224921265818, 12.41706793386162211, 18.50655187082627862 ) ) ;
#3610=LINE ( 'NONE', #17812, #3342 ) ;
#3611=EDGE_LOOP ( 'NONE', ( #18236, #15064, #11627, #15783 ) ) ;
#3612=ORIENTED_EDGE ( 'NONE', *, *, #4449, .F. ) ;
#3615=CARTESIAN_POINT ( 'NONE',  ( -4.596254364928607394, 16.38944764646977603, 19.56050940960062690 ) ) ;
#3618=EDGE_CURVE ( 'NONE', #26330, #27411, #29134, .T. ) ;
#3622=ORIENTED_EDGE ( 'NONE', *, *, #15918, .T. ) ;
#3623=AXIS2_PLACEMENT_3D ( 'NONE', #3476, #13145, #24840 ) ;
#3627=EDGE_LOOP ( 'NONE', ( #25027, #11175, #18096, #17252 ) ) ;
#3629=VECTOR ( 'NONE', #13122, 1000.000000000000000 ) ;
#3633=AXIS2_PLACEMENT_3D ( 'NONE', #26985, #5610, #15106 ) ;
#3645=CARTESIAN_POINT ( 'NONE',  ( 12.30878326772640996, 11.79452912058117242, 20.34789198813115263 ) ) ;
#3648=CARTESIAN_POINT ( 'NONE',  ( -10.98804681698542574, -16.73276138505788779, 20.19668224736330941 ) ) ;
#3649=CARTESIAN_POINT ( 'NONE',  ( -15.16517292768934944, -7.781889190071453299, 7.652108011868850035 ) ) ;
#3651=AXIS2_PLACEMENT_3D ( 'NONE', #19018, #4514, #14022 ) ;
#3652=CARTESIAN_POINT ( 'NONE',  ( 11.48757468322166808, -16.39371511241312618, 5.749491821935610147 ) ) ;
#3656=EDGE_LOOP ( 'NONE', ( #26090, #21109, #18977, #7393 ) ) ;
#3657=ORIENTED_EDGE ( 'NONE', *, *, #25723, .F. ) ;
#3663=CARTESIAN_POINT ( 'NONE',  ( -7.548823014270604759, 5.738360882150024267, 13.00000000000000178 ) ) ;
#3665=CARTESIAN_POINT ( 'NONE',  ( 3.113107691802094124, 16.79024107225297513, 6.329955581934033404 ) ) ;
#3667=CARTESIAN_POINT ( 'NONE',  ( -11.37681265597469960, -16.47072995046971755, 6.641371103590088865 ) ) ;
#3669=VERTEX_POINT ( 'NONE', #2284 ) ;
#3670=ADVANCED_FACE ( 'NONE', ( #25857 ), #4027, .F. ) ;
#3671=B_SPLINE_SURFACE_WITH_KNOTS ( 'NONE', 3, 1, ( 
 ( #4653, #7614 ),
 ( #7467, #24129 ),
 ( #21483, #19310 ),
 ( #7305, #4797 ),
 ( #6995, #21330 ),
 ( #14776, #16966 ),
 ( #14309, #2781 ),
 ( #23825, #2474 ),
 ( #14473, #11990 ),
 ( #30846, #16817 ),
 ( #28522, #24295 ),
 ( #7153, #12295 ),
 ( #125, #19007 ),
 ( #581, #12142 ),
 ( #439, #23975 ),
 ( #9491, #16664 ),
 ( #10101, #2945 ),
 ( #23660, #28373 ),
 ( #19157, #4964 ),
 ( #16507, #2622 ),
 ( #21643, #14156 ),
 ( #278, #9797 ),
 ( #28830, #21800 ),
 ( #26485, #9955 ),
 ( #19463, #13075 ),
 ( #27105, #899 ),
 ( #10570, #1366 ),
 ( #22102, #29291 ),
 ( #5434, #29599 ),
 ( #5890, #26961 ),
 ( #29748, #27257 ) ),
 .UNSPECIFIED., .F., .F., .F.,
 ( 4, 3, 3, 3, 3, 3, 3, 3, 3, 3, 4 ),
 ( 2, 2 ),
 ( 0.4999999998345686647, 0.5360336730431939367, 0.5907651151589012883, 0.6456034593241830599, 0.6998270958050434309, 0.7529536536315937223, 0.8052385063053260073, 0.8575343587103997356, 0.9106564858195042023, 0.9648414833209685293, 1.000000006602610236 ),
 ( 0.000000000000000000, 1.000000000000000000 ),
 .UNSPECIFIED. ) ;
#3672=VECTOR ( 'NONE', #12552, 1000.000000000000000 ) ;
#3674=CARTESIAN_POINT ( 'NONE',  ( 19.59831178344208169, 3.989367808977733354, 19.96797677718664232 ) ) ;
#3675=ORIENTED_EDGE ( 'NONE', *, *, #6937, .F. ) ;
#3676=ADVANCED_FACE ( 'NONE', ( #13701 ), #20857, .F. ) ;
#3683=FACE_OUTER_BOUND ( 'NONE', #7046, .T. ) ;
#3684=ORIENTED_EDGE ( 'NONE', *, *, #13760, .F. ) ;
#3685=CARTESIAN_POINT ( 'NONE',  ( 12.35846533491530685, 11.73919094685904341, 20.34789198813115263 ) ) ;
#3687=CARTESIAN_POINT ( 'NONE',  ( -8.546423435383420752, -14.74799740001550141, 5.652196082368483587 ) ) ;
#3692=CARTESIAN_POINT ( 'NONE',  ( 9.999999999999959144, 1.510243460696181139E-14, 24.50000000000000000 ) ) ;
#3693=CARTESIAN_POINT ( 'NONE',  ( 19.81789086666767119, 2.695592600026630148, 5.775318986477952166 ) ) ;
#3696=EDGE_LOOP ( 'NONE', ( #28129, #2459, #12691, #30638 ) ) ;
#3697=VERTEX_POINT ( 'NONE', #18532 ) ;
#3700=FACE_OUTER_BOUND ( 'NONE', #830, .T. ) ;
#3710=ORIENTED_EDGE ( 'NONE', *, *, #24779, .F. ) ;
#3712=CARTESIAN_POINT ( 'NONE',  ( -19.78525473782456601, 3.044038662852082133, 7.500898271101006820 ) ) ;
#3713=CARTESIAN_POINT ( 'NONE',  ( 16.61573067466906650, 3.902325345048615279, 20.06253562465620632 ) ) ;
#3714=DIRECTION ( 'NONE',  ( 1.000000000000000000, 0.000000000000000000, 0.000000000000000000 ) ) ;
#3716=ORIENTED_EDGE ( 'NONE', *, *, #26503, .F. ) ;
#3717=CARTESIAN_POINT ( 'NONE',  ( -5.393256883115301825, -14.81828060999315433, -0.6213203435596476032 ) ) ;
#3723=CARTESIAN_POINT ( 'NONE',  ( -15.34618031767423041, 12.82553819247484128, 18.34798005863227388 ) ) ;
#3724=DIRECTION ( 'NONE',  ( -0.000000000000000000, -0.000000000000000000, 1.000000000000000000 ) ) ;
#3725=CARTESIAN_POINT ( 'NONE',  ( 19.68435877536853340, 3.639270104310704745, 5.749491821935610147 ) ) ;
#3727=CARTESIAN_POINT ( 'NONE',  ( -10.33762405876901980, -17.14187335405549462, 20.32367522806703874 ) ) ;
#3729=DIRECTION ( 'NONE',  ( 1.000000000000000000, 0.000000000000000000, 0.000000000000000000 ) ) ;
#3731=ORIENTED_EDGE ( 'NONE', *, *, #21200, .F. ) ;
#3736=ORIENTED_EDGE ( 'NONE', *, *, #15617, .T. ) ;
#3740=CARTESIAN_POINT ( 'NONE',  ( -5.369726540290508332, 19.28438192063506307, 5.862424720655265098 ) ) ;
#3747=CARTESIAN_POINT ( 'NONE',  ( 14.45824965121216010, 13.84471048730597786, 5.872146474157316831 ) ) ;
#3749=ORIENTED_EDGE ( 'NONE', *, *, #15480, .T. ) ;
#3755=CARTESIAN_POINT ( 'NONE',  ( 3.200917658998827964, 16.77053181957578332, 6.131018562779544823 ) ) ;
#3760=VECTOR ( 'NONE', #9073, 1000.000000000000227 ) ;
#3762=CARTESIAN_POINT ( 'NONE',  ( 9.833055564703260032, -13.92194044488497084, 18.34777357837152323 ) ) ;
#3763=CARTESIAN_POINT ( 'NONE',  ( 16.82340201860977302, 2.653416696629038007, 20.19668224736330941 ) ) ;
#3764=VERTEX_POINT ( 'NONE', #18393 ) ;
#3766=CARTESIAN_POINT ( 'NONE',  ( 15.38930515692759471, -7.273136567754737491, 6.530762810602277924 ) ) ;
#3768=CARTESIAN_POINT ( 'NONE',  ( -15.95709955354364418, 12.08619843917606929, 6.341840715582230281 ) ) ;
#3769=CARTESIAN_POINT ( 'NONE',  ( 4.414161002286802749, 19.52491365267160361, 19.79423548914561692 ) ) ;
#3771=VERTEX_POINT ( 'NONE', #26626 ) ;
#3774=CARTESIAN_POINT ( 'NONE',  ( -2.703030265324078307, -12.75514121382991384, 1.500000000000001332 ) ) ;
#3778=CARTESIAN_POINT ( 'NONE',  ( 1.000000000000008438, 16.48749217771910125, -0.6213203435596476032 ) ) ;
#3780=ORIENTED_EDGE ( 'NONE', *, *, #9565, .T. ) ;
#3782=LINE ( 'NONE', #27643, #27161 ) ;
#3783=FACE_OUTER_BOUND ( 'NONE', #27772, .T. ) ;
#3784=ORIENTED_EDGE ( 'NONE', *, *, #21200, .T. ) ;
#3785=CIRCLE ( 'NONE', #21176, 0.7499999999999988898 ) ;
#3786=ORIENTED_EDGE ( 'NONE', *, *, #28796, .F. ) ;
#3787=CARTESIAN_POINT ( 'NONE',  ( 9.590471615930072247, -1.687027447297460236, 21.50000000000000000 ) ) ;
#3793=DIRECTION ( 'NONE',  ( 1.000000000000000000, 0.000000000000000000, 0.000000000000000000 ) ) ;
#3798=CARTESIAN_POINT ( 'NONE',  ( 1.350727940147186112, -19.97202376558938752, 6.447548852708279377 ) ) ;
#3800=CARTESIAN_POINT ( 'NONE',  ( -10.97902775627723670, -16.73874854128740353, 18.49267272388512140 ) ) ;
#3802=CARTESIAN_POINT ( 'NONE',  ( -4.573988094335657451, 16.39521158297133141, 6.714907520933424578 ) ) ;
#3804=CARTESIAN_POINT ( 'NONE',  ( 11.23845335764779385, -16.56542118924665630, 7.643931100913408550 ) ) ;
#3815=FACE_OUTER_BOUND ( 'NONE', #29238, .T. ) ;
#3818=CARTESIAN_POINT ( 'NONE',  ( -10.52280129341197323, -17.02885805942690567, 5.652196082367002994 ) ) ;
#3819=AXIS2_PLACEMENT_3D ( 'NONE', #20597, #22942, #1731 ) ;
#3823=VERTEX_POINT ( 'NONE', #7752 ) ;
#3825=VECTOR ( 'NONE', #7196, 1000.000000000000000 ) ;
#3827=CIRCLE ( 'NONE', #13302, 20.00000000000000000 ) ;
#3828=CARTESIAN_POINT ( 'NONE',  ( -15.16517293421788537, -7.781889191988407006, 20.34789198813115263 ) ) ;
#3832=CARTESIAN_POINT ( 'NONE',  ( 12.88533868971568808, 11.12831076058098745, 19.96344307082653202 ) ) ;
#3833=ADVANCED_FACE ( 'NONE', ( #12590 ), #23803, .F. ) ;
#3834=CARTESIAN_POINT ( 'NONE',  ( 0.4897477184365084391, -19.99444548460946791, 18.34869673959212122 ) ) ;
#3836=CARTESIAN_POINT ( 'NONE',  ( -17.06384985643477847, 0.6725948717588426939, 6.392658652357120275 ) ) ;
#3838=CARTESIAN_POINT ( 'NONE',  ( 5.881244434206234217, 6.812559277181991391, 1.500000000000001332 ) ) ;
#3840=DIRECTION ( 'NONE',  ( -0.000000000000000000, -0.000000000000000000, 1.000000000000000000 ) ) ;
#3842=CARTESIAN_POINT ( 'NONE',  ( 9.117173258182925011, -14.37672153453698343, 7.156916968540298463 ) ) ;
#3843=FACE_OUTER_BOUND ( 'NONE', #8490, .T. ) ;
#3844=CARTESIAN_POINT ( 'NONE',  ( -9.228184491520634580, -14.30775539779752847, 19.96344307082651781 ) ) ;
#3845=AXIS2_PLACEMENT_3D ( 'NONE', #29030, #10152, #7667 ) ;
#3852=ORIENTED_EDGE ( 'NONE', *, *, #5782, .F. ) ;
#3853=CARTESIAN_POINT ( 'NONE',  ( 9.169883732660084164, -9.268939115642975679, 1.500000000000001332 ) ) ;
#3854=EDGE_CURVE ( 'NONE', #13757, #21278, #24113, .T. ) ;
#3855=CARTESIAN_POINT ( 'NONE',  ( 9.117173258235231614, -14.37672153450547619, 19.85270094495842130 ) ) ;
#3856=EDGE_CURVE ( 'NONE', #23663, #21250, #2763, .T. ) ;
#3860=CARTESIAN_POINT ( 'NONE',  ( -16.81737828845396265, 2.629481162813160022, 6.420335371522007506 ) ) ;
#3863=AXIS2_PLACEMENT_3D ( 'NONE', #9359, #8436, #9821 ) ;
#3864=CARTESIAN_POINT ( 'NONE',  ( 15.52007383991470135, 12.61466978257045746, 6.386539667786101937 ) ) ;
#3868=ORIENTED_EDGE ( 'NONE', *, *, #1967, .F. ) ;
#3870=CARTESIAN_POINT ( 'NONE',  ( -14.93254240672194122, -8.254432589262984621, 7.545655578832112909 ) ) ;
#3871=CARTESIAN_POINT ( 'NONE',  ( -16.87879800891222359, 2.262652451654310060, 18.54473042795394733 ) ) ;
#3872=AXIS2_PLACEMENT_3D ( 'NONE', #18899, #11257, #11880 ) ;
#3876=CARTESIAN_POINT ( 'NONE',  ( -6.910239377218535317, 18.76835738875811899, 19.08830981656263859 ) ) ;
#3879=CARTESIAN_POINT ( 'NONE',  ( 19.64806919293054932, 3.830191698062872074, 5.872146474157316831 ) ) ;
#3882=CARTESIAN_POINT ( 'NONE',  ( -9.736160311572513493, -17.49040459468425368, 19.79423548914561692 ) ) ;
#3884=CARTESIAN_POINT ( 'NONE',  ( -17.02601880987613825, 1.106972870283159160, 18.50655187082627862 ) ) ;
#3886=ORIENTED_EDGE ( 'NONE', *, *, #15278, .T. ) ;
#3895=CARTESIAN_POINT ( 'NONE',  ( -15.51517975927889736, 12.62116967784147548, 5.679672709359370408 ) ) ;
#3896=ADVANCED_FACE ( 'NONE', ( #5100 ), #9935, .F. ) ;
#3900=AXIS2_PLACEMENT_3D ( 'NONE', #250, #16941, #19584 ) ;
#3901=CARTESIAN_POINT ( 'NONE',  ( -12.85122823565992789, 11.16779817455389434, 6.031926333436658183 ) ) ;
#3905=LINE ( 'NONE', #11674, #2799 ) ;
#3908=DIRECTION ( 'NONE',  ( 1.000000000000000000, 0.000000000000000000, 0.000000000000000000 ) ) ;
#3910=VECTOR ( 'NONE', #17305, 1000.000000000000000 ) ;
#3918=B_SPLINE_CURVE_WITH_KNOTS ( 'NONE', 3,
 ( #25303, #13904, #23406, #3948, #25906, #30129, #30581, #11422, #20911, #30434, #20753, #9220, #9074, #8759, #6877, #4536, #23868, #476 ),
 .UNSPECIFIED., .F., .F.,
 ( 4, 2, 2, 2, 2, 2, 2, 2, 4 ),
 ( 0.003174295595554312618, 0.003570702171545547116, 0.003967108747536782047, 0.004363515323528016111, 0.004759921899519251043, 0.005156328475510485107, 0.005552735051501720039, 0.005949141627492954970, 0.006345548203484189034 ),
 .UNSPECIFIED. ) ;
#3919=CARTESIAN_POINT ( 'NONE',  ( 4.400293182487617472, 19.52803631353506120, 6.233981582756856987 ) ) ;
#3920=DIRECTION ( 'NONE',  ( 0.000000000000000000, 0.000000000000000000, 1.000000000000000000 ) ) ;
#3921=DIRECTION ( 'NONE',  ( -0.000000000000000000, -0.000000000000000000, 1.000000000000000000 ) ) ;
#3922=EDGE_LOOP ( 'NONE', ( #19589, #4316, #17440, #28748 ) ) ;
#3925=CARTESIAN_POINT ( 'NONE',  ( 11.02326084422093011, -16.70928013427648295, 18.35377592296120497 ) ) ;
#3926=CARTESIAN_POINT ( 'NONE',  ( 19.87340826026480656, 2.401441585233817566, 19.96783386855779341 ) ) ;
#3928=CARTESIAN_POINT ( 'NONE',  ( 14.88222593340886668, 13.36111339922579866, 20.34789198813115263 ) ) ;
#3929=CARTESIAN_POINT ( 'NONE',  ( 17.92822150912323664, -8.904799031605449500, 6.530762810602277924 ) ) ;
#3930=CARTESIAN_POINT ( 'NONE',  ( -13.72472375636738029, 10.13620556525982330, 5.810767894563978686 ) ) ;
#3931=CARTESIAN_POINT ( 'NONE',  ( 4.045241160498761701, 16.55840174588940528, 18.34798005862662507 ) ) ;
#3933=ORIENTED_EDGE ( 'NONE', *, *, #19011, .T. ) ;
#3936=CARTESIAN_POINT ( 'NONE',  ( 10.29553672503491057, -13.60582241699094119, 7.545655578832112020 ) ) ;
#3938=CARTESIAN_POINT ( 'NONE',  ( -5.002692087210951932, 19.38273059899790951, 19.45164628100866722 ) ) ;
#3941=CARTESIAN_POINT ( 'NONE',  ( 0.000000000000000000, 0.000000000000000000, 1.500000000000001332 ) ) ;
#3942=CARTESIAN_POINT ( 'NONE',  ( 1.000000000000008438, 16.48749217771910125, -0.6213203435596476032 ) ) ;
#3945=DIRECTION ( 'NONE',  ( 0.000000000000000000, 0.000000000000000000, 1.000000000000000000 ) ) ;
#3948=CARTESIAN_POINT ( 'NONE',  ( 19.81826808356699132, 2.692791747024146254, 20.22277707861861273 ) ) ;
#3955=ORIENTED_EDGE ( 'NONE', *, *, #2747, .T. ) ;
#3956=CARTESIAN_POINT ( 'NONE',  ( -0.5297379638125898627, -19.99304770284714650, 7.156831654632817674 ) ) ;
#3959=DIRECTION ( 'NONE',  ( 0.000000000000000000, 0.000000000000000000, -1.000000000000000000 ) ) ;
#3963=CARTESIAN_POINT ( 'NONE',  ( 1.363408835038997236, -19.97112866468681602, 6.782048567692550378 ) ) ;
#3966=CARTESIAN_POINT ( 'NONE',  ( 0.000000000000000000, 0.000000000000000000, 1.500000000000001332 ) ) ;
#3968=CARTESIAN_POINT ( 'NONE',  ( -17.77309463542033541, -9.210542792609437868, 18.56793045041961321 ) ) ;
#3975=CARTESIAN_POINT ( 'NONE',  ( -6.102995743689038299, 19.04655207687856944, 5.652912763329821288 ) ) ;
#3981=ORIENTED_EDGE ( 'NONE', *, *, #21808, .F. ) ;
#3984=ORIENTED_EDGE ( 'NONE', *, *, #18723, .T. ) ;
#3987=CYLINDRICAL_SURFACE ( 'NONE', #17331, 0.7500000000000006661 ) ;
#3988=CARTESIAN_POINT ( 'NONE',  ( 0.4302108320067679070, -20.01327865860580602, 18.34838970509067479 ) ) ;
#3990=CARTESIAN_POINT ( 'NONE',  ( 11.69640250238807333, 12.44177653180062748, 19.02573955821369012 ) ) ;
#3993=CARTESIAN_POINT ( 'NONE',  ( -15.42380629414487991, -7.219239307198620281, 20.14907003336613300 ) ) ;
#3997=CARTESIAN_POINT ( 'NONE',  ( 19.74251403343738076, 3.198927889078825970, 5.652196082369965069 ) ) ;
#3998=CARTESIAN_POINT ( 'NONE',  ( -9.372686588590493528, -14.20906563288477997, 19.08155846658118548 ) ) ;
#3999=ORIENTED_EDGE ( 'NONE', *, *, #30693, .F. ) ;
#4000=ORIENTED_EDGE ( 'NONE', *, *, #24041, .F. ) ;
#4004=ORIENTED_EDGE ( 'NONE', *, *, #2534, .F. ) ;
#4008=CARTESIAN_POINT ( 'NONE',  ( 9.051788058555931826, -14.41610800088323252, 19.66962785902261857 ) ) ;
#4011=CARTESIAN_POINT ( 'NONE',  ( -10.62409560796092833, -16.94539057243558489, 18.34726407865098707 ) ) ;
#4013=DIRECTION ( 'NONE',  ( -0.000000000000000000, -0.000000000000000000, 1.000000000000000000 ) ) ;
#4020=FACE_OUTER_BOUND ( 'NONE', #26751, .T. ) ;
#4023=VERTEX_POINT ( 'NONE', #7595 ) ;
#4024=CARTESIAN_POINT ( 'NONE',  ( 0.000000000000000000, 0.000000000000000000, 1.500000000000001332 ) ) ;
#4026=EDGE_CURVE ( 'NONE', #24952, #26662, #8650, .T. ) ;
#4027=CYLINDRICAL_SURFACE ( 'NONE', #17745, 0.7500000000000006661 ) ;
#4028=EDGE_CURVE ( 'NONE', #13391, #8694, #14252, .T. ) ;
#4030=CARTESIAN_POINT ( 'NONE',  ( -8.546423435383420752, -14.74799740001550141, 5.652196082368483587 ) ) ;
#4032=CARTESIAN_POINT ( 'NONE',  ( 11.18191171624325797, -16.60365183919260090, 18.34838970509067479 ) ) ;
#4034=ORIENTED_EDGE ( 'NONE', *, *, #21197, .F. ) ;
#4036=DIRECTION ( 'NONE',  ( 1.000000000000000000, 0.000000000000000000, 0.000000000000000000 ) ) ;
#4039=ORIENTED_EDGE ( 'NONE', *, *, #16675, .F. ) ;
#4040=DIRECTION ( 'NONE',  ( -1.000000000000000000, 0.000000000000000000, 0.000000000000000000 ) ) ;
#4043=ADVANCED_FACE ( 'NONE', ( #5561 ), #20515, .F. ) ;
#4047=DIRECTION ( 'NONE',  ( 0.000000000000000000, 0.000000000000000000, -1.000000000000000000 ) ) ;
#4050=ORIENTED_EDGE ( 'NONE', *, *, #21197, .T. ) ;
#4053=CARTESIAN_POINT ( 'NONE',  ( -6.974883619896829146, -5.687793815610328707, 1.500000000000001332 ) ) ;
#4055=ORIENTED_EDGE ( 'NONE', *, *, #21799, .T. ) ;
#4060=CARTESIAN_POINT ( 'NONE',  ( -0.4564504349075055867, 9.471281197126600659, 21.50000000000000000 ) ) ;
#4061=ORIENTED_EDGE ( 'NONE', *, *, #17013, .T. ) ;
#4064=FACE_OUTER_BOUND ( 'NONE', #9660, .T. ) ;
#4066=VERTEX_POINT ( 'NONE', #15678 ) ;
#4067=CARTESIAN_POINT ( 'NONE',  ( -16.90489691178405707, 2.092419235659072729, 20.25336174263950184 ) ) ;
#4069=CARTESIAN_POINT ( 'NONE',  ( -15.57270467870638342, 12.57827228024023825, 5.704143890883081269 ) ) ;
#4070=CARTESIAN_POINT ( 'NONE',  ( 3.623302445573593378, 16.66947753447049152, 20.25542030744407640 ) ) ;
#4071=VERTEX_POINT ( 'NONE', #24730 ) ;
#4076=CARTESIAN_POINT ( 'NONE',  ( -4.626122995383912695, 16.38173570853529881, 19.00652017443069752 ) ) ;
#4086=CARTESIAN_POINT ( 'NONE',  ( 1.239979252855709868, -19.96159058730291136, 6.149077423860696001 ) ) ;
#4087=DIRECTION ( 'NONE',  ( -0.000000000000000000, -0.000000000000000000, 1.000000000000000000 ) ) ;
#4089=ORIENTED_EDGE ( 'NONE', *, *, #130, .F. ) ;
#4092=CARTESIAN_POINT ( 'NONE',  ( 2.094186647214743235, -9.248129367672072831, 13.00000000000000178 ) ) ;
#4093=CARTESIAN_POINT ( 'NONE',  ( -19.94291556179616265, 1.510882595598286970, 19.08830981656264214 ) ) ;
#4095=DIRECTION ( 'NONE',  ( 1.000000000000000000, 0.000000000000000000, 0.000000000000000000 ) ) ;
#4102=CARTESIAN_POINT ( 'NONE',  ( -16.84890868873869607, 2.447051129653413870, 6.031926333436659071 ) ) ;
#4109=CARTESIAN_POINT ( 'NONE',  ( -17.86170306354901527, -9.037578821739913337, 18.44527579819791185 ) ) ;
#4110=EDGE_CURVE ( 'NONE', #19511, #20108, #9346, .T. ) ;
#4112=EDGE_CURVE ( 'NONE', #14448, #4543, #20664, .T. ) ;
#4114=ORIENTED_EDGE ( 'NONE', *, *, #249, .F. ) ;
#4115=CARTESIAN_POINT ( 'NONE',  ( -0.4522595252855764469, -19.99510590919687303, 18.72886616302735519 ) ) ;
#4116=AXIS2_PLACEMENT_3D ( 'NONE', #10753, #20264, #29789 ) ;
#4119=CARTESIAN_POINT ( 'NONE',  ( -2.555255504830902691, 9.131494062835640690, 13.00000000000000178 ) ) ;
#4130=FACE_OUTER_BOUND ( 'NONE', #14028, .T. ) ;
#4131=CARTESIAN_POINT ( 'NONE',  ( 0.5064538767941890729, -20.01148730445866164, 18.35718225375110180 ) ) ;
#4133=CARTESIAN_POINT ( 'NONE',  ( 11.65964093050817674, 12.47882650181266051, 19.28454053338348828 ) ) ;
#4134=AXIS2_PLACEMENT_3D ( 'NONE', #29072, #5984, #5366 ) ;
#4139=CARTESIAN_POINT ( 'NONE',  ( -15.52715705409945457, -6.980092275558532400, 18.83976166372255179 ) ) ;
#4142=DIRECTION ( 'NONE',  ( 0.000000000000000000, 0.000000000000000000, 1.000000000000000000 ) ) ;
#4143=CARTESIAN_POINT ( 'NONE',  ( -18.04156136322730219, -8.631457789788591128, 18.34798005863226678 ) ) ;
#4146=EDGE_LOOP ( 'NONE', ( #11075, #24133, #28915, #1546 ) ) ;
#4157=VERTEX_POINT ( 'NONE', #23315 ) ;
#4160=DIRECTION ( 'NONE',  ( 0.000000000000000000, 0.000000000000000000, 1.000000000000000000 ) ) ;
#4161=CARTESIAN_POINT ( 'NONE',  ( 12.72536390617885438, -2.839914339433650348, 1.500000000000001332 ) ) ;
#4166=CARTESIAN_POINT ( 'NONE',  ( -14.93932203929706759, 13.29757777824904075, 7.454139397117721444 ) ) ;
#4167=ORIENTED_EDGE ( 'NONE', *, *, #29989, .T. ) ;
#4170=CARTESIAN_POINT ( 'NONE',  ( 19.73705937795079279, 3.341332093703274442, 7.643931100913408550 ) ) ;
#4173=CARTESIAN_POINT ( 'NONE',  ( -16.99844672493304998, 1.385815296451945899, 18.34938820207544907 ) ) ;
#4175=CARTESIAN_POINT ( 'NONE',  ( -9.395142731145654125, -14.19351217900082496, 6.519181285484530797 ) ) ;
#4183=EDGE_CURVE ( 'NONE', #5874, #10035, #5818, .T. ) ;
#4184=LINE ( 'NONE', #8426, #26587 ) ;
#4188=CARTESIAN_POINT ( 'NONE',  ( -12.73056545647080640, 11.29944703098672854, 6.385774490351133537 ) ) ;
#4190=ORIENTED_EDGE ( 'NONE', *, *, #25406, .F. ) ;
#4192=CARTESIAN_POINT ( 'NONE',  ( -18.04156136322730219, -8.631457789788591128, 18.34798005863226678 ) ) ;
#4197=EDGE_LOOP ( 'NONE', ( #27838, #16737, #25976, #14993 ) ) ;
#4206=CARTESIAN_POINT ( 'NONE',  ( 16.80963242778062749, 2.754998275627143389, 20.25336174263950184 ) ) ;
#4209=EDGE_CURVE ( 'NONE', #25701, #23663, #9125, .T. ) ;
#4210=CARTESIAN_POINT ( 'NONE',  ( -16.88948989945504309, 2.193765388987376497, 20.19668224736330941 ) ) ;
#4211=CARTESIAN_POINT ( 'NONE',  ( 18.09058649146511044, -8.570415951004783039, 5.862424720655265098 ) ) ;
#4212=CARTESIAN_POINT ( 'NONE',  ( -15.90168156411149170, 12.15925017959999188, 6.131018562779544823 ) ) ;
#4213=CARTESIAN_POINT ( 'NONE',  ( 3.200917658998823967, 16.77053181957577621, 18.82680253904184298 ) ) ;
#4215=ORIENTED_EDGE ( 'NONE', *, *, #28347, .T. ) ;
#4220=CARTESIAN_POINT ( 'NONE',  ( -5.222323004038176286, 16.21609733491350980, 20.29090034784956131 ) ) ;
#4221=CARTESIAN_POINT ( 'NONE',  ( 11.68275852896170619, 12.45554129447766378, 6.392658652357122939 ) ) ;
#4224=EDGE_CURVE ( 'NONE', #27607, #29319, #11944, .T. ) ;
#4226=CARTESIAN_POINT ( 'NONE',  ( -17.06612199394663421, 0.6423840055640266389, 6.782048567692550378 ) ) ;
#4231=EDGE_CURVE ( 'NONE', #30675, #20736, #20734, .T. ) ;
#4234=CARTESIAN_POINT ( 'NONE',  ( 18.38343463818524626, -7.922482876633606175, 5.652605728828373977 ) ) ;
#4236=ORIENTED_EDGE ( 'NONE', *, *, #14115, .T. ) ;
#4237=DIRECTION ( 'NONE',  ( -0.000000000000000000, -0.000000000000000000, 1.000000000000000000 ) ) ;
#4245=EDGE_CURVE ( 'NONE', #24485, #20446, #30795, .T. ) ;
#4249=FACE_OUTER_BOUND ( 'NONE', #6363, .T. ) ;
#4251=CYLINDRICAL_SURFACE ( 'NONE', #22007, 9.482273699623480212 ) ;
#4252=CARTESIAN_POINT ( 'NONE',  ( -17.81743587613174284, -9.123988531026231641, 18.50655187082627862 ) ) ;
#4257=CARTESIAN_POINT ( 'NONE',  ( -0.2646837113541511410, -19.99846847964001384, 18.54479204710283469 ) ) ;
#4266=LINE ( 'NONE', #1640, #23887 ) ;
#4271=ADVANCED_FACE ( 'NONE', ( #220 ), #25079, .T. ) ;
#4272=CARTESIAN_POINT ( 'NONE',  ( -10.05618025891931389, -17.30842068227156361, 5.810767894563978686 ) ) ;
#4276=VERTEX_POINT ( 'NONE', #10200 ) ;
#4284=CARTESIAN_POINT ( 'NONE',  ( -15.56680656381426786, -6.886169722883741962, 19.08155846658118904 ) ) ;
#4286=DIRECTION ( 'NONE',  ( -0.000000000000000000, -0.000000000000000000, 1.000000000000000000 ) ) ;
#4287=CARTESIAN_POINT ( 'NONE',  ( 3.794966104483022296, 16.62713903700563378, 20.34789198813115263 ) ) ;
#4289=FACE_OUTER_BOUND ( 'NONE', #22147, .T. ) ;
#4299=CARTESIAN_POINT ( 'NONE',  ( 18.35115206909799923, -7.996681782469499566, 20.34789198813115263 ) ) ;
#4300=CARTESIAN_POINT ( 'NONE',  ( 5.372849316406058229, 19.28330981562107027, 5.653912893140659257 ) ) ;
#4301=AXIS2_PLACEMENT_3D ( 'NONE', #1613, #27653, #25148 ) ;
#4303=CARTESIAN_POINT ( 'NONE',  ( -19.84673203616234716, 2.611426761413839781, 5.657991946698900598 ) ) ;
#4309=ORIENTED_EDGE ( 'NONE', *, *, #23142, .F. ) ;
#4312=CARTESIAN_POINT ( 'NONE',  ( -8.072557715923444732, 14.41080185948837311, -0.6213203435596476032 ) ) ;
#4314=EDGE_CURVE ( 'NONE', #30397, #21299, #27759, .T. ) ;
#4316=ORIENTED_EDGE ( 'NONE', *, *, #24326, .F. ) ;
#4319=CARTESIAN_POINT ( 'NONE',  ( 4.049916833591939103, 16.55712665779026693, 20.34789198813115263 ) ) ;
#4320=DIRECTION ( 'NONE',  ( -0.4154150130018864351, 0.9096319953545184411, 0.000000000000000000 ) ) ;
#4322=CARTESIAN_POINT ( 'NONE',  ( -0.6368756358441494125, -20.00777098345651339, 6.864725433338323413 ) ) ;
#4326=DIRECTION ( 'NONE',  ( -1.000000000000000000, 0.000000000000000000, 0.000000000000000000 ) ) ;
#4327=CARTESIAN_POINT ( 'NONE',  ( -17.05413688332568256, 0.7966627085705066946, 19.89182036555910571 ) ) ;
#4328=CARTESIAN_POINT ( 'NONE',  ( -4.163336342344337027E-14, 1.387778780781445676E-14, 24.50000000000000000 ) ) ;
#4331=CARTESIAN_POINT ( 'NONE',  ( 10.69412491129097553, -13.31565357151864859, 19.25672174529527325 ) ) ;
#4351=ORIENTED_EDGE ( 'NONE', *, *, #10466, .T. ) ;
#4355=CARTESIAN_POINT ( 'NONE',  ( 0.5197766397930339011, -17.03069205084988269, 18.37259980046033903 ) ) ;
#4356=AXIS2_PLACEMENT_3D ( 'NONE', #16520, #23385, #2322 ) ;
#4357=VECTOR ( 'NONE', #15370, 1000.000000000000000 ) ;
#4366=VECTOR ( 'NONE', #11189, 1000.000000000000114 ) ;
#4368=CARTESIAN_POINT ( 'NONE',  ( 3.826954525806321339, 16.61697297626111336, 18.37415474056476938 ) ) ;
#4370=ORIENTED_EDGE ( 'NONE', *, *, #15083, .F. ) ;
#4371=AXIS2_PLACEMENT_3D ( 'NONE', #25035, #12733, #24892 ) ;
#4373=CARTESIAN_POINT ( 'NONE',  ( 10.52757208841436309, -13.43854510675287983, 6.037360021877314686 ) ) ;
#4374=DIRECTION ( 'NONE',  ( 0.000000000000000000, 0.000000000000000000, -1.000000000000000000 ) ) ;
#4377=B_SPLINE_CURVE_WITH_KNOTS ( 'NONE', 3,
 ( #23766, #14427, #24231, #7097, #24080, #17221, #2730, #28930, #11771, #16919, #2419, #379, #28619, #9592, #14248, #19103, #530, #12091 ),
 .UNSPECIFIED., .F., .F.,
 ( 4, 2, 2, 2, 2, 2, 2, 2, 4 ),
 ( 0.000000000000000000, 0.0003967869494442860957, 0.0007935738988885721913, 0.001190360848332858287, 0.001587147797777144383, 0.001983934747221430261, 0.002380721696665716574, 0.002777508646110002886, 0.003174295595554288765 ),
 .UNSPECIFIED. ) ;
#4382=CARTESIAN_POINT ( 'NONE',  ( -19.91121867491064279, 2.064381093144387780, 7.559636331181775581 ) ) ;
#4384=CARTESIAN_POINT ( 'NONE',  ( 14.27661992934219626, 14.00645734016342736, 19.85730954408916915 ) ) ;
#4391=VECTOR ( 'NONE', #7705, 1000.000000000000227 ) ;
#4392=CARTESIAN_POINT ( 'NONE',  ( 0.000000000000000000, 0.000000000000000000, 1.500000000000001332 ) ) ;
#4396=CARTESIAN_POINT ( 'NONE',  ( -19.62935297797563905, -3.832558109936532009, 24.50000000000000000 ) ) ;
#4400=CARTESIAN_POINT ( 'NONE',  ( -6.294089901980526314, 15.86740633010675161, 19.97651184436794125 ) ) ;
#4403=ORIENTED_EDGE ( 'NONE', *, *, #7857, .F. ) ;
#4413=CARTESIAN_POINT ( 'NONE',  ( -14.72704883620385630, -8.644027383692558075, 19.03762469184452755 ) ) ;
#4417=VERTEX_POINT ( 'NONE', #18758 ) ;
#4418=DIRECTION ( 'NONE',  ( -1.000000000000000000, 0.000000000000000000, 0.000000000000000000 ) ) ;
#4421=CARTESIAN_POINT ( 'NONE',  ( -6.737892368765494133, 18.83108299337147784, 7.272192800924337952 ) ) ;
#4422=ORIENTED_EDGE ( 'NONE', *, *, #1182, .F. ) ;
#4427=ADVANCED_FACE ( 'NONE', ( #4249 ), #6903, .F. ) ;
#4435=CARTESIAN_POINT ( 'NONE',  ( 16.55527708515955609, 4.194179076328807376, 19.28454053338348473 ) ) ;
#4439=CARTESIAN_POINT ( 'NONE',  ( -8.361245565923718814, -14.86101098545373489, 7.627891251804737927 ) ) ;
#4442=CARTESIAN_POINT ( 'NONE',  ( 0.8870900849372836960, -19.99803318816115549, 20.19593175699879595 ) ) ;
#4446=CARTESIAN_POINT ( 'NONE',  ( 12.53055695656588497, 11.54555247029844800, 18.37259980046034613 ) ) ;
#4449=EDGE_CURVE ( 'NONE', #21250, #27848, #15964, .T. ) ;
#4452=AXIS2_PLACEMENT_3D ( 'NONE', #20719, #27769, #15916 ) ;
#4454=CARTESIAN_POINT ( 'NONE',  ( -12.73345385815705555, 11.29622791819166494, 19.60617949693493500 ) ) ;
#4455=DIRECTION ( 'NONE',  ( 0.000000000000000000, 0.000000000000000000, 1.000000000000000000 ) ) ;
#4456=CARTESIAN_POINT ( 'NONE',  ( 3.062271323958273950, 16.80150817659525231, 19.47952243369111258 ) ) ;
#4457=CARTESIAN_POINT ( 'NONE',  ( -18.04365185506137337, -8.627086862512673093, 7.652108011868850035 ) ) ;
#4458=CARTESIAN_POINT ( 'NONE',  ( -18.47553274370957155, -7.705290464775618631, 19.33715507985239412 ) ) ;
#4471=CARTESIAN_POINT ( 'NONE',  ( 15.38564065975359796, -7.280544306537534816, 19.45164628100866722 ) ) ;
#4472=CARTESIAN_POINT ( 'NONE',  ( 5.997818345539172924, 19.09841206584651729, 7.359006845440219102 ) ) ;
#4475=CARTESIAN_POINT ( 'NONE',  ( -16.81263688882342322, 2.656251026639211421, 6.641371103590088865 ) ) ;
#4479=ORIENTED_EDGE ( 'NONE', *, *, #6561, .T. ) ;
#4481=CARTESIAN_POINT ( 'NONE',  ( -14.70303524442681997, -8.688445896238663479, 6.588756557121050683 ) ) ;
#4484=CARTESIAN_POINT ( 'NONE',  ( 16.86471733739940859, 2.322843836249472105, 18.83976166372255179 ) ) ;
#4487=CARTESIAN_POINT ( 'NONE',  ( 0.1433833641520070590, -17.02852539342428884, 7.429667576816606278 ) ) ;
#4491=CARTESIAN_POINT ( 'NONE',  ( -19.87893182697125027, 2.354587536660440072, 20.33971507717571114 ) ) ;
#4492=CARTESIAN_POINT ( 'NONE',  ( -10.47960520055065636, -7.757439966934454034, 24.50000000000000000 ) ) ;
#4495=CARTESIAN_POINT ( 'NONE',  ( 11.94600218753717868, -16.06231219995582293, 19.36813350477385143 ) ) ;
#4498=ORIENTED_EDGE ( 'NONE', *, *, #20279, .T. ) ;
#4499=CARTESIAN_POINT ( 'NONE',  ( -15.34307810681595718, 12.82926163924266483, 7.652108011868850035 ) ) ;
#4509=LINE ( 'NONE', #23664, #3372 ) ;
#4510=EDGE_LOOP ( 'NONE', ( #26970, #16542, #29849, #25228 ) ) ;
#4512=VERTEX_POINT ( 'NONE', #25323 ) ;
#4514=DIRECTION ( 'NONE',  ( -0.000000000000000000, -0.000000000000000000, -1.000000000000000000 ) ) ;
#4515=CARTESIAN_POINT ( 'NONE',  ( -17.68050765791475243, -9.349252870402523286, 7.272192800924347722 ) ) ;
#4516=CARTESIAN_POINT ( 'NONE',  ( 19.72232476070952956, 3.323723214581396412, 7.652108011868850923 ) ) ;
#4518=VERTEX_POINT ( 'NONE', #18610 ) ;
#4519=CARTESIAN_POINT ( 'NONE',  ( -16.96555893295483841, 1.647560171216679192, 18.34798005862930381 ) ) ;
#4522=CARTESIAN_POINT ( 'NONE',  ( -13.77701868333376645, 10.07013474916661266, 7.441806358946449151 ) ) ;
#4523=CARTESIAN_POINT ( 'NONE',  ( 10.50506478158603407, 13.32952022457704544, 1.500000000000000000 ) ) ;
#4524=ORIENTED_EDGE ( 'NONE', *, *, #5364, .T. ) ;
#4530=ADVANCED_FACE ( 'NONE', ( #13638 ), #23118, .F. ) ;
#4534=CARTESIAN_POINT ( 'NONE',  ( -19.93913687200723572, 1.772791844786496762, 5.951255046771932733 ) ) ;
#4536=CARTESIAN_POINT ( 'NONE',  ( 19.78337026033622337, 2.938244205458798941, 18.37250658438899009 ) ) ;
#4537=ORIENTED_EDGE ( 'NONE', *, *, #21177, .F. ) ;
#4540=CARTESIAN_POINT ( 'NONE',  ( 15.87456320658224485, -6.220724357885995204, 5.661398277488801867 ) ) ;
#4543=VERTEX_POINT ( 'NONE', #20776 ) ;
#4547=AXIS2_PLACEMENT_3D ( 'NONE', #10799, #3945, #8482 ) ;
#4548=CARTESIAN_POINT ( 'NONE',  ( -18.04365185506137337, -8.627086862512673093, 7.652108011868850035 ) ) ;
#4549=CARTESIAN_POINT ( 'NONE',  ( -6.374050743166105981, 15.83881588044503808, 18.82680253904184298 ) ) ;
#4550=LINE ( 'NONE', #23563, #29260 ) ;
#4552=CARTESIAN_POINT ( 'NONE',  ( 14.44122519041005859, -13.83658248990206729, 24.50000000000000000 ) ) ;
#4560=CARTESIAN_POINT ( 'NONE',  ( 0.000000000000000000, 0.000000000000000000, 1.500000000000001332 ) ) ;
#4561=CARTESIAN_POINT ( 'NONE',  ( -14.71441417907128013, -8.667509008793198078, 19.58863275299554019 ) ) ;
#4564=( NAMED_UNIT ( * ) SI_UNIT ( $, .STERADIAN. ) SOLID_ANGLE_UNIT ( ) );
#4568=CARTESIAN_POINT ( 'NONE',  ( 12.72536390617885438, -2.839914339433650348, 1.500000000000001332 ) ) ;
#4571=EDGE_CURVE ( 'NONE', #19951, #10643, #12792, .T. ) ;
#4576=DIRECTION ( 'NONE',  ( 1.000000000000000000, 0.000000000000000000, 0.000000000000000000 ) ) ;
#4579=DIRECTION ( 'NONE',  ( 0.000000000000000000, 0.000000000000000000, 1.000000000000000000 ) ) ;
#4582=CARTESIAN_POINT ( 'NONE',  ( -0.6660349346848405405, -20.00682905350634400, 19.33715507985239412 ) ) ;
#4584=CARTESIAN_POINT ( 'NONE',  ( -10.52692686119061172, -17.02631563033162365, 7.652108011868850035 ) ) ;
#4587=CARTESIAN_POINT ( 'NONE',  ( 0.4984457374290387488, -20.01168570850558481, 20.33971507717571114 ) ) ;
#4588=EDGE_LOOP ( 'NONE', ( #467, #6769, #28243, #8881 ) ) ;
#4591=CARTESIAN_POINT ( 'NONE',  ( 14.21537200517654398, 14.09360477215026108, 19.58863275299554019 ) ) ;
#4594=CARTESIAN_POINT ( 'NONE',  ( -15.22163550582783031, -7.663797071066537292, 20.34789198813115974 ) ) ;
#4595=DIRECTION ( 'NONE',  ( 1.000000000000000000, 0.000000000000000000, 0.000000000000000000 ) ) ;
#4599=EDGE_CURVE ( 'NONE', #14232, #5487, #9545, .T. ) ;
#4601=AXIS2_PLACEMENT_3D ( 'NONE', #26016, #2612, #9323 ) ;
#4614=CARTESIAN_POINT ( 'NONE',  ( 18.21411928606760711, -8.304179478877907528, 20.29090034784956131 ) ) ;
#4615=CARTESIAN_POINT ( 'NONE',  ( 6.270562923531074695, 19.01045013183040311, 6.755862304746362845 ) ) ;
#4619=CARTESIAN_POINT ( 'NONE',  ( 6.171684994647416822, 19.04275422834224329, 18.90679857307105749 ) ) ;
#4620=CYLINDRICAL_SURFACE ( 'NONE', #10747, 0.7499999999999997780 ) ;
#4621=CARTESIAN_POINT ( 'NONE',  ( -0.9307681286967910417, 9.436481611552762772, 1.500000000000001332 ) ) ;
#4626=CIRCLE ( 'NONE', #11618, 9.482273699623480212 ) ;
#4631=CARTESIAN_POINT ( 'NONE',  ( -18.46427634282258268, -7.732205987805706116, 6.864725433338323413 ) ) ;
#4638=DIRECTION ( 'NONE',  ( 0.000000000000000000, 0.000000000000000000, 1.000000000000000000 ) ) ;
#4643=CARTESIAN_POINT ( 'NONE',  ( 11.86528446860017105, -16.12209958341615135, 19.79423548914561692 ) ) ;
#4645=VERTEX_POINT ( 'NONE', #2533 ) ;
#4648=DIRECTION ( 'NONE',  ( -0.000000000000000000, -0.000000000000000000, 1.000000000000000000 ) ) ;
#4653=CARTESIAN_POINT ( 'NONE',  ( 18.35307771382469255, -7.992233955150557456, 18.34798005862662507 ) ) ;
#4654=CARTESIAN_POINT ( 'NONE',  ( 19.57285800138751952, 4.196195780087080607, 19.25672174529527325 ) ) ;
#4655=DIRECTION ( 'NONE',  ( 1.000000000000000000, 0.000000000000000000, 0.000000000000000000 ) ) ;
#4665=DIRECTION ( 'NONE',  ( 0.000000000000000000, 0.000000000000000000, 1.000000000000000000 ) ) ;
#4667=CARTESIAN_POINT ( 'NONE',  ( 0.8531715179115259007, -17.02613171184588126, 7.652108011868850035 ) ) ;
#4668=CARTESIAN_POINT ( 'NONE',  ( -14.76455652123169138, -8.574248774011078211, 18.84329447212443753 ) ) ;
#4669=CARTESIAN_POINT ( 'NONE',  ( -0.7220001660363114526, -9.454746441592957851, 21.50000000000000000 ) ) ;
#4672=CARTESIAN_POINT ( 'NONE',  ( 9.860909911264739591, -13.90333503211347654, 7.652108011868850035 ) ) ;
#4674=CARTESIAN_POINT ( 'NONE',  ( -13.87349289520722806, 9.945669722324359086, 7.280727868105637768 ) ) ;
#4676=VERTEX_POINT ( 'NONE', #33 ) ;
#4677=VERTEX_POINT ( 'NONE', #2680 ) ;
#4679=LINE ( 'NONE', #9514, #27590 ) ;
#4680=DIRECTION ( 'NONE',  ( 0.8412535328311810945, 0.5406408174555976665, 0.000000000000000000 ) ) ;
#4682=DIRECTION ( 'NONE',  ( 0.9594929736144951482, -0.2817325568414371095, 0.000000000000000000 ) ) ;
#4685=AXIS2_PLACEMENT_3D ( 'NONE', #850, #28781, #24399 ) ;
#4688=CARTESIAN_POINT ( 'NONE',  ( -19.88720069594608475, 2.282442057551330450, 7.627891251804737927 ) ) ;
#4691=VERTEX_POINT ( 'NONE', #27326 ) ;
#4692=DIRECTION ( 'NONE',  ( 0.000000000000000000, 0.000000000000000000, 1.000000000000000000 ) ) ;
#4693=VERTEX_POINT ( 'NONE', #20140 ) ;
#4696=ORIENTED_EDGE ( 'NONE', *, *, #17013, .F. ) ;
#4700=CARTESIAN_POINT ( 'NONE',  ( -18.30120037456298832, -8.066899270990512960, 5.849008070840539197 ) ) ;
#4703=EDGE_CURVE ( 'NONE', #17954, #21094, #3610, .T. ) ;
#4706=DIRECTION ( 'NONE',  ( 0.000000000000000000, 0.000000000000000000, -1.000000000000000000 ) ) ;
#4708=CARTESIAN_POINT ( 'NONE',  ( 15.44332723074500180, -7.163653983975262207, 6.143977687428009204 ) ) ;
#4713=CARTESIAN_POINT ( 'NONE',  ( -15.10044507415838488, -7.916284227987608446, 20.33971507717571114 ) ) ;
#4714=CARTESIAN_POINT ( 'NONE',  ( 6.631244434206235105, 6.812559277181991391, 1.500000000000001332 ) ) ;
#4715=CARTESIAN_POINT ( 'NONE',  ( 4.892923698309762592, 16.30563068515024838, 6.143977687428008316 ) ) ;
#4718=DIRECTION ( 'NONE',  ( -1.000000000000000000, 0.000000000000000000, 0.000000000000000000 ) ) ;
#4725=CARTESIAN_POINT ( 'NONE',  ( 0.000000000000000000, 0.000000000000000000, 1.500000000000001332 ) ) ;
#4729=CARTESIAN_POINT ( 'NONE',  ( 7.730328572437743517, -4.608906612435629491, 1.500000000000001332 ) ) ;
#4732=CARTESIAN_POINT ( 'NONE',  ( 0.5496282100021194772, -17.03044801512709938, 20.32842677360128292 ) ) ;
#4733=CARTESIAN_POINT ( 'NONE',  ( -7.919226493207299100, -15.11997014267743822, 5.951255046771932733 ) ) ;
#4734=CARTESIAN_POINT ( 'NONE',  ( 4.892923698324559645, 16.30563068514543446, 18.83976166372255534 ) ) ;
#4735=CARTESIAN_POINT ( 'NONE',  ( 1.303806812501130619, -19.97511938206333681, 19.69140814234746273 ) ) ;
#4736=ORIENTED_EDGE ( 'NONE', *, *, #8425, .F. ) ;
#4737=CARTESIAN_POINT ( 'NONE',  ( 18.70859934877966424, -7.070433808158458788, 6.919864475265772086 ) ) ;
#4739=CARTESIAN_POINT ( 'NONE',  ( 11.98626544954000117, 12.14249340222027129, 18.50655187082627862 ) ) ;
#4743=CARTESIAN_POINT ( 'NONE',  ( -17.66624025659152863, -9.413543259203214220, 6.131018562779544823 ) ) ;
#4744=CARTESIAN_POINT ( 'NONE',  ( 9.349584168494304848, 12.69858007495367680, 1.500000000000001332 ) ) ;
#4753=CARTESIAN_POINT ( 'NONE',  ( 2.810445847081857629, 9.056208293496320394, 1.500000000000001332 ) ) ;
#4755=CARTESIAN_POINT ( 'NONE',  ( -12.74366836927934976, 11.28516576207253053, 6.974106381145714018 ) ) ;
#4757=ORIENTED_EDGE ( 'NONE', *, *, #14546, .T. ) ;
#4758=CARTESIAN_POINT ( 'NONE',  ( 17.97060409579513163, -8.818932628521073624, 18.90679857307105749 ) ) ;
#4759=CARTESIAN_POINT ( 'NONE',  ( 6.275630943545792206, 19.00876817605120195, 6.641371103590088865 ) ) ;
#4761=CARTESIAN_POINT ( 'NONE',  ( 4.575061044035268587, 16.40537387836874927, 20.19668224736330941 ) ) ;
#4772=VERTEX_POINT ( 'NONE', #22468 ) ;
#4773=CARTESIAN_POINT ( 'NONE',  ( -18.11003155545034460, -8.529482236167142517, 7.652108011868850035 ) ) ;
#4775=CARTESIAN_POINT ( 'NONE',  ( -3.196529495465446402, -8.413215745754985875, 1.500000000000001332 ) ) ;
#4782=LINE ( 'NONE', #6525, #15356 ) ;
#4784=ADVANCED_FACE ( 'NONE', ( #24353 ), #3000, .F. ) ;
#4785=CARTESIAN_POINT ( 'NONE',  ( 11.17648341053133976, -16.60731568869665153, 20.34789198813115263 ) ) ;
#4787=EDGE_CURVE ( 'NONE', #1099, #23147, #22773, .T. ) ;
#4790=CIRCLE ( 'NONE', #8782, 9.482273699623480212 ) ;
#4791=EDGE_CURVE ( 'NONE', #7470, #18940, #19832, .T. ) ;
#4792=CARTESIAN_POINT ( 'NONE',  ( 5.291489565152559749, 19.28730510418394672, 18.34798005863226678 ) ) ;
#4794=ORIENTED_EDGE ( 'NONE', *, *, #11872, .T. ) ;
#4796=CARTESIAN_POINT ( 'NONE',  ( 12.51082390549570889, 11.56795297236522480, 20.32842677360128292 ) ) ;
#4797=CARTESIAN_POINT ( 'NONE',  ( 15.90320373664000009, -6.152843468454362252, 18.37415474056476938 ) ) ;
#4798=CARTESIAN_POINT ( 'NONE',  ( 19.60578376704636838, 4.040313317649107283, 19.89182036555910571 ) ) ;
#4799=AXIS2_PLACEMENT_3D ( 'NONE', #12088, #24391, #14879 ) ;
#4802=CARTESIAN_POINT ( 'NONE',  ( 14.44122519041005859, -13.83658248990206729, 1.500000000000001332 ) ) ;
#4804=EDGE_CURVE ( 'NONE', #20273, #16284, #11321, .T. ) ;
#4814=CARTESIAN_POINT ( 'NONE',  ( 0.1624814967139596167, -17.02900520012434882, 18.54473042795395443 ) ) ;
#4816=CARTESIAN_POINT ( 'NONE',  ( 0.7902931953360854411, -20.00234323981187856, 7.559636331181775581 ) ) ;
#4819=VERTEX_POINT ( 'NONE', #23227 ) ;
#4820=ADVANCED_FACE ( 'NONE', ( #6098 ), #20354, .T. ) ;
#4821=CARTESIAN_POINT ( 'NONE',  ( -19.85654738780300832, 2.535877853918452995, 18.34777357837152323 ) ) ;
#4823=VECTOR ( 'NONE', #18717, 1000.000000000000000 ) ;
#4826=ORIENTED_EDGE ( 'NONE', *, *, #5765, .F. ) ;
#4830=CARTESIAN_POINT ( 'NONE',  ( -15.16517293421789070, -7.781889191988407894, 7.652108011868850923 ) ) ;
#4835=EDGE_CURVE ( 'NONE', #27607, #115, #14177, .T. ) ;
#4837=EDGE_CURVE ( 'NONE', #9540, #115, #19279, .T. ) ;
#4838=ADVANCED_FACE ( 'NONE', ( #23683 ), #6859, .F. ) ;
#4841=CARTESIAN_POINT ( 'NONE',  ( -17.59500444164589794, -9.508866521682287853, 19.61564845152807735 ) ) ;
#4843=VERTEX_POINT ( 'NONE', #11855 ) ;
#4844=CARTESIAN_POINT ( 'NONE',  ( 15.48724201788533428, 12.68311944884417919, 6.211014596808754007 ) ) ;
#4845=ORIENTED_EDGE ( 'NONE', *, *, #25979, .F. ) ;
#4846=VECTOR ( 'NONE', #4013, 1000.000000000000000 ) ;
#4851=VECTOR ( 'NONE', #26357, 1000.000000000000227 ) ;
#4858=CIRCLE ( 'NONE', #19287, 0.7499999999999997780 ) ;
#4863=CARTESIAN_POINT ( 'NONE',  ( -8.549050687778191104, -4.102102735472431760, 1.500000000000001332 ) ) ;
#4867=EDGE_LOOP ( 'NONE', ( #30617, #2776, #28876, #19505 ) ) ;
#4872=CARTESIAN_POINT ( 'NONE',  ( 4.644508076310276401, 16.38413139300089227, 7.453286057244488561 ) ) ;
#4879=CARTESIAN_POINT ( 'NONE',  ( -6.933969404122152902, 18.75953273845654579, 6.788986777570698905 ) ) ;
#4881=DIRECTION ( 'NONE',  ( -0.000000000000000000, -0.000000000000000000, 1.000000000000000000 ) ) ;
#4882=VECTOR ( 'NONE', #29455, 1000.000000000000000 ) ;
#4883=VERTEX_POINT ( 'NONE', #4523 ) ;
#4886=AXIS2_PLACEMENT_3D ( 'NONE', #26893, #8326, #17842 ) ;
#4887=VERTEX_POINT ( 'NONE', #23995 ) ;
#4888=VERTEX_POINT ( 'NONE', #12012 ) ;
#4891=ORIENTED_EDGE ( 'NONE', *, *, #21373, .F. ) ;
#4892=ORIENTED_EDGE ( 'NONE', *, *, #14529, .F. ) ;
#4893=CARTESIAN_POINT ( 'NONE',  ( -0.1864951924744789880, -20.01724188655222747, 18.49267272388512140 ) ) ;
#4894=CARTESIAN_POINT ( 'NONE',  ( -9.972083266784114386, -17.35726207598482063, 5.872146474157316831 ) ) ;
#4895=AXIS2_PLACEMENT_3D ( 'NONE', #25187, #15525, #27081 ) ;
#4897=CARTESIAN_POINT ( 'NONE',  ( 1.568770080425526237, -16.99791492429841711, 19.97651184436794125 ) ) ;
#4898=CIRCLE ( 'NONE', #9376, 20.00000000000000000 ) ;
#4900=CARTESIAN_POINT ( 'NONE',  ( 11.11118388262826251, -16.62953976291647962, 5.652196082369964181 ) ) ;
#4902=CARTESIAN_POINT ( 'NONE',  ( 11.81884104268966773, 12.31686436340674184, 19.97651184436794125 ) ) ;
#4907=CARTESIAN_POINT ( 'NONE',  ( -17.69908921317806261, -9.351398086983019553, 6.041646659195333058 ) ) ;
#4908=DIRECTION ( 'NONE',  ( -0.000000000000000000, -0.000000000000000000, -1.000000000000000000 ) ) ;
#4917=CARTESIAN_POINT ( 'NONE',  ( -14.70379955820389561, 13.58362208154139772, 6.864725433338323413 ) ) ;
#4919=ORIENTED_EDGE ( 'NONE', *, *, #332, .F. ) ;
#4922=DIRECTION ( 'NONE',  ( 0.000000000000000000, 0.000000000000000000, 1.000000000000000000 ) ) ;
#4924=CARTESIAN_POINT ( 'NONE',  ( 6.060672894209297112, 19.07852886212369725, 6.018569869498933578 ) ) ;
#4926=CARTESIAN_POINT ( 'NONE',  ( 4.971436688744666377, 16.28007576866361816, 19.66989035740801839 ) ) ;
#4933=DIRECTION ( 'NONE',  ( -0.000000000000000000, -0.000000000000000000, 1.000000000000000000 ) ) ;
#4934=B_SPLINE_CURVE_WITH_KNOTS ( 'NONE', 3,
 ( #23015, #20387, #1363, #6037, #10878, #1820, #3855, #4008, #20678, #15546, #13533, #20222, #1213, #11343, #1520, #25531, #8844, #29911, #20532, #25061 ),
 .UNSPECIFIED., .F., .F.,
 ( 4, 2, 2, 2, 2, 2, 2, 2, 2, 4 ),
 ( 0.000000000000000000, 0.06250000000000006939, 0.1250000000000001388, 0.1875000000000002220, 0.2187499999999995282, 0.2499999999999988065, 0.3124999999999990563, 0.3749999999999992784, 0.4374999999999995559, 0.4999999999999997224 ),
 .UNSPECIFIED. ) ;
#4936=EDGE_CURVE ( 'NONE', #27180, #9077, #13812, .T. ) ;
#4937=DIRECTION ( 'NONE',  ( 1.000000000000000000, 0.000000000000000000, 0.000000000000000000 ) ) ;
#4938=ORIENTED_EDGE ( 'NONE', *, *, #29023, .F. ) ;
#4940=CARTESIAN_POINT ( 'NONE',  ( -18.28579658156514043, -8.145820804509362745, 5.796888747622817029 ) ) ;
#4944=DIRECTION ( 'NONE',  ( 0.000000000000000000, 0.000000000000000000, 1.000000000000000000 ) ) ;
#4949=VERTEX_POINT ( 'NONE', #14648 ) ;
#4950=CARTESIAN_POINT ( 'NONE',  ( -7.667077102831937552, 13.77986170986486592, 1.500000000000001332 ) ) ;
#4954=VERTEX_POINT ( 'NONE', #21355 ) ;
#4955=EDGE_CURVE ( 'NONE', #4819, #2473, #21661, .T. ) ;
#4958=EDGE_LOOP ( 'NONE', ( #3675, #4537, #8204, #25298 ) ) ;
#4963=EDGE_CURVE ( 'NONE', #21613, #27751, #9203, .T. ) ;
#4964=CARTESIAN_POINT ( 'NONE',  ( 16.17271416092066261, -5.480318835022395696, 19.69140814234746273 ) ) ;
#4965=CARTESIAN_POINT ( 'NONE',  ( 16.74250592927944936, 3.198927888044590162, 18.34798005862662507 ) ) ;
#4973=EDGE_CURVE ( 'NONE', #30466, #23022, #14032, .T. ) ;
#4974=LINE ( 'NONE', #19320, #10114 ) ;
#4975=CARTESIAN_POINT ( 'NONE',  ( -12.74837729798237440, 11.28012212083751642, 19.00652017443069752 ) ) ;
#4978=CARTESIAN_POINT ( 'NONE',  ( 1.047421501641249364, -17.02264912680065478, 18.34938820207545263 ) ) ;
#4979=CARTESIAN_POINT ( 'NONE',  ( 16.85411910731514240, 2.412525337365567513, 18.71435384576123440 ) ) ;
#4982=CARTESIAN_POINT ( 'NONE',  ( 15.78348099220817957, -6.430800111306883338, 5.653912893140659257 ) ) ;
#4983=CARTESIAN_POINT ( 'NONE',  ( -15.35487439336962012, 12.84287527963942921, 7.652108011868850035 ) ) ;
#4984=CARTESIAN_POINT ( 'NONE',  ( 1.000000000000008438, 15.73749217771910125, -0.6213203435596476032 ) ) ;
#4989=PLANE ( 'NONE',  #9636 ) ;
#4990=ADVANCED_FACE ( 'NONE', ( #7333 ), #298, .F. ) ;
#4992=CARTESIAN_POINT ( 'NONE',  ( -5.128149923613388950, 16.24357618101654666, 18.44501272782439827 ) ) ;
#4993=CARTESIAN_POINT ( 'NONE',  ( -15.22000698767478788, -7.667275872209097898, 5.651492010659115550 ) ) ;
#4996=LINE ( 'NONE', #14656, #29364 ) ;
#5003=CARTESIAN_POINT ( 'NONE',  ( 12.65169814564037054, 11.40562544919841415, 7.557577766377196582 ) ) ;
#5007=CARTESIAN_POINT ( 'NONE',  ( 16.56110944985486455, 4.167213836826286766, 19.61324152429826739 ) ) ;
#5012=CARTESIAN_POINT ( 'NONE',  ( 5.151948548241254144, 19.34356600583523544, 5.661398277488802755 ) ) ;
#5014=DIRECTION ( 'NONE',  ( 0.000000000000000000, 0.000000000000000000, 1.000000000000000000 ) ) ;
#5016=CIRCLE ( 'NONE', #9011, 9.482273699623480212 ) ;
#5022=DIRECTION ( 'NONE',  ( 0.000000000000000000, 0.000000000000000000, 1.000000000000000000 ) ) ;
#5023=ORIENTED_EDGE ( 'NONE', *, *, #28486, .F. ) ;
#5025=CARTESIAN_POINT ( 'NONE',  ( -17.70591931088123516, -9.338465149306660606, 19.97651184436794125 ) ) ;
#5031=EDGE_LOOP ( 'NONE', ( #26106, #4757, #2029, #7902 ) ) ;
#5033=CARTESIAN_POINT ( 'NONE',  ( 0.000000000000000000, 0.000000000000000000, 1.500000000000001332 ) ) ;
#5036=CARTESIAN_POINT ( 'NONE',  ( 19.58271949849003590, 4.064458250759529712, 7.161525567826888761 ) ) ;
#5042=ORIENTED_EDGE ( 'NONE', *, *, #2561, .T. ) ;
#5043=DIRECTION ( 'NONE',  ( -0.000000000000000000, -0.000000000000000000, 1.000000000000000000 ) ) ;
#5044=DIRECTION ( 'NONE',  ( 0.000000000000000000, 0.000000000000000000, 1.000000000000000000 ) ) ;
#5046=EDGE_LOOP ( 'NONE', ( #12211, #4039 ) ) ;
#5047=DIRECTION ( 'NONE',  ( 0.6548607339452783282, -0.7557495743542641531, 0.000000000000000000 ) ) ;
#5050=ORIENTED_EDGE ( 'NONE', *, *, #25458, .T. ) ;
#5051=LINE ( 'NONE', #26101, #2914 ) ;
#5052=CARTESIAN_POINT ( 'NONE',  ( -7.870033247355589623, -15.14769711951103304, 7.280727868105637768 ) ) ;
#5054=CARTESIAN_POINT ( 'NONE',  ( 1.342146863054723971, -19.97260970722470219, 19.58863275299554019 ) ) ;
#5056=CARTESIAN_POINT ( 'NONE',  ( 4.045242219987652987, 16.55840560649981441, 5.652196082368482699 ) ) ;
#5058=CARTESIAN_POINT ( 'NONE',  ( 11.72050123711541225, 12.41739018441317199, 18.92976555901915603 ) ) ;
#5061=ADVANCED_FACE ( 'NONE', ( #9936 ), #879, .F. ) ;
#5064=VECTOR ( 'NONE', #23251, 1000.000000000000000 ) ;
#5065=CARTESIAN_POINT ( 'NONE',  ( 11.80555446153501897, -11.55276080277260320, 24.50000000000000000 ) ) ;
#5066=CARTESIAN_POINT ( 'NONE',  ( -15.06439250341027858, -7.989583865232171789, 5.678370764302467677 ) ) ;
#5067=CARTESIAN_POINT ( 'NONE',  ( -6.789382699754177963, 18.83122862112907114, 7.196036389296800451 ) ) ;
#5071=ORIENTED_EDGE ( 'NONE', *, *, #5596, .T. ) ;
#5075=CARTESIAN_POINT ( 'NONE',  ( 1.195154792889394635, 9.406652940105990623, 13.00000000000000178 ) ) ;
#5080=CARTESIAN_POINT ( 'NONE',  ( 16.12090643793933964, -5.615848544254287589, 19.96568007040468373 ) ) ;
#5081=DIRECTION ( 'NONE',  ( 1.000000000000000000, -0.000000000000000000, 0.000000000000000000 ) ) ;
#5083=CARTESIAN_POINT ( 'NONE',  ( 4.159666964149443480, 16.52698801271857221, 20.34789198813115263 ) ) ;
#5084=CARTESIAN_POINT ( 'NONE',  ( 14.26939381558975484, 14.03892697587676786, 7.098451512883313441 ) ) ;
#5086=CARTESIAN_POINT ( 'NONE',  ( -8.321991900554296606, -14.88664253293455353, 18.34938820207545263 ) ) ;
#5088=EDGE_LOOP ( 'NONE', ( #29820, #29190, #17479, #29943 ) ) ;
#5090=B_SPLINE_CURVE_WITH_KNOTS ( 'NONE', 3,
 ( #2770, #5570, #15066, #5260, #24581, #3224, #29437, #17108, #1047, #20065, #29585, #7601, #8217, #14761, #21787, #425, #9943, #720 ),
 .UNSPECIFIED., .F., .F.,
 ( 4, 2, 2, 2, 2, 2, 2, 2, 4 ),
 ( 0.000000000000000000, 0.0003967869494442915167, 0.0007935738988885830333, 0.001190360848332874550, 0.001587147797777166067, 0.001983934747221457583, 0.002380721696665749100, 0.002777508646110040617, 0.003174295595554332133 ),
 .UNSPECIFIED. ) ;
#5091=CARTESIAN_POINT ( 'NONE',  ( 8.413215745754998309, -3.196529495465417980, 1.500000000000001332 ) ) ;
#5094=LINE ( 'NONE', #26142, #337 ) ;
#5095=DIRECTION ( 'NONE',  ( -1.000000000000000000, 0.000000000000000000, -0.000000000000000000 ) ) ;
#5096=CARTESIAN_POINT ( 'NONE',  ( 14.53924466656744663, 13.73408656550489759, 7.528076282304593470 ) ) ;
#5098=CARTESIAN_POINT ( 'NONE',  ( 0.6691466709101926424, -17.02906906675068299, 5.657991946698900598 ) ) ;
#5099=EDGE_CURVE ( 'NONE', #10066, #1290, #24575, .T. ) ;
#5100=FACE_OUTER_BOUND ( 'NONE', #23941, .T. ) ;
#5112=CARTESIAN_POINT ( 'NONE',  ( 14.97341519046260316, 13.28616376876794725, 20.34789198813115263 ) ) ;
#5117=AXIS2_PLACEMENT_3D ( 'NONE', #12449, #17429, #885 ) ;
#5119=CARTESIAN_POINT ( 'NONE',  ( 19.63091490780798765, 3.916522693408248657, 18.64703902303423178 ) ) ;
#5120=CARTESIAN_POINT ( 'NONE',  ( -15.71962203721309592, -1.249857212218242752, 24.50000000000000000 ) ) ;
#5126=CARTESIAN_POINT ( 'NONE',  ( 9.163215745754998309, -3.196529495465417980, 21.50000000000000000 ) ) ;
#5127=CARTESIAN_POINT ( 'NONE',  ( -17.76782356872499591, -9.182228809334526787, 7.454606537396346155 ) ) ;
#5128=LINE ( 'NONE', #12624, #8774 ) ;
#5132=CARTESIAN_POINT ( 'NONE',  ( 8.637616862297843312, -3.912171961291978306, 1.500000000000001332 ) ) ;
#5135=CARTESIAN_POINT ( 'NONE',  ( 10.33891776879019986, -17.14136798460503996, 7.080843742048788414 ) ) ;
#5138=EDGE_LOOP ( 'NONE', ( #18048, #9564, #12206, #9985 ) ) ;
#5141=CARTESIAN_POINT ( 'NONE',  ( 10.68225562352957070, -16.90870462272443575, 7.526993102356321685 ) ) ;
#5142=CARTESIAN_POINT ( 'NONE',  ( -5.548724899233040908, 19.23375410423647836, 7.557577766377196582 ) ) ;
#5145=ORIENTED_EDGE ( 'NONE', *, *, #9638, .F. ) ;
#5149=FACE_OUTER_BOUND ( 'NONE', #26061, .T. ) ;
#5151=ORIENTED_EDGE ( 'NONE', *, *, #14931, .T. ) ;
#5155=CARTESIAN_POINT ( 'NONE',  ( 18.59495189863232412, -7.412450086248064451, 7.441806358946449151 ) ) ;
#5159=EDGE_CURVE ( 'NONE', #1292, #21299, #24291, .T. ) ;
#5161=ORIENTED_EDGE ( 'NONE', *, *, #26331, .F. ) ;
#5162=EDGE_CURVE ( 'NONE', #15220, #9060, #714, .T. ) ;
#5163=CARTESIAN_POINT ( 'NONE',  ( 4.972463595808061854, 19.39063357279558275, 5.704143890883081269 ) ) ;
#5164=EDGE_CURVE ( 'NONE', #624, #11023, #30257, .T. ) ;
#5169=ADVANCED_FACE ( 'NONE', ( #22400 ), #19744, .F. ) ;
#5170=CARTESIAN_POINT ( 'NONE',  ( 10.58932223943304685, -16.96688107778387078, 18.54479204710284179 ) ) ;
#5171=EDGE_LOOP ( 'NONE', ( #3384, #908, #26832, #3749 ) ) ;
#5177=ORIENTED_EDGE ( 'NONE', *, *, #5968, .F. ) ;
#5183=DIRECTION ( 'NONE',  ( 1.000000000000000000, 0.000000000000000000, 0.000000000000000000 ) ) ;
#5186=EDGE_CURVE ( 'NONE', #23254, #15912, #894, .T. ) ;
#5190=ORIENTED_EDGE ( 'NONE', *, *, #4599, .F. ) ;
#5198=ORIENTED_EDGE ( 'NONE', *, *, #4973, .T. ) ;
#5200=ORIENTED_EDGE ( 'NONE', *, *, #8775, .T. ) ;
#5202=CARTESIAN_POINT ( 'NONE',  ( -0.2093543646724285723, -17.02041581256300873, 19.11611934778430921 ) ) ;
#5208=CYLINDRICAL_SURFACE ( 'NONE', #28803, 0.7500000000000006661 ) ;
#5213=CARTESIAN_POINT ( 'NONE',  ( 14.29853178503252309, 14.00938365128603458, 18.82680253904184298 ) ) ;
#5217=CARTESIAN_POINT ( 'NONE',  ( -10.52692833102915770, -17.02631732661572883, 20.34789198813115263 ) ) ;
#5219=DIRECTION ( 'NONE',  ( -0.7557495743542579358, 0.6548607339452855447, 0.000000000000000000 ) ) ;
#5221=CARTESIAN_POINT ( 'NONE',  ( -17.75446986341067301, 9.207540381081360081, 1.500000000000001332 ) ) ;
#5223=DIRECTION ( 'NONE',  ( 0.000000000000000000, 0.000000000000000000, 1.000000000000000000 ) ) ;
#5225=ORIENTED_EDGE ( 'NONE', *, *, #9404, .F. ) ;
#5229=CARTESIAN_POINT ( 'NONE',  ( -8.325649706230674241, -14.88445757356298493, 7.652108011868850035 ) ) ;
#5230=CARTESIAN_POINT ( 'NONE',  ( -13.16038179581985723, 10.81844819380990330, 7.595116371587256054 ) ) ;
#5233=SHAPE_DEFINITION_REPRESENTATION ( #23350, #10497 ) ;
#5238=CARTESIAN_POINT ( 'NONE',  ( 6.249808329856146649, 19.01727106391103916, 19.11611934778430921 ) ) ;
#5240=DIRECTION ( 'NONE',  ( 0.000000000000000000, 0.000000000000000000, 1.000000000000000000 ) ) ;
#5244=ORIENTED_EDGE ( 'NONE', *, *, #19672, .F. ) ;
#5249=CARTESIAN_POINT ( 'NONE',  ( -15.51812306427841293, -7.001296657735112561, 6.111214848085761986 ) ) ;
#5255=DIRECTION ( 'NONE',  ( 0.6548607339452890974, 0.7557495743542548272, 0.000000000000000000 ) ) ;
#5258=ORIENTED_EDGE ( 'NONE', *, *, #21763, .T. ) ;
#5260=CARTESIAN_POINT ( 'NONE',  ( 4.800123045415255696, 19.41580659536132103, 5.779535427900766464 ) ) ;
#5263=DIRECTION ( 'NONE',  ( -0.9096319953545183301, -0.4154150130018863796, -0.000000000000000000 ) ) ;
#5266=CARTESIAN_POINT ( 'NONE',  ( 13.01404215953673571, 10.97082360537801193, 19.45164628100866722 ) ) ;
#5267=VECTOR ( 'NONE', #14540, 1000.000000000000000 ) ;
#5268=CARTESIAN_POINT ( 'NONE',  ( -11.06207408980607276, -16.68369011021418302, 7.429667576816606278 ) ) ;
#5269=ORIENTED_EDGE ( 'NONE', *, *, #7968, .F. ) ;
#5271=CARTESIAN_POINT ( 'NONE',  ( -15.73346977245379819, 12.34774510571039308, 20.15039051365863898 ) ) ;
#5273=ADVANCED_FACE ( 'NONE', ( #29579 ), #11169, .F. ) ;
#5277=CARTESIAN_POINT ( 'NONE',  ( 6.974883619896790954, 5.687793815610376669, 21.50000000000000000 ) ) ;
#5282=CARTESIAN_POINT ( 'NONE',  ( -6.359874605901119082, 15.84393421166758742, 19.89182036555910571 ) ) ;
#5283=CARTESIAN_POINT ( 'NONE',  ( -14.99868389510896982, 13.25752457422374597, 20.19668224736330941 ) ) ;
#5288=ORIENTED_EDGE ( 'NONE', *, *, #28220, .T. ) ;
#5289=CARTESIAN_POINT ( 'NONE',  ( 9.331524088667746852, -14.24511854140750522, 5.862424720655265098 ) ) ;
#5292=CARTESIAN_POINT ( 'NONE',  ( 19.85631519639702347, 2.394924755340403166, 7.267242832833948007 ) ) ;
#5301=CARTESIAN_POINT ( 'NONE',  ( 5.296161872597630271, 19.28602264385381204, 7.652108011868850035 ) ) ;
#5305=CARTESIAN_POINT ( 'NONE',  ( 18.33793066653144521, -7.982499537706466697, 5.652196082369965069 ) ) ;
#5307=VECTOR ( 'NONE', #17672, 1000.000000000000000 ) ;
#5309=ORIENTED_EDGE ( 'NONE', *, *, #8981, .F. ) ;
#5310=CARTESIAN_POINT ( 'NONE',  ( 16.19464367748838640, -5.422319245274333177, 6.672349528511551497 ) ) ;
#5314=CARTESIAN_POINT ( 'NONE',  ( -12.86767874445213877, -1.850092897552710225, 24.50000000000000000 ) ) ;
#5318=CARTESIAN_POINT ( 'NONE',  ( 15.41296542101254552, 5.939519782021115191, 24.50000000000000000 ) ) ;
#5326=CARTESIAN_POINT ( 'NONE',  ( 18.33599632111990729, -7.986941774664182425, 7.652108011868850035 ) ) ;
#5328=AXIS2_PLACEMENT_3D ( 'NONE', #21950, #12463, #14630 ) ;
#5334=CARTESIAN_POINT ( 'NONE',  ( -15.17333614897415650, 13.03014763290140721, 20.32243167357988867 ) ) ;
#5335=CARTESIAN_POINT ( 'NONE',  ( 4.303751186762871939, 16.48600304569812991, 7.626437579292366209 ) ) ;
#5345=EDGE_CURVE ( 'NONE', #4954, #4066, #20204, .T. ) ;
#5347=CYLINDRICAL_SURFACE ( 'NONE', #23379, 0.7500000000000006661 ) ;
#5348=VERTEX_POINT ( 'NONE', #3537 ) ;
#5354=AXIS2_PLACEMENT_3D ( 'NONE', #16823, #26336, #9959 ) ;
#5360=VECTOR ( 'NONE', #13631, 1000.000000000000000 ) ;
#5364=EDGE_CURVE ( 'NONE', #30675, #11240, #25192, .T. ) ;
#5366=DIRECTION ( 'NONE',  ( -1.000000000000000000, 0.000000000000000000, 0.000000000000000000 ) ) ;
#5372=CARTESIAN_POINT ( 'NONE',  ( -17.60607916434269526, -9.525343863633429109, 6.447548852708279377 ) ) ;
#5373=CARTESIAN_POINT ( 'NONE',  ( -6.855891330591546762, 18.80700764124136271, 6.233981582756856987 ) ) ;
#5374=DIRECTION ( 'NONE',  ( 1.000000000000000000, 0.000000000000000000, 0.000000000000000000 ) ) ;
#5376=DIRECTION ( 'NONE',  ( -0.000000000000000000, -0.000000000000000000, 1.000000000000000000 ) ) ;
#5377=AXIS2_PLACEMENT_3D ( 'NONE', #17445, #26968, #5589 ) ;
#5379=EDGE_LOOP ( 'NONE', ( #4794, #20659, #19453, #6625 ) ) ;
#5382=CARTESIAN_POINT ( 'NONE',  ( -5.380257496407078399, 19.26296000801971431, 18.54479204710283824 ) ) ;
#5383=EDGE_CURVE ( 'NONE', #15220, #26699, #2383, .T. ) ;
#5384=CARTESIAN_POINT ( 'NONE',  ( -9.185733585337896301, 2.352830851074203533, 21.50000000000000000 ) ) ;
#5385=EDGE_CURVE ( 'NONE', #17362, #30019, #18909, .T. ) ;
#5386=CARTESIAN_POINT ( 'NONE',  ( 0.000000000000000000, 0.000000000000000000, 1.500000000000001332 ) ) ;
#5390=CARTESIAN_POINT ( 'NONE',  ( 15.81416325002590817, -6.360572704314725101, 18.34798005862930736 ) ) ;
#5400=VERTEX_POINT ( 'NONE', #4744 ) ;
#5401=EDGE_CURVE ( 'NONE', #13443, #24159, #26267, .T. ) ;
#5402=DIRECTION ( 'NONE',  ( 0.000000000000000000, 0.000000000000000000, -1.000000000000000000 ) ) ;
#5403=ADVANCED_FACE ( 'NONE', ( #13962 ), #16147, .F. ) ;
#5407=EDGE_LOOP ( 'NONE', ( #25318, #3596 ) ) ;
#5409=FACE_OUTER_BOUND ( 'NONE', #25094, .T. ) ;
#5413=CARTESIAN_POINT ( 'NONE',  ( 0.000000000000000000, 0.000000000000000000, 1.500000000000001332 ) ) ;
#5414=CARTESIAN_POINT ( 'NONE',  ( -3.000000000000041744, 1.387778780781445676E-14, 24.50000000000000000 ) ) ;
#5416=EDGE_LOOP ( 'NONE', ( #30246, #5071, #3786, #1010 ) ) ;
#5417=EDGE_CURVE ( 'NONE', #25523, #28836, #28618, .T. ) ;
#5418=CIRCLE ( 'NONE', #20780, 9.482273699623480212 ) ;
#5419=CYLINDRICAL_SURFACE ( 'NONE', #22709, 9.482273699623480212 ) ;
#5420=DIRECTION ( 'NONE',  ( 1.000000000000000000, 0.000000000000000000, 0.000000000000000000 ) ) ;
#5426=ADVANCED_FACE ( 'NONE', ( #25821 ), #1803, .F. ) ;
#5431=CARTESIAN_POINT ( 'NONE',  ( 12.77540468287705444, 11.25967455357098679, 20.12545155307891065 ) ) ;
#5432=CARTESIAN_POINT ( 'NONE',  ( -11.33306590618138543, -16.50086680533498296, 6.974106381145714018 ) ) ;
#5433=ORIENTED_EDGE ( 'NONE', *, *, #5934, .F. ) ;
#5434=CARTESIAN_POINT ( 'NONE',  ( 18.41033144393026078, -7.859752488074927435, 20.33971507717571114 ) ) ;
#5439=CARTESIAN_POINT ( 'NONE',  ( -6.187077094091591789, 11.47693674426096955, 1.500000000000001332 ) ) ;
#5443=ORIENTED_EDGE ( 'NONE', *, *, #20483, .F. ) ;
#5445=CARTESIAN_POINT ( 'NONE',  ( -6.575147850411302564, 18.90724948634255753, 20.13759033520874908 ) ) ;
#5446=CARTESIAN_POINT ( 'NONE',  ( -13.09005700315871579, 10.89973235955168107, 20.25336174263950184 ) ) ;
#5447=VECTOR ( 'NONE', #30090, 1000.000000000000000 ) ;
#5448=LINE ( 'NONE', #596, #11248 ) ;
#5450=CARTESIAN_POINT ( 'NONE',  ( -5.976018955020170331, 19.08630078664910812, 5.652196082369963293 ) ) ;
#5451=ORIENTED_EDGE ( 'NONE', *, *, #17497, .T. ) ;
#5453=CARTESIAN_POINT ( 'NONE',  ( 10.92986663323816821, -16.77091174116444705, 5.670038381137163519 ) ) ;
#5454=AXIS2_PLACEMENT_3D ( 'NONE', #8164, #27188, #15316 ) ;
#5456=CARTESIAN_POINT ( 'NONE',  ( 19.86476987328767763, 2.322391784566621542, 6.144783687052517429 ) ) ;
#5458=ORIENTED_EDGE ( 'NONE', *, *, #4112, .F. ) ;
#5460=CARTESIAN_POINT ( 'NONE',  ( 10.25394813640221692, -17.17138746996171506, 6.781503518395080476 ) ) ;
#5462=DIRECTION ( 'NONE',  ( 1.000000000000000000, 0.000000000000000000, 0.000000000000000000 ) ) ;
#5463=CARTESIAN_POINT ( 'NONE',  ( 11.66432357650252349, 12.47412091822830149, 6.521906765011497242 ) ) ;
#5465=CARTESIAN_POINT ( 'NONE',  ( 6.139601762201234436, 19.03438667047814903, 6.144783687052517429 ) ) ;
#5470=CARTESIAN_POINT ( 'NONE',  ( 16.85411910731515306, 2.412525337365569733, 6.018569869498933578 ) ) ;
#5472=CARTESIAN_POINT ( 'NONE',  ( 15.25711736267466812, 12.95927645368826298, 7.500898271101006820 ) ) ;
#5474=CARTESIAN_POINT ( 'NONE',  ( 16.19384365167809392, -5.424445124423267650, 6.782048567692550378 ) ) ;
#5477=DIRECTION ( 'NONE',  ( 1.000000000000000000, 0.000000000000000000, 0.000000000000000000 ) ) ;
#5478=ORIENTED_EDGE ( 'NONE', *, *, #24996, .F. ) ;
#5480=B_SPLINE_CURVE_WITH_KNOTS ( 'NONE', 3,
 ( #17009, #26530, #18631, #19508, #10002, #29020, #20943, #21997, #4435, #21845, #5007, #12182, #21679, #7358, #2822, #14667 ),
 .UNSPECIFIED., .F., .F.,
 ( 4, 2, 2, 2, 2, 2, 2, 4 ),
 ( 0.5000000000000000000, 0.6250000000000014433, 0.6875000000000021094, 0.7187500000000024425, 0.7500000000000028866, 0.8125000000000018874, 0.8750000000000008882, 1.000000000000000000 ),
 .UNSPECIFIED. ) ;
#5485=CARTESIAN_POINT ( 'NONE',  ( 9.326937650406419422, -14.24778824691897050, 20.12545155307891065 ) ) ;
#5487=VERTEX_POINT ( 'NONE', #26904 ) ;
#5489=AXIS2_PLACEMENT_3D ( 'NONE', #311, #19351, #28406 ) ;
#5490=CARTESIAN_POINT ( 'NONE',  ( -13.65791587866002388, 10.22062306005669541, 20.25542030744407640 ) ) ;
#5491=CARTESIAN_POINT ( 'NONE',  ( 5.291486201320592997, 19.28729773841935469, 5.652196082369963293 ) ) ;
#5492=VERTEX_POINT ( 'NONE', #12403 ) ;
#5495=CARTESIAN_POINT ( 'NONE',  ( -15.34618562042307843, 12.82554431217322310, 18.34798005863227388 ) ) ;
#5501=ORIENTED_EDGE ( 'NONE', *, *, #19304, .T. ) ;
#5504=ORIENTED_EDGE ( 'NONE', *, *, #29254, .T. ) ;
#5505=EDGE_LOOP ( 'NONE', ( #7577, #18196, #6030, #2181 ) ) ;
#5506=CYLINDRICAL_SURFACE ( 'NONE', #30209, 20.00000000000000000 ) ;
#5507=VERTEX_POINT ( 'NONE', #12557 ) ;
#5513=CARTESIAN_POINT ( 'NONE',  ( -9.436481611552759219, -0.9307681286968216838, 21.50000000000000000 ) ) ;
#5516=ADVANCED_FACE ( 'NONE', ( #17382 ), #17219, .F. ) ;
#5517=CARTESIAN_POINT ( 'NONE',  ( -11.35972605147146020, -16.46076013017339434, 6.518927109361845496 ) ) ;
#5518=DIRECTION ( 'NONE',  ( 1.000000000000000000, 0.000000000000000000, 0.000000000000000000 ) ) ;
#5519=CYLINDRICAL_SURFACE ( 'NONE', #18222, 20.00000000000000355 ) ;
#5522=CARTESIAN_POINT ( 'NONE',  ( -11.29739510359497423, -16.52539200402570785, 19.77662771831109367 ) ) ;
#5524=CARTESIAN_POINT ( 'NONE',  ( -5.870757325077154754, 16.01346137069357667, 5.704143890883081269 ) ) ;
#5525=CARTESIAN_POINT ( 'NONE',  ( 11.77505735701808121, -16.18809529858903318, 6.041646659195333058 ) ) ;
#5529=VECTOR ( 'NONE', #19949, 1000.000000000000000 ) ;
#5534=CARTESIAN_POINT ( 'NONE',  ( -5.027435569059560905, 19.35787894679205934, 19.08232364404840098 ) ) ;
#5536=CARTESIAN_POINT ( 'NONE',  ( 1.195154792889395079, 9.406652940105990623, 21.50000000000000000 ) ) ;
#5537=ORIENTED_EDGE ( 'NONE', *, *, #8603, .F. ) ;
#5542=CARTESIAN_POINT ( 'NONE',  ( 5.409330662328859063, 19.27307614344555020, 18.35377592296120497 ) ) ;
#5547=CARTESIAN_POINT ( 'NONE',  ( -9.248129367672078160, -2.094186647214714814, 13.00000000000000178 ) ) ;
#5549=ADVANCED_FACE ( 'NONE', ( #12709 ), #11410, .T. ) ;
#5550=AXIS2_PLACEMENT_3D ( 'NONE', #6274, #15786, #25308 ) ;
#5560=AXIS2_PLACEMENT_3D ( 'NONE', #1012, #19886, #8038 ) ;
#5561=FACE_OUTER_BOUND ( 'NONE', #17940, .T. ) ;
#5566=EDGE_LOOP ( 'NONE', ( #17118, #10038, #16960, #17238 ) ) ;
#5568=VECTOR ( 'NONE', #25236, 1000.000000000000000 ) ;
#5569=CYLINDRICAL_SURFACE ( 'NONE', #7804, 20.00000000000000000 ) ;
#5570=CARTESIAN_POINT ( 'NONE',  ( 5.163176754322195805, 19.32250783072323230, 5.652912763329821288 ) ) ;
#5575=EDGE_CURVE ( 'NONE', #2154, #2241, #27201, .T. ) ;
#5579=AXIS2_PLACEMENT_3D ( 'NONE', #4312, #13393, #13843 ) ;
#5582=LINE ( 'NONE', #8080, #21121 ) ;
#5583=EDGE_CURVE ( 'NONE', #8511, #15390, #8142, .T. ) ;
#5588=EDGE_LOOP ( 'NONE', ( #24455, #3172, #6613, #24294 ) ) ;
#5589=DIRECTION ( 'NONE',  ( 0.9096319953545183301, 0.4154150130018864906, 0.000000000000000000 ) ) ;
#5590=VERTEX_POINT ( 'NONE', #5992 ) ;
#5592=CARTESIAN_POINT ( 'NONE',  ( -16.93068695967834358, 1.913742347823925938, 20.32222155561919053 ) ) ;
#5595=CARTESIAN_POINT ( 'NONE',  ( -6.453144054752233849, 18.93070788617553646, 20.22386025856690139 ) ) ;
#5596=EDGE_CURVE ( 'NONE', #27593, #19541, #22658, .T. ) ;
#5598=CARTESIAN_POINT ( 'NONE',  ( 16.57618148055193430, 4.095680178559270246, 7.098451512883313441 ) ) ;
#5603=CARTESIAN_POINT ( 'NONE',  ( -8.416592248870401249, -14.82768166143396193, 18.35718225375110180 ) ) ;
#5608=CARTESIAN_POINT ( 'NONE',  ( 10.83635815962788307, -16.83143582838889074, 5.701226463332907279 ) ) ;
#5610=DIRECTION ( 'NONE',  ( 0.000000000000000000, 0.000000000000000000, 1.000000000000000000 ) ) ;
#5614=CARTESIAN_POINT ( 'NONE',  ( 4.340342926364955112, 8.430595340551274575, 21.50000000000000000 ) ) ;
#5615=AXIS2_PLACEMENT_3D ( 'NONE', #22980, #20643, #8796 ) ;
#5616=CARTESIAN_POINT ( 'NONE',  ( 11.10715495309692891, -16.63223102436628409, 7.652108011868850035 ) ) ;
#5619=DIRECTION ( 'NONE',  ( -1.000000000000000000, 0.000000000000000000, 0.000000000000000000 ) ) ;
#5623=CARTESIAN_POINT ( 'NONE',  ( 5.783356563690326801, 19.14595685992715346, 7.526993102356318133 ) ) ;
#5636=DIRECTION ( 'NONE',  ( 0.000000000000000000, 0.000000000000000000, 1.000000000000000000 ) ) ;
#5639=DIRECTION ( 'NONE',  ( 0.000000000000000000, 0.000000000000000000, 1.000000000000000000 ) ) ;
#5642=CARTESIAN_POINT ( 'NONE',  ( 10.65605551513794680, -16.94611923951457300, 20.19668224736330941 ) ) ;
#5643=CARTESIAN_POINT ( 'NONE',  ( 10.36464550818150876, -17.10487384371581143, 18.84056766331482180 ) ) ;
#5646=CARTESIAN_POINT ( 'NONE',  ( -15.98601489809225740, 12.04791232832106118, 19.47783254395485031 ) ) ;
#5648=ORIENTED_EDGE ( 'NONE', *, *, #20619, .F. ) ;
#5651=B_SPLINE_SURFACE_WITH_KNOTS ( 'NONE', 3, 1, ( 
 ( #6319, #25350 ),
 ( #3988, #13511 ),
 ( #4131, #21574 ),
 ( #2240, #7399 ),
 ( #2565, #2406 ),
 ( #2716, #30622 ),
 ( #211, #24065 ),
 ( #18950, #19234 ),
 ( #9268, #23448 ),
 ( #7085, #28760 ),
 ( #9724, #18789 ),
 ( #12224, #25811 ),
 ( #16909, #11933 ),
 ( #9434, #21724 ),
 ( #28459, #16590 ),
 ( #26105, #26425 ),
 ( #66, #6935 ),
 ( #5054, #364 ),
 ( #4735, #21103 ),
 ( #14236, #2086 ),
 ( #9885, #28310 ),
 ( #11608, #4897 ),
 ( #19402, #11759 ),
 ( #28920, #7553 ),
 ( #4442, #13953 ),
 ( #16445, #25959 ),
 ( #21424, #9579 ),
 ( #23918, #14416 ),
 ( #4587, #14087 ),
 ( #23597, #21257 ),
 ( #30785, #19090 ) ),
 .UNSPECIFIED., .F., .F., .F.,
 ( 4, 3, 3, 3, 3, 3, 3, 3, 3, 3, 4 ),
 ( 2, 2 ),
 ( 0.4999999998345686647, 0.5360336730431939367, 0.5907651151589012883, 0.6456034593241830599, 0.6998270958050434309, 0.7529536536315937223, 0.8052385063053260073, 0.8575343587103997356, 0.9106564858195042023, 0.9648414833209685293, 1.000000006602610014 ),
 ( 0.000000000000000000, 1.000000000000000000 ),
 .UNSPECIFIED. ) ;
#5652=CARTESIAN_POINT ( 'NONE',  ( -15.34307810681595186, 12.82926163924265950, 20.34789198813115263 ) ) ;
#5654=FACE_OUTER_BOUND ( 'NONE', #7086, .T. ) ;
#5656=AXIS2_PLACEMENT_3D ( 'NONE', #28237, #2188, #6867 ) ;
#5659=CARTESIAN_POINT ( 'NONE',  ( 14.88222593340887023, 13.36111339922579866, 20.34789198813115263 ) ) ;
#5661=ORIENTED_EDGE ( 'NONE', *, *, #23269, .T. ) ;
#5664=ORIENTED_EDGE ( 'NONE', *, *, #20517, .T. ) ;
#5667=LINE ( 'NONE', #8167, #21228 ) ;
#5668=DIRECTION ( 'NONE',  ( 0.000000000000000000, 0.000000000000000000, 1.000000000000000000 ) ) ;
#5672=AXIS2_PLACEMENT_3D ( 'NONE', #22092, #25526, #18359 ) ;
#5673=DIRECTION ( 'NONE',  ( 0.000000000000000000, 0.000000000000000000, -1.000000000000000000 ) ) ;
#5674=FACE_OUTER_BOUND ( 'NONE', #21417, .T. ) ;
#5675=CYLINDRICAL_SURFACE ( 'NONE', #17626, 0.7500000000000006661 ) ;
#5677=AXIS2_PLACEMENT_3D ( 'NONE', #18237, #27758, #4040 ) ;
#5678=CARTESIAN_POINT ( 'NONE',  ( -14.84326473672823887, -8.425446036094902169, 7.366751648393900176 ) ) ;
#5679=CARTESIAN_POINT ( 'NONE',  ( -5.062693764981381683, 16.26276758967398095, 5.774779864094945481 ) ) ;
#5680=CARTESIAN_POINT ( 'NONE',  ( 11.70583205457081810, -16.23839729645239416, 7.366751648393900176 ) ) ;
#5687=CARTESIAN_POINT ( 'NONE',  ( -15.33339156390900371, 12.86857621502489479, 5.651989602109218858 ) ) ;
#5691=CARTESIAN_POINT ( 'NONE',  ( 3.062271323958281499, 16.80150817659524520, 6.783738457429056012 ) ) ;
#5696=DIRECTION ( 'NONE',  ( 1.000000000000000000, 0.000000000000000000, 0.000000000000000000 ) ) ;
#5700=ADVANCED_FACE ( 'NONE', ( #20778 ), #6748, .F. ) ;
#5703=ORIENTED_EDGE ( 'NONE', *, *, #12646, .F. ) ;
#5704=CARTESIAN_POINT ( 'NONE',  ( -18.09182123201595971, -8.567353834808582036, 5.653912893140659257 ) ) ;
#5706=CARTESIAN_POINT ( 'NONE',  ( 15.91946090795792657, -6.118695898272386025, 5.653604225791664106 ) ) ;
#5710=CARTESIAN_POINT ( 'NONE',  ( 0.000000000000000000, 0.000000000000000000, 1.500000000000001332 ) ) ;
#5713=DIRECTION ( 'NONE',  ( 1.000000000000000000, 0.000000000000000000, 0.000000000000000000 ) ) ;
#5717=ORIENTED_EDGE ( 'NONE', *, *, #16017, .F. ) ;
#5723=CARTESIAN_POINT ( 'NONE',  ( 12.50580948684386051, 11.57370347876661221, 18.36582235739946611 ) ) ;
#5725=VERTEX_POINT ( 'NONE', #25929 ) ;
#5729=CARTESIAN_POINT ( 'NONE',  ( 17.92197892105642154, -8.877232523309842804, 6.386539667786092167 ) ) ;
#5732=ORIENTED_EDGE ( 'NONE', *, *, #5782, .T. ) ;
#5734=CIRCLE ( 'NONE', #17196, 9.482273699623480212 ) ;
#5735=ADVANCED_FACE ( 'NONE', ( #16114 ), #15966, .F. ) ;
#5736=ORIENTED_EDGE ( 'NONE', *, *, #12838, .T. ) ;
#5738=CARTESIAN_POINT ( 'NONE',  ( -16.83599852035921884, 2.522587596188540449, 18.83976166372255534 ) ) ;
#5740=CARTESIAN_POINT ( 'NONE',  ( -6.934930584103120133, 18.75917743548997763, 19.21940439362674269 ) ) ;
#5743=CARTESIAN_POINT ( 'NONE',  ( 19.65054205152827649, 3.817440173033142425, 7.441806358946449151 ) ) ;
#5746=CARTESIAN_POINT ( 'NONE',  ( -9.668922248712513934, -17.52764785324847452, 19.58863275299554019 ) ) ;
#5747=ADVANCED_FACE ( 'NONE', ( #25636 ), #4251, .F. ) ;
#5750=LINE ( 'NONE', #1392, #14847 ) ;
#5752=CARTESIAN_POINT ( 'NONE',  ( 10.51735345234056851, -17.03234025559531162, 5.940635272151477686 ) ) ;
#5759=DIRECTION ( 'NONE',  ( 0.000000000000000000, 0.000000000000000000, -1.000000000000000000 ) ) ;
#5765=EDGE_CURVE ( 'NONE', #29085, #3383, #9699, .T. ) ;
#5766=LINE ( 'NONE', #7970, #2959 ) ;
#5770=CARTESIAN_POINT ( 'NONE',  ( -10.28466407052217235, -17.15343732189304404, 18.37545668562167478 ) ) ;
#5771=DIRECTION ( 'NONE',  ( -0.000000000000000000, -0.000000000000000000, 1.000000000000000000 ) ) ;
#5772=CARTESIAN_POINT ( 'NONE',  ( 19.77948086832033425, 3.081792779576176589, 7.652108011868850035 ) ) ;
#5777=EDGE_CURVE ( 'NONE', #28158, #23071, #9569, .T. ) ;
#5782=EDGE_CURVE ( 'NONE', #14763, #13104, #27016, .T. ) ;
#5783=CARTESIAN_POINT ( 'NONE',  ( 4.606472074292932817, 19.48056636435423528, 7.366751648393900176 ) ) ;
#5785=CARTESIAN_POINT ( 'NONE',  ( 5.422617586916729238, 19.25129646183502174, 20.34789198813115618 ) ) ;
#5789=CARTESIAN_POINT ( 'NONE',  ( 10.26788185420488375, -17.18392197670719312, 19.22654678686458141 ) ) ;
#5793=CARTESIAN_POINT ( 'NONE',  ( -13.91614452448632555, 9.890357823660679060, 19.89182036555910571 ) ) ;
#5800=DIRECTION ( 'NONE',  ( -1.000000000000000000, 0.000000000000000000, 0.000000000000000000 ) ) ;
#5802=CARTESIAN_POINT ( 'NONE',  ( -15.25895845836713072, 12.92986402562787696, 20.34789198813115618 ) ) ;
#5806=CARTESIAN_POINT ( 'NONE',  ( -7.827050521741844236, 5.352643706120543854, 13.00000000000000178 ) ) ;
#5807=AXIS2_PLACEMENT_3D ( 'NONE', #3152, #24976, #19836 ) ;
#5808=CARTESIAN_POINT ( 'NONE',  ( 16.86493654370565665, 2.320966539639655490, 7.156916968540300239 ) ) ;
#5813=DIRECTION ( 'NONE',  ( 0.000000000000000000, 0.000000000000000000, -1.000000000000000000 ) ) ;
#5818=CIRCLE ( 'NONE', #15257, 0.7500000000000006661 ) ;
#5826=DIRECTION ( 'NONE',  ( -0.000000000000000000, -0.000000000000000000, -1.000000000000000000 ) ) ;
#5828=CARTESIAN_POINT ( 'NONE',  ( -8.549050687778191104, -4.102102735472429096, 13.00000000000000178 ) ) ;
#5831=DIRECTION ( 'NONE',  ( -0.000000000000000000, -0.000000000000000000, 1.000000000000000000 ) ) ;
#5833=AXIS2_PLACEMENT_3D ( 'NONE', #26308, #4944, #9771 ) ;
#5835=CARTESIAN_POINT ( 'NONE',  ( -8.744978663125428042, -14.62407600317563272, 20.32842677360128292 ) ) ;
#5837=CARTESIAN_POINT ( 'NONE',  ( -17.75446986341067301, 9.207540381081360081, 24.50000000000000000 ) ) ;
#5838=CARTESIAN_POINT ( 'NONE',  ( 11.76322808224952254, -16.19669642467957615, 7.280727868105637768 ) ) ;
#5839=EDGE_CURVE ( 'NONE', #4843, #18506, #27282, .T. ) ;
#5842=VECTOR ( 'NONE', #14495, 1000.000000000000000 ) ;
#5843=EDGE_LOOP ( 'NONE', ( #43, #18790, #29373, #22465 ) ) ;
#5847=CARTESIAN_POINT ( 'NONE',  ( -15.21204208253569412, 13.01227270423824045, 5.670038381137163519 ) ) ;
#5858=CARTESIAN_POINT ( 'NONE',  ( 11.33091155972628350, -16.48105488812122488, 5.679672709359370408 ) ) ;
#5862=CARTESIAN_POINT ( 'NONE',  ( -19.71415773217921696, 3.369653345580893689, 19.85261563089511938 ) ) ;
#5864=ORIENTED_EDGE ( 'NONE', *, *, #28978, .T. ) ;
#5867=FACE_OUTER_BOUND ( 'NONE', #8602, .T. ) ;
#5870=CIRCLE ( 'NONE', #19799, 0.7500000000000006661 ) ;
#5874=VERTEX_POINT ( 'NONE', #336 ) ;
#5877=ORIENTED_EDGE ( 'NONE', *, *, #24461, .F. ) ;
#5878=ORIENTED_EDGE ( 'NONE', *, *, #25979, .T. ) ;
#5879=FACE_OUTER_BOUND ( 'NONE', #20137, .T. ) ;
#5881=CARTESIAN_POINT ( 'NONE',  ( 1.687027447297431371, 8.840471615930075799, 1.500000000000001332 ) ) ;
#5890=CARTESIAN_POINT ( 'NONE',  ( 18.38084888341871093, -7.928499866610144942, 20.34789198813115263 ) ) ;
#5891=CARTESIAN_POINT ( 'NONE',  ( -4.163336342344337027E-14, 1.387778780781445676E-14, 1.500000000000000000 ) ) ;
#5892=VECTOR ( 'NONE', #15518, 1000.000000000000000 ) ;
#5895=CARTESIAN_POINT ( 'NONE',  ( -4.773373620122390193, 16.34284820694567486, 18.72771030977187579 ) ) ;
#5896=VERTEX_POINT ( 'NONE', #26230 ) ;
#5898=ORIENTED_EDGE ( 'NONE', *, *, #1710, .F. ) ;
#5900=AXIS2_PLACEMENT_3D ( 'NONE', #3425, #10446, #5462 ) ;
#5902=CARTESIAN_POINT ( 'NONE',  ( 16.58472157312809259, 4.055073576757204812, 6.131018562779544823 ) ) ;
#5903=CARTESIAN_POINT ( 'NONE',  ( -15.00589365688690435, 13.24944937571967962, 18.49267272388512140 ) ) ;
#5906=CARTESIAN_POINT ( 'NONE',  ( -7.931808866138725378, -15.11281102451791547, 20.06253562465620632 ) ) ;
#5908=CARTESIAN_POINT ( 'NONE',  ( -19.62935297797563905, -3.832558109936532897, 24.50000000000000000 ) ) ;
#5909=CARTESIAN_POINT ( 'NONE',  ( -19.91230480659700319, 2.053870633397347323, 18.44527579819791185 ) ) ;
#5913=CARTESIAN_POINT ( 'NONE',  ( 11.24508296785401917, -16.56092475412858889, 18.35718225375110180 ) ) ;
#5914=AXIS2_PLACEMENT_3D ( 'NONE', #13375, #30048, #15072 ) ;
#5916=VERTEX_POINT ( 'NONE', #7372 ) ;
#5917=EDGE_LOOP ( 'NONE', ( #27094, #348, #5878, #19538 ) ) ;
#5918=CARTESIAN_POINT ( 'NONE',  ( 18.28487737789067324, -8.104377114558884543, 18.34726407865098707 ) ) ;
#5921=DIRECTION ( 'NONE',  ( 1.000000000000000000, 0.000000000000000000, 0.000000000000000000 ) ) ;
#5922=EDGE_LOOP ( 'NONE', ( #5864, #16546, #15139, #199 ) ) ;
#5924=DIRECTION ( 'NONE',  ( 1.000000000000000000, 0.000000000000000000, 0.000000000000000000 ) ) ;
#5925=DIRECTION ( 'NONE',  ( 0.000000000000000000, 1.000000000000000000, 0.000000000000000000 ) ) ;
#5930=CARTESIAN_POINT ( 'NONE',  ( 12.20325286834225942, 11.91007939804258875, 5.678370764302467677 ) ) ;
#5931=AXIS2_PLACEMENT_3D ( 'NONE', #3778, #8614, #27341 ) ;
#5932=CARTESIAN_POINT ( 'NONE',  ( 19.88037316481945282, 2.342382300094909553, 7.176035686813569292 ) ) ;
#5934=EDGE_CURVE ( 'NONE', #5507, #24431, #22542, .T. ) ;
#5935=CARTESIAN_POINT ( 'NONE',  ( 14.97043017101258400, 13.28903844302880444, 5.657991946698900598 ) ) ;
#5936=ORIENTED_EDGE ( 'NONE', *, *, #16826, .T. ) ;
#5937=CARTESIAN_POINT ( 'NONE',  ( 9.471281197126602436, 0.4564504349074720024, 21.50000000000000000 ) ) ;
#5939=ORIENTED_EDGE ( 'NONE', *, *, #5951, .T. ) ;
#5940=AXIS2_PLACEMENT_3D ( 'NONE', #18280, #30574, #21051 ) ;
#5942=CARTESIAN_POINT ( 'NONE',  ( 4.592382419210019329, 19.48389062382846504, 5.951255046771932733 ) ) ;
#5950=ORIENTED_EDGE ( 'NONE', *, *, #4110, .T. ) ;
#5951=EDGE_CURVE ( 'NONE', #28288, #984, #19565, .T. ) ;
#5952=CARTESIAN_POINT ( 'NONE',  ( 9.471281197126604212, 0.4564504349074710587, 1.500000000000001332 ) ) ;
#5953=CARTESIAN_POINT ( 'NONE',  ( 15.58729175431055047, -6.863221649612943231, 7.500898271101006820 ) ) ;
#5954=CARTESIAN_POINT ( 'NONE',  ( -14.00963640524698306, 9.767049959719264152, 19.47783254395485031 ) ) ;
#5957=DIRECTION ( 'NONE',  ( -0.4154150130018972598, -0.9096319953545133341, 0.000000000000000000 ) ) ;
#5959=EDGE_CURVE ( 'NONE', #15686, #3764, #24621, .T. ) ;
#5961=EDGE_CURVE ( 'NONE', #6583, #1130, #27443, .T. ) ;
#5962=CARTESIAN_POINT ( 'NONE',  ( -5.025762778208110682, 19.37674427759095863, 19.56050940960062690 ) ) ;
#5964=DIRECTION ( 'NONE',  ( -1.000000000000000000, 0.000000000000000000, 0.000000000000000000 ) ) ;
#5966=DIRECTION ( 'NONE',  ( 1.000000000000000000, 0.000000000000000000, 0.000000000000000000 ) ) ;
#5968=EDGE_CURVE ( 'NONE', #21915, #16485, #30511, .T. ) ;
#5975=CARTESIAN_POINT ( 'NONE',  ( -19.72722132040463450, 3.293256439147198122, 6.033082186765059696 ) ) ;
#5976=CARTESIAN_POINT ( 'NONE',  ( -19.91205802435384697, 1.875831072725641313, 18.54958172136248251 ) ) ;
#5982=CARTESIAN_POINT ( 'NONE',  ( -5.978582532085236600, 19.10413086404602723, 18.34798005862662507 ) ) ;
#5984=DIRECTION ( 'NONE',  ( 0.000000000000000000, 0.000000000000000000, -1.000000000000000000 ) ) ;
#5985=CARTESIAN_POINT ( 'NONE',  ( 14.59923040764597957, 13.69601292063889275, 20.25542030744407640 ) ) ;
#5986=EDGE_CURVE ( 'NONE', #16618, #24186, #19544, .T. ) ;
#5987=ORIENTED_EDGE ( 'NONE', *, *, #4231, .T. ) ;
#5989=CIRCLE ( 'NONE', #9463, 9.482273699623480212 ) ;
#5990=CARTESIAN_POINT ( 'NONE',  ( 0.000000000000000000, 0.000000000000000000, 21.50000000000000000 ) ) ;
#5992=CARTESIAN_POINT ( 'NONE',  ( 9.406652940105985294, -1.195154792889423057, 21.50000000000000000 ) ) ;
#5993=CARTESIAN_POINT ( 'NONE',  ( 10.45210396439254197, -13.49311571392157028, 7.366751648393900176 ) ) ;
#5997=ORIENTED_EDGE ( 'NONE', *, *, #11106, .F. ) ;
#6000=DIRECTION ( 'NONE',  ( 1.000000000000000000, 0.000000000000000000, 0.000000000000000000 ) ) ;
#6013=ADVANCED_FACE ( 'NONE', ( #14618 ), #16654, .F. ) ;
#6014=CYLINDRICAL_SURFACE ( 'NONE', #4371, 20.00000000000000000 ) ;
#6017=CARTESIAN_POINT ( 'NONE',  ( 12.35522425158188931, 11.74279415389956327, 18.34798005863078885 ) ) ;
#6024=FACE_OUTER_BOUND ( 'NONE', #7908, .T. ) ;
#6025=ORIENTED_EDGE ( 'NONE', *, *, #5099, .T. ) ;
#6026=CARTESIAN_POINT ( 'NONE',  ( 9.051788058582081575, -14.41610800086747801, 6.973843882838225205 ) ) ;
#6028=CARTESIAN_POINT ( 'NONE',  ( -8.546423435383418976, -14.74799740001549786, 18.34798005863078885 ) ) ;
#6029=ORIENTED_EDGE ( 'NONE', *, *, #266, .T. ) ;
#6030=ORIENTED_EDGE ( 'NONE', *, *, #14679, .T. ) ;
#6035=VERTEX_POINT ( 'NONE', #21472 ) ;
#6036=CARTESIAN_POINT ( 'NONE',  ( -6.047835543816287185, 15.95440705816254479, 18.45571264222803975 ) ) ;
#6037=CARTESIAN_POINT ( 'NONE',  ( 9.436006877715755081, -14.17980878084792629, 20.22273502201483808 ) ) ;
#6038=EDGE_LOOP ( 'NONE', ( #25329, #3027, #16141, #23402 ) ) ;
#6041=CARTESIAN_POINT ( 'NONE',  ( 19.73705937795079635, 3.341332093703275330, 20.33971507717571114 ) ) ;
#6042=AXIS2_PLACEMENT_3D ( 'NONE', #1345, #20667, #10863 ) ;
#6046=CARTESIAN_POINT ( 'NONE',  ( -4.623640074040875625, 16.38233772743891947, 19.66962785902261857 ) ) ;
#6051=CARTESIAN_POINT ( 'NONE',  ( 14.87898187659695992, 13.36471393577513389, 18.34798005863227388 ) ) ;
#6056=CARTESIAN_POINT ( 'NONE',  ( 1.047421501149297329, -17.02264912680942643, 5.653604225791661442 ) ) ;
#6057=CARTESIAN_POINT ( 'NONE',  ( -16.99797872337576266, 1.390050218429698115, 20.34789198813115263 ) ) ;
#6058=CARTESIAN_POINT ( 'NONE',  ( -8.658642352887948590, -14.67867993418359340, 5.651492010659114662 ) ) ;
#6059=LINE ( 'NONE', #30227, #2907 ) ;
#6060=EDGE_LOOP ( 'NONE', ( #29299, #30194, #5717, #15131 ) ) ;
#6063=CIRCLE ( 'NONE', #18518, 9.482273699623480212 ) ;
#6064=CARTESIAN_POINT ( 'NONE',  ( -19.84403786039537465, 2.492757843112275218, 18.34798005863227388 ) ) ;
#6065=ORIENTED_EDGE ( 'NONE', *, *, #7292, .T. ) ;
#6069=CARTESIAN_POINT ( 'NONE',  ( -4.721574378597743760, 16.35655934831870795, 6.111214848085761986 ) ) ;
#6072=CARTESIAN_POINT ( 'NONE',  ( 9.864937699929955173, -13.90063973435163724, 5.652196082368482699 ) ) ;
#6077=CARTESIAN_POINT ( 'NONE',  ( 14.66647055262614785, 13.62412221374329846, 5.704143890883081269 ) ) ;
#6078=CARTESIAN_POINT ( 'NONE',  ( 19.79578860058543910, 2.975267875541940832, 5.670038381137163519 ) ) ;
#6080=CYLINDRICAL_SURFACE ( 'NONE', #8860, 0.7500000000000006661 ) ;
#6081=CARTESIAN_POINT ( 'NONE',  ( -13.88720712124151468, 9.928229803686351218, 18.73314399819311760 ) ) ;
#6082=CIRCLE ( 'NONE', #28990, 0.7500000000000006661 ) ;
#6084=EDGE_LOOP ( 'NONE', ( #19487, #14226, #1883, #22909 ) ) ;
#6086=CARTESIAN_POINT ( 'NONE',  ( 3.077027262763125215, 16.79827892558873970, 6.447548852708279377 ) ) ;
#6089=CARTESIAN_POINT ( 'NONE',  ( 6.070111251556830290, 19.05682731086504944, 19.96302680909623817 ) ) ;
#6091=CARTESIAN_POINT ( 'NONE',  ( 9.025811419443954264, -14.43167044742871497, 19.11611934778430921 ) ) ;
#6092=CARTESIAN_POINT ( 'NONE',  ( 16.09518941752841670, 6.251081041772567737, 1.500000000000000000 ) ) ;
#6093=ORIENTED_EDGE ( 'NONE', *, *, #20279, .F. ) ;
#6096=CARTESIAN_POINT ( 'NONE',  ( 18.13085077595200190, -8.485104792618537672, 5.796888747622817029 ) ) ;
#6097=CARTESIAN_POINT ( 'NONE',  ( -13.92530307126622802, 9.878387810998203733, 18.82680253904184298 ) ) ;
#6098=FACE_OUTER_BOUND ( 'NONE', #788, .T. ) ;
#6100=ORIENTED_EDGE ( 'NONE', *, *, #28425, .F. ) ;
#6103=CARTESIAN_POINT ( 'NONE',  ( -5.147812317479953492, 19.34466387292044232, 19.87181966307587544 ) ) ;
#6104=CARTESIAN_POINT ( 'NONE',  ( -2.523760598493608232, -1.621922452366769907, 24.50000000000000000 ) ) ;
#6106=CARTESIAN_POINT ( 'NONE',  ( 0.000000000000000000, 0.000000000000000000, 21.50000000000000000 ) ) ;
#6108=EDGE_CURVE ( 'NONE', #9077, #4023, #28509, .T. ) ;
#6113=VECTOR ( 'NONE', #22834, 1000.000000000000227 ) ;
#6114=VECTOR ( 'NONE', #26857, 1000.000000000000227 ) ;
#6116=ORIENTED_EDGE ( 'NONE', *, *, #5839, .T. ) ;
#6117=DIRECTION ( 'NONE',  ( 1.000000000000000000, 0.000000000000000000, 0.000000000000000000 ) ) ;
#6120=CARTESIAN_POINT ( 'NONE',  ( -8.637616862297813114, 3.912171961292039590, 13.00000000000000178 ) ) ;
#6121=ORIENTED_EDGE ( 'NONE', *, *, #24601, .F. ) ;
#6125=EDGE_CURVE ( 'NONE', #22613, #19044, #7921, .T. ) ;
#6129=CARTESIAN_POINT ( 'NONE',  ( 4.340342926364956888, 8.430595340551274575, 1.500000000000001332 ) ) ;
#6133=ORIENTED_EDGE ( 'NONE', *, *, #2115, .T. ) ;
#6134=EDGE_CURVE ( 'NONE', #13976, #15490, #19451, .T. ) ;
#6135=CARTESIAN_POINT ( 'NONE',  ( -11.05774036494470103, -16.68675304545164195, 18.55820869691756769 ) ) ;
#6137=CARTESIAN_POINT ( 'NONE',  ( -5.755751318732963639, 16.05090033862148857, 7.627891251804737927 ) ) ;
#6138=ADVANCED_FACE ( 'NONE', ( #10407 ), #12596, .T. ) ;
#6140=CARTESIAN_POINT ( 'NONE',  ( -14.80332652839582863, -8.501125445468646902, 18.73743063545763121 ) ) ;
#6148=CIRCLE ( 'NONE', #21562, 9.482273699623480212 ) ;
#6149=CARTESIAN_POINT ( 'NONE',  ( -14.79144470604038375, 13.48820156989937047, 6.111214848085761986 ) ) ;
#6152=CARTESIAN_POINT ( 'NONE',  ( 4.049916833591940879, 16.55712665779027049, 7.652108011868850923 ) ) ;
#6154=CARTESIAN_POINT ( 'NONE',  ( -8.579043560828052861, -14.72784502467623291, 5.651989602109218858 ) ) ;
#6157=EDGE_CURVE ( 'NONE', #6669, #10785, #9105, .T. ) ;
#6158=B_SPLINE_SURFACE_WITH_KNOTS ( 'NONE', 3, 1, ( 
 ( #13509, #22991 ),
 ( #20362, #20657 ),
 ( #13661, #29887 ),
 ( #23143, #30331 ),
 ( #18487, #27991 ),
 ( #16139, #25654 ),
 ( #4272, #2714 ),
 ( #4894, #23751 ),
 ( #16907, #4733 ),
 ( #16443, #24063 ),
 ( #9882, #362 ),
 ( #19400, #11930 ),
 ( #12221, #2403 ),
 ( #21571, #6932 ),
 ( #21101, #2083 ),
 ( #21421, #26423 ),
 ( #25956, #21722 ),
 ( #21254, #9266 ),
 ( #28918, #28307 ),
 ( #23595, #23446 ),
 ( #14565, #16289 ),
 ( #9722, #5052 ),
 ( #7081, #25808 ),
 ( #64, #7227 ),
 ( #18948, #7397 ),
 ( #2238, #16588 ),
 ( #9576, #19087 ),
 ( #12076, #4439 ),
 ( #11606, #28457 ),
 ( #30619, #11757 ),
 ( #4584, #14085 ) ),
 .UNSPECIFIED., .F., .F., .F.,
 ( 4, 3, 3, 3, 3, 3, 3, 3, 3, 3, 4 ),
 ( 2, 2 ),
 ( 0.4999999998345686092, 0.5360336730431942698, 0.5907651151589017324, 0.6456034593241839481, 0.6998270958050443191, 0.7529536536315944995, 0.8052385063053264513, 0.8575343587103996246, 0.9106564858195047574, 0.9648414833209688624, 1.000000006602610014 ),
 ( 0.000000000000000000, 1.000000000000000000 ),
 .UNSPECIFIED. ) ;
#6166=AXIS2_PLACEMENT_3D ( 'NONE', #3941, #20148, #29978 ) ;
#6169=DIRECTION ( 'NONE',  ( 1.000000000000000000, 0.000000000000000000, 0.000000000000000000 ) ) ;
#6171=ORIENTED_EDGE ( 'NONE', *, *, #14771, .T. ) ;
#6174=CARTESIAN_POINT ( 'NONE',  ( 16.18505772753977823, -5.447928388670486122, 6.917457548096561659 ) ) ;
#6176=DIRECTION ( 'NONE',  ( -1.000000000000000000, 0.000000000000000000, 0.000000000000000000 ) ) ;
#6181=DIRECTION ( 'NONE',  ( -0.7557495743542579358, 0.6548607339452854337, -0.000000000000000000 ) ) ;
#6188=CYLINDRICAL_SURFACE ( 'NONE', #23089, 20.00000000000000355 ) ;
#6192=EDGE_CURVE ( 'NONE', #7470, #18090, #5090, .T. ) ;
#6194=CARTESIAN_POINT ( 'NONE',  ( 11.11118388262826784, -16.62953976291649028, 18.34798005863226678 ) ) ;
#6195=EDGE_LOOP ( 'NONE', ( #9343, #21599 ) ) ;
#6197=CARTESIAN_POINT ( 'NONE',  ( -19.85166970746585946, 2.573860339590178903, 5.653912893140659257 ) ) ;
#6198=DIRECTION ( 'NONE',  ( -0.000000000000000000, -0.000000000000000000, 1.000000000000000000 ) ) ;
#6199=CARTESIAN_POINT ( 'NONE',  ( 15.45572804192159211, 12.69342571624615523, 6.144783687052517429 ) ) ;
#6202=CARTESIAN_POINT ( 'NONE',  ( -12.24063095261064227, 4.490763173670005770, 1.500000000000001332 ) ) ;
#6204=CYLINDRICAL_SURFACE ( 'NONE', #5579, 0.7499999999999997780 ) ;
#6208=CIRCLE ( 'NONE', #23615, 0.7500000000000002220 ) ;
#6211=CARTESIAN_POINT ( 'NONE',  ( 16.55849529797291098, 4.179294809495486263, 6.447548852708279377 ) ) ;
#6212=CARTESIAN_POINT ( 'NONE',  ( -13.02951369420309646, 10.96858531083378985, 18.49267272388512140 ) ) ;
#6213=CARTESIAN_POINT ( 'NONE',  ( -7.870033247355587847, -15.14769711951102771, 19.97651184436794125 ) ) ;
#6214=CARTESIAN_POINT ( 'NONE',  ( 12.72536390617885438, -2.839914339433650348, 24.50000000000000000 ) ) ;
#6215=CARTESIAN_POINT ( 'NONE',  ( -19.87987511945007313, 2.346632672767393402, 18.35718225375110180 ) ) ;
#6216=DIRECTION ( 'NONE',  ( -0.000000000000000000, -0.000000000000000000, 1.000000000000000000 ) ) ;
#6224=CARTESIAN_POINT ( 'NONE',  ( -5.439684697860721840, 16.15075171424584610, 5.657991946698900598 ) ) ;
#6225=ORIENTED_EDGE ( 'NONE', *, *, #11907, .F. ) ;
#6228=EDGE_CURVE ( 'NONE', #29559, #606, #26794, .T. ) ;
#6233=CARTESIAN_POINT ( 'NONE',  ( 11.85823002435686924, 12.27640118502221256, 5.951255046771932733 ) ) ;
#6234=CARTESIAN_POINT ( 'NONE',  ( 16.74250592919980818, 3.198927888535953112, 5.652196082367002994 ) ) ;
#6238=CARTESIAN_POINT ( 'NONE',  ( -14.01114995435608890, 9.765040422203625781, 19.28454053338348473 ) ) ;
#6239=VERTEX_POINT ( 'NONE', #22087 ) ;
#6240=ORIENTED_EDGE ( 'NONE', *, *, #1382, .F. ) ;
#6241=CARTESIAN_POINT ( 'NONE',  ( 3.160432912108486203, 16.77963207014078861, 7.098451512883313441 ) ) ;
#6242=DIRECTION ( 'NONE',  ( 1.000000000000000000, 0.000000000000000000, 0.000000000000000000 ) ) ;
#6243=DIRECTION ( 'NONE',  ( 1.000000000000000000, 0.000000000000000000, 0.000000000000000000 ) ) ;
#6244=ORIENTED_EDGE ( 'NONE', *, *, #14740, .F. ) ;
#6245=VECTOR ( 'NONE', #8619, 1000.000000000000000 ) ;
#6247=CARTESIAN_POINT ( 'NONE',  ( 10.27954044202352968, -17.17695407163359533, 19.11611934778430921 ) ) ;
#6250=CARTESIAN_POINT ( 'NONE',  ( -19.71764211798356925, 3.454211555243456910, 19.66989035740801839 ) ) ;
#6251=CARTESIAN_POINT ( 'NONE',  ( 17.96497429814991875, -8.830595420483335900, 7.080843742048788414 ) ) ;
#6252=CARTESIAN_POINT ( 'NONE',  ( -14.00963640524697418, 9.767049959719264152, 6.782048567692550378 ) ) ;
#6253=CARTESIAN_POINT ( 'NONE',  ( 3.905960108394943564, 16.59621863701447708, 20.33971507717571114 ) ) ;
#6255=EDGE_LOOP ( 'NONE', ( #19790, #2644, #10684, #21349 ) ) ;
#6259=CARTESIAN_POINT ( 'NONE',  ( 12.76326067953069021, 11.27442216563262356, 5.848946451764563292 ) ) ;
#6261=CYLINDRICAL_SURFACE ( 'NONE', #14624, 9.482273699623480212 ) ;
#6262=AXIS2_PLACEMENT_3D ( 'NONE', #4024, #20993, #14132 ) ;
#6265=VERTEX_POINT ( 'NONE', #19750 ) ;
#6269=ORIENTED_EDGE ( 'NONE', *, *, #29385, .F. ) ;
#6274=CARTESIAN_POINT ( 'NONE',  ( 0.4269445148198864892, 2.969464325642835689, 24.50000000000000000 ) ) ;
#6281=AXIS2_PLACEMENT_3D ( 'NONE', #13357, #11472, #11166 ) ;
#6284=CARTESIAN_POINT ( 'NONE',  ( -16.81375614428661791, 2.649924382790501021, 6.519181285484531685 ) ) ;
#6289=CARTESIAN_POINT ( 'NONE',  ( -5.419526071979801074, 16.15737324486737947, 7.652108011868851811 ) ) ;
#6291=CARTESIAN_POINT ( 'NONE',  ( -18.05883735157482661, -8.636530476581221194, 18.34798005862662507 ) ) ;
#6301=EDGE_CURVE ( 'NONE', #11660, #1290, #28174, .T. ) ;
#6303=ORIENTED_EDGE ( 'NONE', *, *, #13371, .T. ) ;
#6304=DIRECTION ( 'NONE',  ( -0.000000000000000000, -0.000000000000000000, 1.000000000000000000 ) ) ;
#6306=CARTESIAN_POINT ( 'NONE',  ( -9.269489102446176076, -14.27959628656686597, 6.111214848085761986 ) ) ;
#6307=AXIS2_PLACEMENT_3D ( 'NONE', #23730, #3005, #14388 ) ;
#6308=ORIENTED_EDGE ( 'NONE', *, *, #23292, .T. ) ;
#6312=ORIENTED_EDGE ( 'NONE', *, *, #3093, .T. ) ;
#6319=CARTESIAN_POINT ( 'NONE',  ( 0.3541522971493302196, -20.01464067411590264, 18.34798005862662507 ) ) ;
#6321=CARTESIAN_POINT ( 'NONE',  ( 11.65972768484889954, 12.47873923859708079, 19.47952243369111258 ) ) ;
#6325=CARTESIAN_POINT ( 'NONE',  ( -15.52789627656017224, -6.978352780261414701, 19.85270094495842486 ) ) ;
#6328=DIRECTION ( 'NONE',  ( 0.9594929736144974797, -0.2817325568414297265, 0.000000000000000000 ) ) ;
#6330=EDGE_CURVE ( 'NONE', #22249, #540, #7613, .T. ) ;
#6332=CARTESIAN_POINT ( 'NONE',  ( 9.118789845666759319, -14.37574228026362988, 6.143977687428010093 ) ) ;
#6333=CARTESIAN_POINT ( 'NONE',  ( -9.369089179316107519, -14.21146650728099381, 19.60617949693493856 ) ) ;
#6339=DIRECTION ( 'NONE',  ( 0.1423148382732889461, 0.9898214418809321291, 0.000000000000000000 ) ) ;
#6340=CARTESIAN_POINT ( 'NONE',  ( -13.68208811019134785, -10.53240720452297374, 1.500000000000000000 ) ) ;
#6341=PLANE ( 'NONE',  #22365 ) ;
#6351=EDGE_LOOP ( 'NONE', ( #2530, #13783, #8315, #56, #1126, #30652, #565, #30623, #28984, #197, #7390, #13612, #25640, #20397, #1083, #13098, #8215, #1676, #26864, #777, #30251, #20777, #759, #6029, #10352, #20885, #18447, #8992, #3076, #28564, #13195, #19452, #4351, #17913, #20629, #20500, #2246, #6133, #26132, #9168, #3955, #15267, #26335, #28977, #24268, #20534, #29212, #14479, #12323, #26645, #11536, #16061, #28300, #29913, #7360, #3255, #16934, #17039, #84, #4215, #28043, #2160, #12284, #23345, #29390, #10462, #16670, #27598, #17689, #28149, #24749, #5939, #8617, #10057, #5987, #26763, #15662, #24701, #14294, #25511, #24121, #10588, #25111 ) ) ;
#6352=CARTESIAN_POINT ( 'NONE',  ( -16.85109579167143679, 2.433552959544808658, 6.018569869498933578 ) ) ;
#6359=ORIENTED_EDGE ( 'NONE', *, *, #17938, .T. ) ;
#6361=CARTESIAN_POINT ( 'NONE',  ( -14.76455652122660211, -8.574248774020551522, 6.147510495896840510 ) ) ;
#6363=EDGE_LOOP ( 'NONE', ( #30767, #20212, #3852, #420 ) ) ;
#6365=CIRCLE ( 'NONE', #26279, 1.000000000000004441 ) ;
#6366=CARTESIAN_POINT ( 'NONE',  ( 16.83292851409026980, 2.581421006622409031, 20.14907003336613300 ) ) ;
#6369=PLANE ( 'NONE',  #9618 ) ;
#6371=AXIS2_PLACEMENT_3D ( 'NONE', #19909, #29423, #27077 ) ;
#6372=CARTESIAN_POINT ( 'NONE',  ( 1.788804076111017549, -16.98411955790531991, 6.521906765011497242 ) ) ;
#6373=CARTESIAN_POINT ( 'NONE',  ( -16.96556290498877573, 1.647560670993253540, 18.34798005863078885 ) ) ;
#6377=EDGE_CURVE ( 'NONE', #17660, #26457, #26119, .T. ) ;
#6378=VECTOR ( 'NONE', #16777, 1000.000000000000000 ) ;
#6379=EDGE_CURVE ( 'NONE', #25657, #6669, #2579, .T. ) ;
#6385=FACE_OUTER_BOUND ( 'NONE', #25780, .T. ) ;
#6390=CARTESIAN_POINT ( 'NONE',  ( -13.05132497920473611, 10.94401179279875969, 5.774779864094943704 ) ) ;
#6396=CARTESIAN_POINT ( 'NONE',  ( 0.000000000000000000, 0.000000000000000000, 1.500000000000001332 ) ) ;
#6398=AXIS2_PLACEMENT_3D ( 'NONE', #3119, #12639, #22132 ) ;
#6401=ORIENTED_EDGE ( 'NONE', *, *, #22169, .T. ) ;
#6402=CARTESIAN_POINT ( 'NONE',  ( 3.085425824774463255, 16.79642356368105283, 6.892848776733236704 ) ) ;
#6409=CARTESIAN_POINT ( 'NONE',  ( 10.92986663323816465, -16.77091174116444350, 18.36582235739946611 ) ) ;
#6413=FACE_OUTER_BOUND ( 'NONE', #18578, .T. ) ;
#6414=CARTESIAN_POINT ( 'NONE',  ( -13.98072106069837517, 9.805336070574281138, 6.341840715582230281 ) ) ;
#6415=CARTESIAN_POINT ( 'NONE',  ( 3.122919890997783110, 16.78802993858287707, 19.69140814234746273 ) ) ;
#6421=CARTESIAN_POINT ( 'NONE',  ( 12.35522425158189108, 11.74279415389956505, 5.652196082368482699 ) ) ;
#6422=DIRECTION ( 'NONE',  ( 1.000000000000000000, 0.000000000000000000, 0.000000000000000000 ) ) ;
#6425=CIRCLE ( 'NONE', #2435, 9.482273699623480212 ) ;
#6427=CYLINDRICAL_SURFACE ( 'NONE', #6902, 0.7500000000000002220 ) ;
#6430=CARTESIAN_POINT ( 'NONE',  ( 0.9770435002939149571, -19.97634058022567771, 5.853797745100181693 ) ) ;
#6431=AXIS2_PLACEMENT_3D ( 'NONE', #28012, #6497, #23163 ) ;
#6432=CYLINDRICAL_SURFACE ( 'NONE', #8235, 0.7499999999999997780 ) ;
#6433=CARTESIAN_POINT ( 'NONE',  ( 0.000000000000000000, 0.000000000000000000, 1.500000000000001332 ) ) ;
#6436=EDGE_LOOP ( 'NONE', ( #30599, #14041 ) ) ;
#6437=CARTESIAN_POINT ( 'NONE',  ( -19.80980381183503525, 2.754394816484158515, 5.676722608126683056 ) ) ;
#6440=DIRECTION ( 'NONE',  ( 0.000000000000000000, 0.000000000000000000, 1.000000000000000000 ) ) ;
#6441=ORIENTED_EDGE ( 'NONE', *, *, #4973, .F. ) ;
#6442=CARTESIAN_POINT ( 'NONE',  ( -0.6573828633908590513, -19.98919327533015533, 6.781503518395075147 ) ) ;
#6451=CARTESIAN_POINT ( 'NONE',  ( -16.96556290498877573, 1.647560670993253540, 5.652196082368482699 ) ) ;
#6458=CARTESIAN_POINT ( 'NONE',  ( -15.01497154418443891, -8.089954645606729500, 18.39992786714538298 ) ) ;
#6463=CARTESIAN_POINT ( 'NONE',  ( -0.5282983270408734278, -19.99308596983832587, 18.84056766331481825 ) ) ;
#6466=DIRECTION ( 'NONE',  ( -0.000000000000000000, -0.000000000000000000, -1.000000000000000000 ) ) ;
#6471=VECTOR ( 'NONE', #6618, 1000.000000000000000 ) ;
#6474=ORIENTED_EDGE ( 'NONE', *, *, #14850, .F. ) ;
#6480=CARTESIAN_POINT ( 'NONE',  ( 11.75084321055936520, 12.38658771204268128, 18.84329447212444109 ) ) ;
#6481=LINE ( 'NONE', #28146, #29833 ) ;
#6483=EDGE_CURVE ( 'NONE', #17576, #8468, #20966, .T. ) ;
#6487=CARTESIAN_POINT ( 'NONE',  ( -6.778663211761418061, 6.630478080506979843, 13.00000000000000178 ) ) ;
#6488=CARTESIAN_POINT ( 'NONE',  ( -18.15587082468813307, -8.389233089038011570, 20.32243167357988156 ) ) ;
#6489=DIRECTION ( 'NONE',  ( -0.5406408174555976665, 0.8412535328311810945, 0.000000000000000000 ) ) ;
#6497=DIRECTION ( 'NONE',  ( -0.000000000000000000, -0.000000000000000000, 1.000000000000000000 ) ) ;
#6503=ORIENTED_EDGE ( 'NONE', *, *, #7707, .T. ) ;
#6504=CARTESIAN_POINT ( 'NONE',  ( -19.74686063004095971, 3.283826233409512074, 6.018569869498933578 ) ) ;
#6506=CARTESIAN_POINT ( 'NONE',  ( 14.96781329949620698, 13.26582956964654159, 5.651480102388687143 ) ) ;
#6508=ORIENTED_EDGE ( 'NONE', *, *, #1182, .T. ) ;
#6511=ORIENTED_EDGE ( 'NONE', *, *, #21639, .F. ) ;
#6520=CARTESIAN_POINT ( 'NONE',  ( 0.6650193650332598683, -17.02944248263315785, 7.652108011868850035 ) ) ;
#6524=CARTESIAN_POINT ( 'NONE',  ( -8.975220329042338463, -14.47597657772618085, 5.774779864094944593 ) ) ;
#6525=CARTESIAN_POINT ( 'NONE',  ( 14.87898187659696170, 13.36471393577513389, 5.652196082369963293 ) ) ;
#6526=ORIENTED_EDGE ( 'NONE', *, *, #10961, .F. ) ;
#6531=ORIENTED_EDGE ( 'NONE', *, *, #16033, .F. ) ;
#6534=LINE ( 'NONE', #22744, #12654 ) ;
#6536=CARTESIAN_POINT ( 'NONE',  ( -5.128149923613393391, 16.24357618101655021, 5.749228751562096562 ) ) ;
#6541=CARTESIAN_POINT ( 'NONE',  ( 0.000000000000000000, 0.000000000000000000, 21.50000000000000000 ) ) ;
#6546=ORIENTED_EDGE ( 'NONE', *, *, #17599, .F. ) ;
#6556=B_SPLINE_CURVE_WITH_KNOTS ( 'NONE', 3,
 ( #18209, #8398, #1527, #22567, #25067, #10884, #27573, #13688, #20843, #20395, #3864, #6199, #13386, #9006, #18374, #17911, #6506, #27425 ),
 .UNSPECIFIED., .F., .F.,
 ( 4, 2, 2, 2, 2, 2, 2, 2, 4 ),
 ( 0.003174295595554300041, 0.003570702171545529768, 0.003967108747536759496, 0.004363515323527989223, 0.004759921899519219818, 0.005156328475510448678, 0.005552735051501679273, 0.005949141627492909000, 0.006345548203484138727 ),
 .UNSPECIFIED. ) ;
#6558=CARTESIAN_POINT ( 'NONE',  ( 10.44969336715137409, -17.07413037334559647, 18.71435384576123440 ) ) ;
#6559=CARTESIAN_POINT ( 'NONE',  ( -16.96556290498877573, 1.647560670993253540, 18.34798005863078885 ) ) ;
#6561=EDGE_CURVE ( 'NONE', #16378, #17362, #19714, .T. ) ;
#6562=CARTESIAN_POINT ( 'NONE',  ( -16.81358047026920843, 2.650995224496061287, 19.45164628100866722 ) ) ;
#6563=CARTESIAN_POINT ( 'NONE',  ( 18.25868057198135830, -8.206406842115287148, 7.632642797338977658 ) ) ;
#6564=CARTESIAN_POINT ( 'NONE',  ( -13.95039892200172105, 9.845341970609696958, 7.098451512883313441 ) ) ;
#6565=CARTESIAN_POINT ( 'NONE',  ( 3.971879806607519825, 16.57852306707251344, 18.34838970509067479 ) ) ;
#6566=VERTEX_POINT ( 'NONE', #12873 ) ;
#6567=VERTEX_POINT ( 'NONE', #26598 ) ;
#6568=DIRECTION ( 'NONE',  ( 1.000000000000000000, 0.000000000000000000, 0.000000000000000000 ) ) ;
#6570=CARTESIAN_POINT ( 'NONE',  ( -10.82521593960875528, 5.400395169024524655, 24.50000000000000000 ) ) ;
#6571=CARTESIAN_POINT ( 'NONE',  ( -5.020628478053032140, 16.27454347535057622, 20.19668224736330941 ) ) ;
#6575=CARTESIAN_POINT ( 'NONE',  ( -5.971396161871753705, 19.08775596758252391, 7.652108011868850035 ) ) ;
#6577=ORIENTED_EDGE ( 'NONE', *, *, #23178, .T. ) ;
#6578=EDGE_CURVE ( 'NONE', #26575, #29559, #4626, .T. ) ;
#6579=AXIS2_PLACEMENT_3D ( 'NONE', #15050, #12732, #22230 ) ;
#6580=CARTESIAN_POINT ( 'NONE',  ( -19.96205336850438528, 1.490391487655214453, 6.672349528511551497 ) ) ;
#6581=CARTESIAN_POINT ( 'NONE',  ( 14.70507365826911972, 13.55638513645771503, 20.32200205377525393 ) ) ;
#6583=VERTEX_POINT ( 'NONE', #15030 ) ;
#6586=CARTESIAN_POINT ( 'NONE',  ( 18.59976559251667183, -7.400385892474091953, 5.872146474157316831 ) ) ;
#6595=DIRECTION ( 'NONE',  ( 1.000000000000000000, 0.000000000000000000, 0.000000000000000000 ) ) ;
#6597=VERTEX_POINT ( 'NONE', #9901 ) ;
#6602=CARTESIAN_POINT ( 'NONE',  ( -15.13023987665972392, -7.854877310202117435, 18.34838970509067479 ) ) ;
#6606=FACE_BOUND ( 'NONE', #6195, .T. ) ;
#6607=VECTOR ( 'NONE', #1319, 1000.000000000000000 ) ;
#6611=DIRECTION ( 'NONE',  ( -1.000000000000000000, 0.000000000000000000, 0.000000000000000000 ) ) ;
#6613=ORIENTED_EDGE ( 'NONE', *, *, #21231, .F. ) ;
#6614=CARTESIAN_POINT ( 'NONE',  ( -13.37849590498012908, 10.56201291617988147, 7.652108011868850923 ) ) ;
#6617=CARTESIAN_POINT ( 'NONE',  ( -9.471281197126605989, -0.4564504349074081091, 21.50000000000000000 ) ) ;
#6618=DIRECTION ( 'NONE',  ( -0.000000000000000000, -0.000000000000000000, 1.000000000000000000 ) ) ;
#6619=ADVANCED_FACE ( 'NONE', ( #7414 ), #16922, .F. ) ;
#6625=ORIENTED_EDGE ( 'NONE', *, *, #23630, .F. ) ;
#6628=LINE ( 'NONE', #16143, #8897 ) ;
#6632=CARTESIAN_POINT ( 'NONE',  ( 9.471281197126602436, 0.4564504349074715028, 13.00000000000000178 ) ) ;
#6634=CARTESIAN_POINT ( 'NONE',  ( 8.884323311075775109, 1.438332125858202692, 21.50000000000000000 ) ) ;
#6636=CARTESIAN_POINT ( 'NONE',  ( -18.40581374043504681, -7.824871006739526180, 18.84056766331481825 ) ) ;
#6637=CARTESIAN_POINT ( 'NONE',  ( -18.11003155545035881, -8.529482236167146070, 20.34789198813115263 ) ) ;
#6641=DIRECTION ( 'NONE',  ( -0.000000000000000000, -0.000000000000000000, 1.000000000000000000 ) ) ;
#6646=CARTESIAN_POINT ( 'NONE',  ( 17.94887244118349301, -8.863227448567842615, 19.00652017443069752 ) ) ;
#6647=CARTESIAN_POINT ( 'NONE',  ( 4.263339901971998636, 16.49757000336419210, 5.670038381137163519 ) ) ;
#6650=AXIS2_PLACEMENT_3D ( 'NONE', #8153, #17822, #30122 ) ;
#6651=CARTESIAN_POINT ( 'NONE',  ( -19.85654738780300121, 2.535877853918448555, 5.651989602109218858 ) ) ;
#6653=DIRECTION ( 'NONE',  ( 0.000000000000000000, 0.000000000000000000, 1.000000000000000000 ) ) ;
#6655=LINE ( 'NONE', #28952, #16332 ) ;
#6657=CARTESIAN_POINT ( 'NONE',  ( -15.01328179936714413, 13.21424408877643941, 7.526993102356318133 ) ) ;
#6663=CARTESIAN_POINT ( 'NONE',  ( 0.4421796641654209825, -17.03052986487778497, 7.595116371587256054 ) ) ;
#6667=CARTESIAN_POINT ( 'NONE',  ( -17.06629068372215130, 0.6401188461407910646, 19.36813350477385143 ) ) ;
#6669=VERTEX_POINT ( 'NONE', #26748 ) ;
#6671=CARTESIAN_POINT ( 'NONE',  ( 10.67336573878037420, -13.33112751634288706, 19.58863275299554019 ) ) ;
#6675=EDGE_CURVE ( 'NONE', #12022, #17226, #383, .T. ) ;
#6676=CARTESIAN_POINT ( 'NONE',  ( -15.84912786217079450, 12.19893545703369142, 7.272192800924334399 ) ) ;
#6684=CARTESIAN_POINT ( 'NONE',  ( -15.51517975927889204, 12.62116967784147725, 18.37545668562167478 ) ) ;
#6685=DIRECTION ( 'NONE',  ( 0.000000000000000000, 0.000000000000000000, -1.000000000000000000 ) ) ;
#6689=ORIENTED_EDGE ( 'NONE', *, *, #24489, .T. ) ;
#6690=EDGE_CURVE ( 'NONE', #10914, #2256, #9123, .T. ) ;
#6692=VERTEX_POINT ( 'NONE', #25016 ) ;
#6698=CARTESIAN_POINT ( 'NONE',  ( 1.665992581735233014, -16.99218467486976891, 18.84329447212443753 ) ) ;
#6699=DIRECTION ( 'NONE',  ( -0.5406408174555976665, 0.8412535328311812055, 0.000000000000000000 ) ) ;
#6700=EDGE_LOOP ( 'NONE', ( #10809, #11098, #11939, #30233 ) ) ;
#6701=CARTESIAN_POINT ( 'NONE',  ( -19.85166970746586301, 2.573860339590182456, 18.34969686940296185 ) ) ;
#6702=CARTESIAN_POINT ( 'NONE',  ( 3.912171961291947664, 8.637616862297855747, 1.500000000000001332 ) ) ;
#6703=CARTESIAN_POINT ( 'NONE',  ( -13.42620032052776047, 10.50496109755573926, 20.34789198813115263 ) ) ;
#6704=CARTESIAN_POINT ( 'NONE',  ( 4.454645749177147174, 19.51581340210660187, 18.82680253904184298 ) ) ;
#6719=VERTEX_POINT ( 'NONE', #20026 ) ;
#6721=CARTESIAN_POINT ( 'NONE',  ( -19.93785161568571951, 1.787211178945724788, 7.366751648393900176 ) ) ;
#6729=CARTESIAN_POINT ( 'NONE',  ( 18.41347767057966678, -7.852385608265392669, 5.661398277488801867 ) ) ;
#6731=ORIENTED_EDGE ( 'NONE', *, *, #27513, .F. ) ;
#6736=LINE ( 'NONE', #20622, #15792 ) ;
#6737=CARTESIAN_POINT ( 'NONE',  ( -6.044935790874366610, 19.08338196164711675, 20.34789198813115263 ) ) ;
#6741=ORIENTED_EDGE ( 'NONE', *, *, #22526, .T. ) ;
#6744=LINE ( 'NONE', #18466, #25299 ) ;
#6748=CYLINDRICAL_SURFACE ( 'NONE', #1614, 9.482273699623480212 ) ;
#6749=FACE_OUTER_BOUND ( 'NONE', #16940, .T. ) ;
#6753=CARTESIAN_POINT ( 'NONE',  ( 0.09286997694516960222, -20.00015982525768266, 18.37250658438899364 ) ) ;
#6762=ORIENTED_EDGE ( 'NONE', *, *, #14771, .F. ) ;
#6765=ORIENTED_EDGE ( 'NONE', *, *, #11376, .F. ) ;
#6768=DIRECTION ( 'NONE',  ( 1.000000000000000000, 0.000000000000000000, 0.000000000000000000 ) ) ;
#6769=ORIENTED_EDGE ( 'NONE', *, *, #24779, .T. ) ;
#6770=CARTESIAN_POINT ( 'NONE',  ( 18.71829317531095072, -7.044536951825313587, 6.788986777570698017 ) ) ;
#6771=AXIS2_PLACEMENT_3D ( 'NONE', #7171, #12010, #25735 ) ;
#6775=ORIENTED_EDGE ( 'NONE', *, *, #8004, .T. ) ;
#6777=CARTESIAN_POINT ( 'NONE',  ( 0.000000000000000000, 0.000000000000000000, 21.50000000000000000 ) ) ;
#6778=VECTOR ( 'NONE', #3170, 1000.000000000000227 ) ;
#6781=CARTESIAN_POINT ( 'NONE',  ( -13.11527592942575282, -10.04126165406389326, 24.50000000000000000 ) ) ;
#6784=CARTESIAN_POINT ( 'NONE',  ( -18.32589276785171606, -8.054604467211156305, 20.12545155307891065 ) ) ;
#6794=CARTESIAN_POINT ( 'NONE',  ( -6.045292009585545578, 15.95527889502104024, 20.24143955528809258 ) ) ;
#6795=CARTESIAN_POINT ( 'NONE',  ( 4.476939094886643211, 16.43504713094788272, 7.557577766377196582 ) ) ;
#6796=AXIS2_PLACEMENT_3D ( 'NONE', #21849, #29342, #17014 ) ;
#6798=CARTESIAN_POINT ( 'NONE',  ( -19.71314312682348557, 3.479754436677863438, 6.420335371522007506 ) ) ;
#6800=CARTESIAN_POINT ( 'NONE',  ( 14.24237608451263348, 14.06627278277045079, 6.995624166085161910 ) ) ;
#6804=ORIENTED_EDGE ( 'NONE', *, *, #2144, .T. ) ;
#6809=CARTESIAN_POINT ( 'NONE',  ( 16.87360174012497538, 2.245128340606972639, 19.66962785902261857 ) ) ;
#6811=CARTESIAN_POINT ( 'NONE',  ( -9.056208293496290196, 2.810445847081948667, 21.50000000000000000 ) ) ;
#6813=VECTOR ( 'NONE', #23335, 1000.000000000000000 ) ;
#6817=CARTESIAN_POINT ( 'NONE',  ( -19.93785161568571951, 1.787211178945723677, 20.06253562465620632 ) ) ;
#6818=CARTESIAN_POINT ( 'NONE',  ( -13.00999358272542494, -0.8602714556717691030, 1.500000000000001332 ) ) ;
#6821=CARTESIAN_POINT ( 'NONE',  ( 11.94417982595701666, -16.06366807669217067, 19.47783254395485031 ) ) ;
#6823=DIRECTION ( 'NONE',  ( 0.000000000000000000, 0.000000000000000000, -1.000000000000000000 ) ) ;
#6826=CARTESIAN_POINT ( 'NONE',  ( 5.296161872597624942, 19.28602264385379428, 20.34789198813115263 ) ) ;
#6827=ORIENTED_EDGE ( 'NONE', *, *, #30346, .T. ) ;
#6828=B_SPLINE_CURVE_WITH_KNOTS ( 'NONE', 3,
 ( #23719, #11892, #9539, #19054, #26223, #12816, #14988, #19519, #26542, #17494, #12515, #5643, #22319, #5170, #8139, #12668, #24816, #12355 ),
 .UNSPECIFIED., .F., .F.,
 ( 4, 2, 2, 2, 2, 2, 2, 2, 4 ),
 ( 0.003174295595554328664, 0.003570702171545568800, 0.003967108747536808935, 0.004363515323528048204, 0.004759921899519288339, 0.005156328475510528475, 0.005552735051501767743, 0.005949141627493007879, 0.006345548203484248015 ),
 .UNSPECIFIED. ) ;
#6832=CIRCLE ( 'NONE', #27783, 0.7500000000000006661 ) ;
#6839=ORIENTED_EDGE ( 'NONE', *, *, #24420, .T. ) ;
#6844=CIRCLE ( 'NONE', #12863, 9.482273699623480212 ) ;
#6847=CARTESIAN_POINT ( 'NONE',  ( -0.1984805017707983177, -17.02075843868200522, 19.60617949693493856 ) ) ;
#6852=CARTESIAN_POINT ( 'NONE',  ( 19.86222817340373226, 2.491431357970652183, 18.63641924841378028 ) ) ;
#6855=CARTESIAN_POINT ( 'NONE',  ( -19.75958569938476472, 3.205325445645400784, 18.63641924841378028 ) ) ;
#6858=CARTESIAN_POINT ( 'NONE',  ( -15.80654879600846741, 12.28271411401622970, 7.366751648393900176 ) ) ;
#6859=CYLINDRICAL_SURFACE ( 'NONE', #3863, 9.482273699623480212 ) ;
#6864=LINE ( 'NONE', #28700, #14621 ) ;
#6866=DIRECTION ( 'NONE',  ( 1.000000000000000000, 0.000000000000000000, 0.000000000000000000 ) ) ;
#6867=DIRECTION ( 'NONE',  ( 1.000000000000000000, 0.000000000000000000, 0.000000000000000000 ) ) ;
#6872=ORIENTED_EDGE ( 'NONE', *, *, #20439, .F. ) ;
#6873=AXIS2_PLACEMENT_3D ( 'NONE', #18609, #27826, #11582 ) ;
#6874=ADVANCED_BREP_SHAPE_REPRESENTATION ( '', ( #2508, #7396 ), #26315 ) ;
#6875=CARTESIAN_POINT ( 'NONE',  ( -17.05861610865858324, 0.7402736376837879551, 7.098451512883313441 ) ) ;
#6876=CARTESIAN_POINT ( 'NONE',  ( 14.79453494486351772, 13.45878767717418789, 20.34789198813115618 ) ) ;
#6877=CARTESIAN_POINT ( 'NONE',  ( 19.81789086666766764, 2.695592600026628372, 18.47110296274024321 ) ) ;
#6886=ADVANCED_FACE ( 'NONE', ( #16565 ), #14217, .F. ) ;
#6890=CARTESIAN_POINT ( 'NONE',  ( -18.45589647530846023, -7.705834498630351526, 6.781503518395066266 ) ) ;
#6891=CARTESIAN_POINT ( 'NONE',  ( -6.185259412586026961, 19.03819474808297230, 20.32367522806703874 ) ) ;
#6894=EDGE_CURVE ( 'NONE', #21299, #6719, #9248, .T. ) ;
#6902=AXIS2_PLACEMENT_3D ( 'NONE', #3942, #16228, #11107 ) ;
#6903=CYLINDRICAL_SURFACE ( 'NONE', #2829, 1.000000000000009548 ) ;
#6910=CARTESIAN_POINT ( 'NONE',  ( -14.58213539500865785, 7.758783772730382111, 24.50000000000000000 ) ) ;
#6914=CARTESIAN_POINT ( 'NONE',  ( -4.608906612435655248, -7.730328572437724866, 1.500000000000001332 ) ) ;
#6920=CARTESIAN_POINT ( 'NONE',  ( -14.01107592578417993, 9.765138712360668549, 6.783738457429056012 ) ) ;
#6928=ORIENTED_EDGE ( 'NONE', *, *, #29680, .F. ) ;
#6929=CARTESIAN_POINT ( 'NONE',  ( -0.2808233399669979313, -20.01605574108312169, 18.55820869691756769 ) ) ;
#6931=ADVANCED_FACE ( 'NONE', ( #27486 ), #22632, .F. ) ;
#6932=CARTESIAN_POINT ( 'NONE',  ( -7.685008110482990595, -15.25093183970990296, 6.447548852708279377 ) ) ;
#6934=VECTOR ( 'NONE', #5925, 1000.000000000000000 ) ;
#6935=CARTESIAN_POINT ( 'NONE',  ( 1.792916928892102080, -16.98383425522534651, 19.47783254395485031 ) ) ;
#6937=EDGE_CURVE ( 'NONE', #22820, #27449, #11119, .T. ) ;
#6938=CARTESIAN_POINT ( 'NONE',  ( 18.70942253818554235, -7.068249826530434099, 6.392525840300342210 ) ) ;
#6939=CARTESIAN_POINT ( 'NONE',  ( 16.74328841314637017, 3.194145055459935545, 7.652108011868850923 ) ) ;
#6940=DIRECTION ( 'NONE',  ( -0.000000000000000000, -0.000000000000000000, 1.000000000000000000 ) ) ;
#6946=CARTESIAN_POINT ( 'NONE',  ( -12.74661400762298413, 11.28197093999160394, 19.66962785902261857 ) ) ;
#6948=CARTESIAN_POINT ( 'NONE',  ( -9.169883732660077058, -9.268939115642981008, 1.500000000000001332 ) ) ;
#6950=CARTESIAN_POINT ( 'NONE',  ( -15.30782679199506191, -7.476958555467157375, 20.29090034784956131 ) ) ;
#6953=ORIENTED_EDGE ( 'NONE', *, *, #11284, .T. ) ;
#6954=LINE ( 'NONE', #28476, #11466 ) ;
#6958=VERTEX_POINT ( 'NONE', #24979 ) ;
#6960=AXIS2_PLACEMENT_3D ( 'NONE', #23440, #13793, #4576 ) ;
#6961=CARTESIAN_POINT ( 'NONE',  ( 4.996079307276527715, 16.27198743970617301, 6.420335371522007506 ) ) ;
#6963=ORIENTED_EDGE ( 'NONE', *, *, #27505, .F. ) ;
#6964=DIRECTION ( 'NONE',  ( 1.000000000000000000, 0.000000000000000000, 0.000000000000000000 ) ) ;
#6965=CARTESIAN_POINT ( 'NONE',  ( 11.92830948316210993, 12.20365889974009477, 7.441806358946449151 ) ) ;
#6967=VECTOR ( 'NONE', #23775, 1000.000000000000000 ) ;
#6973=CARTESIAN_POINT ( 'NONE',  ( -14.69500743155267841, 13.56684717634543702, 6.386539667786089502 ) ) ;
#6975=CARTESIAN_POINT ( 'NONE',  ( -15.57452153527462535, -6.867569271111572782, 6.530762810602277924 ) ) ;
#6979=CARTESIAN_POINT ( 'NONE',  ( 0.1201197967225750701, -20.01774464624827132, 7.632642797338977658 ) ) ;
#6983=CARTESIAN_POINT ( 'NONE',  ( 1.687027447297431371, 8.840471615930075799, 1.500000000000001332 ) ) ;
#6986=CARTESIAN_POINT ( 'NONE',  ( -6.501324370950584353, 15.79217903278762947, 6.521906765011497242 ) ) ;
#6989=EDGE_LOOP ( 'NONE', ( #30751, #6872, #30474, #19852 ) ) ;
#6990=CARTESIAN_POINT ( 'NONE',  ( 4.800123045415256584, 19.41580659536132458, 18.47531940416305929 ) ) ;
#6991=ORIENTED_EDGE ( 'NONE', *, *, #6301, .T. ) ;
#6992=CARTESIAN_POINT ( 'NONE',  ( 15.19061449783604623, 13.03728791304909507, 20.25336174263950184 ) ) ;
#6995=CARTESIAN_POINT ( 'NONE',  ( 18.48560952955219960, -7.681425967031921154, 18.39992786714538298 ) ) ;
#6996=CARTESIAN_POINT ( 'NONE',  ( 16.59873159789848529, 3.986191100139168775, 18.73743063545763121 ) ) ;
#7002=ADVANCED_FACE ( 'NONE', ( #25294 ), #22943, .T. ) ;
#7003=ORIENTED_EDGE ( 'NONE', *, *, #10346, .T. ) ;
#7005=ORIENTED_EDGE ( 'NONE', *, *, #21517, .F. ) ;
#7008=CARTESIAN_POINT ( 'NONE',  ( 1.568770080425524904, -16.99791492429842066, 7.280727868105637768 ) ) ;
#7009=DIRECTION ( 'NONE',  ( -0.000000000000000000, -0.000000000000000000, -1.000000000000000000 ) ) ;
#7010=CARTESIAN_POINT ( 'NONE',  ( 1.305293688432930699, -17.01213356654596964, 20.24143955528809613 ) ) ;
#7012=EDGE_LOOP ( 'NONE', ( #23521, #6526, #22022, #1173 ) ) ;
#7013=AXIS2_PLACEMENT_3D ( 'NONE', #18144, #10976, #29852 ) ;
#7014=CARTESIAN_POINT ( 'NONE',  ( -16.82311188420106163, 2.597149461308117413, 19.00652017443069752 ) ) ;
#7016=VECTOR ( 'NONE', #11366, 1000.000000000000000 ) ;
#7017=DIRECTION ( 'NONE',  ( 1.000000000000000000, 0.000000000000000000, 0.000000000000000000 ) ) ;
#7023=CARTESIAN_POINT ( 'NONE',  ( -5.905415913170754649, 19.12693415355693105, 18.34969686940295830 ) ) ;
#7024=B_SPLINE_CURVE_WITH_KNOTS ( 'NONE', 3,
 ( #13310, #15953, #11120, #20614, #5976, #29848, #15475, #4093, #27960, #1136, #15318, #8318, #24993, #8767, #25144, #13625, #1610, #15631 ),
 .UNSPECIFIED., .F., .F.,
 ( 4, 2, 2, 2, 2, 2, 2, 2, 4 ),
 ( 0.000000000000000000, 0.0003967869494442882099, 0.0007935738988885764197, 0.001190360848332864575, 0.001587147797777152839, 0.001983934747221441103, 0.002380721696665729151, 0.002777508646110017632, 0.003174295595554305679 ),
 .UNSPECIFIED. ) ;
#7028=CARTESIAN_POINT ( 'NONE',  ( -19.95437879344081367, 1.590546279198207680, 7.098451512883313441 ) ) ;
#7029=CARTESIAN_POINT ( 'NONE',  ( 14.45728346696244593, 13.82012126338015712, 18.54958172136248606 ) ) ;
#7034=CARTESIAN_POINT ( 'NONE',  ( 13.00999358272542850, -0.8602714556717643291, 1.500000000000001332 ) ) ;
#7036=AXIS2_PLACEMENT_3D ( 'NONE', #20472, #6440, #8626 ) ;
#7043=CARTESIAN_POINT ( 'NONE',  ( -6.493275194760120606, 15.79517802630851797, 19.14333282897057842 ) ) ;
#7046=EDGE_LOOP ( 'NONE', ( #8082, #1320, #16805, #8146 ) ) ;
#7060=CARTESIAN_POINT ( 'NONE',  ( -15.26435939152463384, 8.070345032481604619, -0.6213203435596476032 ) ) ;
#7062=EDGE_CURVE ( 'NONE', #26243, #466, #658, .T. ) ;
#7067=ORIENTED_EDGE ( 'NONE', *, *, #9731, .T. ) ;
#7068=ADVANCED_FACE ( 'NONE', ( #1445 ), #6261, .F. ) ;
#7070=CARTESIAN_POINT ( 'NONE',  ( 12.35846533491531041, 11.73919094685904696, 7.652108011868850923 ) ) ;
#7072=ADVANCED_FACE ( 'NONE', ( #10958 ), #15302, .F. ) ;
#7074=CARTESIAN_POINT ( 'NONE',  ( 2.959227181723801170, -8.499586724479446076, 1.500000000000001332 ) ) ;
#7079=CARTESIAN_POINT ( 'NONE',  ( -0.1401636875787321268, -17.02258069761206372, 19.77662771831109367 ) ) ;
#7081=CARTESIAN_POINT ( 'NONE',  ( -9.908187358984022808, -17.39367339311967342, 7.366751648393900176 ) ) ;
#7083=DIRECTION ( 'NONE',  ( 1.000000000000000000, 0.000000000000000000, 0.000000000000000000 ) ) ;
#7084=EDGE_CURVE ( 'NONE', #9428, #27809, #28090, .T. ) ;
#7085=CARTESIAN_POINT ( 'NONE',  ( 1.153863525602932150, -19.98436899483067819, 18.73743063545763121 ) ) ;
#7086=EDGE_LOOP ( 'NONE', ( #5244, #3291, #30213, #8621 ) ) ;
#7090=CARTESIAN_POINT ( 'NONE',  ( 11.67039530559478777, 12.46804495696167336, 19.14333282897057842 ) ) ;
#7092=ORIENTED_EDGE ( 'NONE', *, *, #28945, .T. ) ;
#7094=CARTESIAN_POINT ( 'NONE',  ( -15.01497154418444602, -8.089954645606729500, 5.704143890883081269 ) ) ;
#7097=CARTESIAN_POINT ( 'NONE',  ( -19.90131041440201187, 1.988107338454515149, 5.779535427900759359 ) ) ;
#7098=CARTESIAN_POINT ( 'NONE',  ( -18.09892777451933910, -8.511549950051179536, 18.34726407865099418 ) ) ;
#7100=DIRECTION ( 'NONE',  ( 0.7557495743542582689, -0.6548607339452851006, 0.000000000000000000 ) ) ;
#7102=ORIENTED_EDGE ( 'NONE', *, *, #18495, .F. ) ;
#7110=ORIENTED_EDGE ( 'NONE', *, *, #26877, .T. ) ;
#7112=CARTESIAN_POINT ( 'NONE',  ( 15.40995608898784397, -7.231564984717127054, 19.00652017443069752 ) ) ;
#7114=CARTESIAN_POINT ( 'NONE',  ( 5.409330662328856398, 19.27307614344555375, 5.657991946698900598 ) ) ;
#7115=ORIENTED_EDGE ( 'NONE', *, *, #19265, .F. ) ;
#7116=CARTESIAN_POINT ( 'NONE',  ( 5.730668117466260369, 19.18033075515274888, 20.25336174263950184 ) ) ;
#7118=LINE ( 'NONE', #245, #7269 ) ;
#7121=ORIENTED_EDGE ( 'NONE', *, *, #9417, .F. ) ;
#7122=LINE ( 'NONE', #28643, #22313 ) ;
#7125=AXIS2_PLACEMENT_3D ( 'NONE', #20307, #1283, #5964 ) ;
#7130=CARTESIAN_POINT ( 'NONE',  ( -15.57976790534003086, -6.855017190910956515, 6.641371103590088865 ) ) ;
#7133=CARTESIAN_POINT ( 'NONE',  ( 0.3158150563615996775, -20.01532941283344513, 5.651989602109218858 ) ) ;
#7136=LINE ( 'NONE', #23642, #26997 ) ;
#7137=CARTESIAN_POINT ( 'NONE',  ( -17.04815991962219357, 0.8662532504481892381, 19.97651184436794125 ) ) ;
#7138=DIRECTION ( 'NONE',  ( 0.000000000000000000, 0.000000000000000000, 1.000000000000000000 ) ) ;
#7142=CARTESIAN_POINT ( 'NONE',  ( 11.23845335764779563, -16.56542118924666340, 20.33971507717571114 ) ) ;
#7144=ORIENTED_EDGE ( 'NONE', *, *, #23562, .F. ) ;
#7147=CARTESIAN_POINT ( 'NONE',  ( 4.434078574240014170, 19.50234843602376955, 18.84486140012300126 ) ) ;
#7151=CARTESIAN_POINT ( 'NONE',  ( -10.52692833102915770, -17.02631732661572883, 7.652108011868850035 ) ) ;
#7153=CARTESIAN_POINT ( 'NONE',  ( 18.70304204834580020, -7.134633872344113392, 18.92976555901915603 ) ) ;
#7154=CARTESIAN_POINT ( 'NONE',  ( 19.59419491516168321, 4.095680178559272022, 19.79423548914561692 ) ) ;
#7157=CARTESIAN_POINT ( 'NONE',  ( 15.47543066139447987, -7.098048983848884497, 19.96344307082653202 ) ) ;
#7158=ORIENTED_EDGE ( 'NONE', *, *, #770, .F. ) ;
#7160=ORIENTED_EDGE ( 'NONE', *, *, #7282, .F. ) ;
#7161=VECTOR ( 'NONE', #21944, 1000.000000000000227 ) ;
#7165=CARTESIAN_POINT ( 'NONE',  ( 0.9820204223201481897, -19.99380624802878970, 7.441806358946449151 ) ) ;
#7166=CARTESIAN_POINT ( 'NONE',  ( -14.80112376877043445, -8.505769479261473975, 19.96568007040468373 ) ) ;
#7168=CARTESIAN_POINT ( 'NONE',  ( 16.74864137134695596, 3.161078882829539971, 18.34777357837152323 ) ) ;
#7169=ORIENTED_EDGE ( 'NONE', *, *, #19874, .F. ) ;
#7171=CARTESIAN_POINT ( 'NONE',  ( -14.58213539500865785, 7.758783772730382111, 24.50000000000000000 ) ) ;
#7177=FACE_OUTER_BOUND ( 'NONE', #18355, .T. ) ;
#7182=AXIS2_PLACEMENT_3D ( 'NONE', #10131, #24478, #3122 ) ;
#7183=CARTESIAN_POINT ( 'NONE',  ( -5.719992972340618209, 19.16498258860014658, 7.626647697317578967 ) ) ;
#7184=ORIENTED_EDGE ( 'NONE', *, *, #11481, .F. ) ;
#7186=CARTESIAN_POINT ( 'NONE',  ( -17.59389297287863840, -9.510918850537244396, 19.08830981656263859 ) ) ;
#7191=CARTESIAN_POINT ( 'NONE',  ( 16.11353791281288395, -5.634185590772410990, 7.280727868105637768 ) ) ;
#7192=DIRECTION ( 'NONE',  ( 1.000000000000000000, 0.000000000000000000, 0.000000000000000000 ) ) ;
#7196=DIRECTION ( 'NONE',  ( -0.000000000000000000, -0.000000000000000000, 1.000000000000000000 ) ) ;
#7197=CARTESIAN_POINT ( 'NONE',  ( -18.04156136322729864, -8.631457789788587576, 5.652196082369963293 ) ) ;
#7202=CARTESIAN_POINT ( 'NONE',  ( 15.76152542347981900, -6.481515897568145057, 5.651492010659114662 ) ) ;
#7207=CARTESIAN_POINT ( 'NONE',  ( -17.61017686385352121, -9.517781650307574282, 19.58863275299554019 ) ) ;
#7208=DIRECTION ( 'NONE',  ( 0.9898214418809327952, -0.1423148382732850048, 0.000000000000000000 ) ) ;
#7214=CARTESIAN_POINT ( 'NONE',  ( -11.40980092660686829, 6.310027164379044429, 1.500000000000001332 ) ) ;
#7215=ORIENTED_EDGE ( 'NONE', *, *, #6108, .F. ) ;
#7217=ORIENTED_EDGE ( 'NONE', *, *, #130, .T. ) ;
#7218=CARTESIAN_POINT ( 'NONE',  ( -15.34307810681595186, 12.82926163924265950, 20.34789198813115263 ) ) ;
#7219=CARTESIAN_POINT ( 'NONE',  ( 0.000000000000000000, 0.000000000000000000, 1.500000000000001332 ) ) ;
#7221=AXIS2_PLACEMENT_3D ( 'NONE', #28946, #12883, #10378 ) ;
#7226=CARTESIAN_POINT ( 'NONE',  ( -0.6606983433884117130, -20.00701505202155062, 19.45164628100866722 ) ) ;
#7227=CARTESIAN_POINT ( 'NONE',  ( -8.006961111548653420, -15.06991809617584899, 7.441806358946449151 ) ) ;
#7231=EDGE_CURVE ( 'NONE', #15032, #5400, #23690, .T. ) ;
#7232=DIRECTION ( 'NONE',  ( 1.000000000000000000, 0.000000000000000000, 0.000000000000000000 ) ) ;
#7234=CARTESIAN_POINT ( 'NONE',  ( 11.65818676052302294, 12.48028922388247253, 19.25672174529527325 ) ) ;
#7236=ORIENTED_EDGE ( 'NONE', *, *, #15125, .F. ) ;
#7238=CIRCLE ( 'NONE', #1816, 0.7500000000000007772 ) ;
#7240=CARTESIAN_POINT ( 'NONE',  ( -15.09693789817080578, -7.923486267757679613, 5.661398277488802755 ) ) ;
#7241=CARTESIAN_POINT ( 'NONE',  ( 12.24063095261064404, 4.490763173670002217, 24.50000000000000000 ) ) ;
#7242=CIRCLE ( 'NONE', #256, 20.00000000000000000 ) ;
#7244=CARTESIAN_POINT ( 'NONE',  ( 19.78395057425408154, 2.934310293824245353, 7.626647697317575414 ) ) ;
#7251=CARTESIAN_POINT ( 'NONE',  ( -8.321991900972895095, -14.88664253267596571, 5.653604225791663218 ) ) ;
#7253=FACE_OUTER_BOUND ( 'NONE', #5138, .T. ) ;
#7254=EDGE_LOOP ( 'NONE', ( #24570, #28698, #5501, #22453 ) ) ;
#7256=CARTESIAN_POINT ( 'NONE',  ( 18.05043922081454610, -8.654756627348808351, 20.05479082170252525 ) ) ;
#7259=CARTESIAN_POINT ( 'NONE',  ( 5.818449564404023278, 19.15386117387415510, 5.796888747622817029 ) ) ;
#7260=EDGE_CURVE ( 'NONE', #9004, #29934, #11139, .T. ) ;
#7263=CARTESIAN_POINT ( 'NONE',  ( 11.86828576611216235, 12.26598719735377863, 7.366751648393900176 ) ) ;
#7264=B_SPLINE_CURVE_WITH_KNOTS ( 'NONE', 3,
 ( #5652, #5802, #5334, #10021, #1121, #14686, #10634, #21867, #17031, #3154, #12983, #20146, #19529, #15147, #24508, #14843, #17656, #5495 ),
 .UNSPECIFIED., .F., .F.,
 ( 4, 2, 2, 2, 2, 2, 2, 2, 4 ),
 ( 0.003174295595554332567, 0.003570702171545570534, 0.003967108747536808935, 0.004363515323528046469, 0.004759921899519284870, 0.005156328475510523271, 0.005552735051501760805, 0.005949141627492998338, 0.006345548203484236739 ),
 .UNSPECIFIED. ) ;
#7267=ORIENTED_EDGE ( 'NONE', *, *, #26959, .F. ) ;
#7269=VECTOR ( 'NONE', #14444, 1000.000000000000000 ) ;
#7270=CARTESIAN_POINT ( 'NONE',  ( 6.630478080506912342, 6.778663211761485563, 13.00000000000000178 ) ) ;
#7272=FACE_OUTER_BOUND ( 'NONE', #15628, .T. ) ;
#7274=CARTESIAN_POINT ( 'NONE',  ( -15.42813811594282036, -7.209250886987519813, 5.862424720655265098 ) ) ;
#7275=CARTESIAN_POINT ( 'NONE',  ( -12.86767874445213877, -1.850092897552710225, 24.50000000000000000 ) ) ;
#7276=AXIS2_PLACEMENT_3D ( 'NONE', #12882, #24708, #20497 ) ;
#7282=EDGE_CURVE ( 'NONE', #9215, #23733, #21584, .T. ) ;
#7284=CARTESIAN_POINT ( 'NONE',  ( 1.000000000000008438, 19.97498435543819184, 1.500000000000001332 ) ) ;
#7285=CARTESIAN_POINT ( 'NONE',  ( -19.96188467872886463, 1.492656647078444809, 19.47783254395485031 ) ) ;
#7287=EDGE_CURVE ( 'NONE', #6669, #203, #18102, .T. ) ;
#7288=CARTESIAN_POINT ( 'NONE',  ( 11.92709382895865566, -16.07640909887372516, 19.58863275299554019 ) ) ;
#7289=DIRECTION ( 'NONE',  ( 0.000000000000000000, 0.000000000000000000, -1.000000000000000000 ) ) ;
#7290=ORIENTED_EDGE ( 'NONE', *, *, #6157, .F. ) ;
#7292=EDGE_CURVE ( 'NONE', #17125, #1255, #15622, .T. ) ;
#7297=B_SPLINE_CURVE_WITH_KNOTS ( 'NONE', 3,
 ( #6575, #1599, #7183, #26053, #16852, #24158, #2191, #2340, #16387, #14507, #26368, #26203, #26517, #21195, #153, #9674, #9369, #19183 ),
 .UNSPECIFIED., .F., .F.,
 ( 4, 2, 2, 2, 2, 2, 2, 2, 4 ),
 ( 0.003174295595554313485, 0.003570702171545544080, 0.003967108747536775108, 0.004363515323528005703, 0.004759921899519236298, 0.005156328475510467760, 0.005552735051501698355, 0.005949141627492928949, 0.006345548203484159544 ),
 .UNSPECIFIED. ) ;
#7300=VERTEX_POINT ( 'NONE', #305 ) ;
#7304=VERTEX_POINT ( 'NONE', #12018 ) ;
#7305=CARTESIAN_POINT ( 'NONE',  ( 18.44211820063743446, -7.784504718833766823, 18.37415474056476938 ) ) ;
#7308=FACE_OUTER_BOUND ( 'NONE', #1251, .T. ) ;
#7311=DIRECTION ( 'NONE',  ( 1.000000000000000000, 0.000000000000000000, 0.000000000000000000 ) ) ;
#7313=VERTEX_POINT ( 'NONE', #9828 ) ;
#7314=EDGE_CURVE ( 'NONE', #30491, #1882, #27179, .T. ) ;
#7319=ADVANCED_FACE ( 'NONE', ( #19635 ), #14654, .F. ) ;
#7322=CARTESIAN_POINT ( 'NONE',  ( -12.85282321250444681, 11.16584596974482935, 19.96783386855779341 ) ) ;
#7323=CIRCLE ( 'NONE', #840, 0.7500000000000006661 ) ;
#7324=EDGE_CURVE ( 'NONE', #20845, #11886, #21081, .T. ) ;
#7325=CARTESIAN_POINT ( 'NONE',  ( 6.630478080506909677, 6.778663211761489116, 1.500000000000001332 ) ) ;
#7326=CARTESIAN_POINT ( 'NONE',  ( 0.000000000000000000, 0.000000000000000000, 1.500000000000001332 ) ) ;
#7330=CARTESIAN_POINT ( 'NONE',  ( -16.85109579167143323, 2.433552959544810435, 18.71435384576123440 ) ) ;
#7331=CARTESIAN_POINT ( 'NONE',  ( -11.40980092660686829, 6.310027164379044429, 24.50000000000000000 ) ) ;
#7333=FACE_OUTER_BOUND ( 'NONE', #19003, .T. ) ;
#7339=CARTESIAN_POINT ( 'NONE',  ( 18.53505294460180508, -7.514422089582846631, 18.47531940416306995 ) ) ;
#7340=DIRECTION ( 'NONE',  ( 0.000000000000000000, 0.000000000000000000, 1.000000000000000000 ) ) ;
#7341=CIRCLE ( 'NONE', #2860, 0.7500000000000006661 ) ;
#7348=CARTESIAN_POINT ( 'NONE',  ( -17.64259547893122360, -9.420269215336071866, 18.84486140012300126 ) ) ;
#7350=ORIENTED_EDGE ( 'NONE', *, *, #30029, .F. ) ;
#7351=CARTESIAN_POINT ( 'NONE',  ( 15.41319392345653938, 12.77323265862689183, 6.018569869498933578 ) ) ;
#7353=VECTOR ( 'NONE', #25663, 1000.000000000000000 ) ;
#7356=AXIS2_PLACEMENT_3D ( 'NONE', #16372, #9351, #14026 ) ;
#7358=CARTESIAN_POINT ( 'NONE',  ( 16.65321191614105345, 3.713086717969341866, 20.24143955528808902 ) ) ;
#7359=DIRECTION ( 'NONE',  ( 1.000000000000000000, 0.000000000000000000, 0.000000000000000000 ) ) ;
#7360=ORIENTED_EDGE ( 'NONE', *, *, #13042, .T. ) ;
#7361=AXIS2_PLACEMENT_3D ( 'NONE', #10774, #23064, #6243 ) ;
#7362=CARTESIAN_POINT ( 'NONE',  ( 3.898220458062934046, 16.59828442330441689, 5.661398277488802755 ) ) ;
#7363=CARTESIAN_POINT ( 'NONE',  ( -8.072557715923444732, 14.41080185948837311, 24.50000000000000000 ) ) ;
#7372=CARTESIAN_POINT ( 'NONE',  ( 9.999999999999959144, 1.510243460696181139E-14, 24.50000000000000000 ) ) ;
#7373=CARTESIAN_POINT ( 'NONE',  ( -14.70315170625142365, -8.688231105434649493, 19.36813350477385143 ) ) ;
#7379=VECTOR ( 'NONE', #13092, 1000.000000000000114 ) ;
#7380=EDGE_LOOP ( 'NONE', ( #24925, #16760 ) ) ;
#7381=CARTESIAN_POINT ( 'NONE',  ( -1.000000000000008438, 13.00000000000001421, 1.500000000000001332 ) ) ;
#7383=CARTESIAN_POINT ( 'NONE',  ( -6.742350454026557749, 18.82948505227174962, 6.037995405461185072 ) ) ;
#7389=CIRCLE ( 'NONE', #18832, 0.7500000000000006661 ) ;
#7390=ORIENTED_EDGE ( 'NONE', *, *, #19318, .T. ) ;
#7393=ORIENTED_EDGE ( 'NONE', *, *, #26959, .T. ) ;
#7394=ORIENTED_EDGE ( 'NONE', *, *, #23095, .F. ) ;
#7395=CARTESIAN_POINT ( 'NONE',  ( -0.6129396130214324057, -20.00853051056088461, 19.66989035740801839 ) ) ;
#7396=AXIS2_PLACEMENT_3D ( 'NONE', #9486, #28514, #21014 ) ;
#7397=CARTESIAN_POINT ( 'NONE',  ( -8.089106849613333594, -15.02215080929124547, 7.500147780736496017 ) ) ;
#7399=CARTESIAN_POINT ( 'NONE',  ( 1.009606305713754315, -17.02204649693582184, 18.37415474056476938 ) ) ;
#7402=CARTESIAN_POINT ( 'NONE',  ( -14.58213539500865785, 7.758783772730382111, 1.500000000000000000 ) ) ;
#7404=CARTESIAN_POINT ( 'NONE',  ( 14.89413573707702021, 13.37445272932973417, 18.34798005862662507 ) ) ;
#7407=B_SPLINE_CURVE_WITH_KNOTS ( 'NONE', 3,
 ( #20924, #8500, #9089, #20481, #16109, #13321, #20332, #10982, #15489, #20772, #30001, #6284, #15797, #27364, #4102, #1620, #25317, #25629, #18302, #6451 ),
 .UNSPECIFIED., .F., .F.,
 ( 4, 2, 2, 2, 2, 2, 2, 2, 2, 4 ),
 ( 0.000000000000000000, 0.06250000000000054123, 0.1250000000000009714, 0.1875000000000014155, 0.2187500000000014433, 0.2500000000000014433, 0.3125000000000011102, 0.3750000000000007216, 0.4375000000000003886, 0.5000000000000000000 ),
 .UNSPECIFIED. ) ;
#7409=CARTESIAN_POINT ( 'NONE',  ( -14.70423443302406419, -8.686234331489293581, 6.782048567692550378 ) ) ;
#7410=CARTESIAN_POINT ( 'NONE',  ( -5.974095823819629558, 15.97878383974769534, 5.749491821935610147 ) ) ;
#7411=DIRECTION ( 'NONE',  ( 0.000000000000000000, 0.000000000000000000, 1.000000000000000000 ) ) ;
#7414=FACE_OUTER_BOUND ( 'NONE', #5171, .T. ) ;
#7420=CARTESIAN_POINT ( 'NONE',  ( 11.11118388262826784, -16.62953976291649028, 18.34798005863226678 ) ) ;
#7423=CARTESIAN_POINT ( 'NONE',  ( 15.81416692036122207, -6.360574302898111654, 18.34798005863078885 ) ) ;
#7424=AXIS2_PLACEMENT_3D ( 'NONE', #12978, #22469, #12092 ) ;
#7428=CARTESIAN_POINT ( 'NONE',  ( 5.627515464934154998, 19.21053377385552707, 20.29090034784956131 ) ) ;
#7431=DIRECTION ( 'NONE',  ( -1.000000000000000000, 0.000000000000000000, 0.000000000000000000 ) ) ;
#7433=ORIENTED_EDGE ( 'NONE', *, *, #7231, .F. ) ;
#7438=AXIS2_PLACEMENT_3D ( 'NONE', #6914, #13932, #11449 ) ;
#7441=CARTESIAN_POINT ( 'NONE',  ( -15.54251014615009296, -6.943938207015639463, 7.080843742048788414 ) ) ;
#7444=CARTESIAN_POINT ( 'NONE',  ( 0.1277494853664074559, -20.01772078232906793, 5.670038381137163519 ) ) ;
#7445=CARTESIAN_POINT ( 'NONE',  ( 6.812559277181973627, -5.881244434206257310, 1.500000000000001332 ) ) ;
#7451=CARTESIAN_POINT ( 'NONE',  ( 12.37236664230077743, -12.04390635323149716, 1.500000000000000000 ) ) ;
#7458=CYLINDRICAL_SURFACE ( 'NONE', #15895, 0.7500000000000003331 ) ;
#7463=ADVANCED_FACE ( 'NONE', ( #15113, #13259 ), #10920, .F. ) ;
#7466=EDGE_CURVE ( 'NONE', #14242, #18086, #12631, .T. ) ;
#7467=CARTESIAN_POINT ( 'NONE',  ( 18.38343463818524981, -7.922482876633608839, 18.34838970509067479 ) ) ;
#7468=CARTESIAN_POINT ( 'NONE',  ( 19.76051936388921604, 3.198927888044590162, 18.34798005862662507 ) ) ;
#7469=DIRECTION ( 'NONE',  ( -1.000000000000000000, 0.000000000000000000, 0.000000000000000000 ) ) ;
#7470=VERTEX_POINT ( 'NONE', #29944 ) ;
#7478=CARTESIAN_POINT ( 'NONE',  ( -12.72741959552008595, 11.30275801665550794, 19.56050940960062690 ) ) ;
#7481=CARTESIAN_POINT ( 'NONE',  ( -7.747355498299749677, -15.21644541356979907, 18.92976555901915603 ) ) ;
#7483=LINE ( 'NONE', #2019, #23981 ) ;
#7485=CARTESIAN_POINT ( 'NONE',  ( 4.045242219987651211, 16.55840560649980731, 18.34798005863078885 ) ) ;
#7487=CARTESIAN_POINT ( 'NONE',  ( 9.676137610658594568, -14.02562811695957024, 5.670038381137163519 ) ) ;
#7489=CARTESIAN_POINT ( 'NONE',  ( 1.438332125858173605, -8.884323311075778662, 1.500000000000001332 ) ) ;
#7490=ORIENTED_EDGE ( 'NONE', *, *, #18921, .T. ) ;
#7491=ORIENTED_EDGE ( 'NONE', *, *, #28842, .F. ) ;
#7493=DIRECTION ( 'NONE',  ( 0.000000000000000000, 0.000000000000000000, -1.000000000000000000 ) ) ;
#7494=CARTESIAN_POINT ( 'NONE',  ( -5.325396069054047388, 16.18574704710537659, 7.632642797338977658 ) ) ;
#7495=CARTESIAN_POINT ( 'NONE',  ( -15.37836256574693827, -7.321964740028795049, 7.526951045817044772 ) ) ;
#7496=CIRCLE ( 'NONE', #5489, 0.9999999999999983347 ) ;
#7503=CARTESIAN_POINT ( 'NONE',  ( -4.163336342344337027E-14, 1.387778780781445676E-14, 24.50000000000000000 ) ) ;
#7504=ADVANCED_FACE ( 'NONE', ( #13105 ), #1088, .F. ) ;
#7507=CARTESIAN_POINT ( 'NONE',  ( 15.12016594919360557, 13.11846484362264320, 7.595116371587256054 ) ) ;
#7509=CARTESIAN_POINT ( 'NONE',  ( 18.38084888341871093, -7.928499866610141389, 7.652108011868850035 ) ) ;
#7513=ORIENTED_EDGE ( 'NONE', *, *, #13608, .F. ) ;
#7519=AXIS2_PLACEMENT_3D ( 'NONE', #4161, #20396, #27885 ) ;
#7524=CARTESIAN_POINT ( 'NONE',  ( 15.40017468080368168, -7.251222802968046999, 6.910395520694542881 ) ) ;
#7529=DIRECTION ( 'NONE',  ( 0.9898214418809326842, 0.1423148382732852268, -0.000000000000000000 ) ) ;
#7531=EDGE_CURVE ( 'NONE', #24159, #2072, #27100, .T. ) ;
#7538=VERTEX_POINT ( 'NONE', #12102 ) ;
#7541=EDGE_LOOP ( 'NONE', ( #2850, #30169, #15330, #2182 ) ) ;
#7543=DIRECTION ( 'NONE',  ( 1.000000000000000000, 0.000000000000000000, 0.000000000000000000 ) ) ;
#7546=FACE_BOUND ( 'NONE', #11922, .T. ) ;
#7547=ORIENTED_EDGE ( 'NONE', *, *, #4231, .F. ) ;
#7549=DIRECTION ( 'NONE',  ( -0.5406408174555974444, -0.8412535328311813165, -0.000000000000000000 ) ) ;
#7552=DIRECTION ( 'NONE',  ( 1.000000000000000000, 0.000000000000000000, 0.000000000000000000 ) ) ;
#7553=CARTESIAN_POINT ( 'NONE',  ( 1.411528516173252923, -17.00651183856732018, 20.13759033520874908 ) ) ;
#7557=CARTESIAN_POINT ( 'NONE',  ( 14.84329864647545349, 13.43104200419766592, 18.34838970509067479 ) ) ;
#7562=CARTESIAN_POINT ( 'NONE',  ( -14.71031647956046839, -8.675071222119054681, 6.447548852708279377 ) ) ;
#7563=CARTESIAN_POINT ( 'NONE',  ( -6.936828876846345082, 18.77725343618824994, 6.672349528511551497 ) ) ;
#7571=CARTESIAN_POINT ( 'NONE',  ( -4.390207617113899730, 7.856594496258241023, 1.500000000000001332 ) ) ;
#7574=CARTESIAN_POINT ( 'NONE',  ( -12.85282321250444681, 11.16584596974482757, 7.272049892295485485 ) ) ;
#7576=CARTESIAN_POINT ( 'NONE',  ( 0.2758680007048933680, -17.03033689273112827, 5.774779864094944593 ) ) ;
#7577=ORIENTED_EDGE ( 'NONE', *, *, #1377, .F. ) ;
#7580=PLANE ( 'NONE',  #15680 ) ;
#7583=CIRCLE ( 'NONE', #27514, 0.7500000000000006661 ) ;
#7584=DIRECTION ( 'NONE',  ( 0.000000000000000000, 0.000000000000000000, -1.000000000000000000 ) ) ;
#7591=VERTEX_POINT ( 'NONE', #23048 ) ;
#7594=CARTESIAN_POINT ( 'NONE',  ( -0.2093543646724261298, -17.02041581256300873, 6.420335371522007506 ) ) ;
#7595=CARTESIAN_POINT ( 'NONE',  ( 9.056208293496307959, -2.810445847081891824, 1.500000000000001332 ) ) ;
#7598=CARTESIAN_POINT ( 'NONE',  ( 0.000000000000000000, 0.000000000000000000, 1.500000000000001332 ) ) ;
#7599=ORIENTED_EDGE ( 'NONE', *, *, #13371, .F. ) ;
#7600=FACE_BOUND ( 'NONE', #7839, .T. ) ;
#7601=CARTESIAN_POINT ( 'NONE',  ( 4.437794406404241165, 19.50150518896415974, 7.161525567826892313 ) ) ;
#7603=EDGE_LOOP ( 'NONE', ( #28178, #18681, #11755, #5936 ) ) ;
#7604=B_SPLINE_CURVE_WITH_KNOTS ( 'NONE', 3,
 ( #25086, #27901, #13246, #22582, #10586, #1075, #25403, #17926, #27742, #24932, #25550, #4175, #20101, #20552, #22734, #27438, #6524, #18073, #6058, #4030 ),
 .UNSPECIFIED., .F., .F.,
 ( 4, 2, 2, 2, 2, 2, 2, 2, 2, 4 ),
 ( 0.000000000000000000, 0.06250000000000072164, 0.1250000000000014433, 0.1875000000000021649, 0.2187500000000021094, 0.2500000000000020539, 0.3125000000000015543, 0.3750000000000010547, 0.4375000000000005551, 0.5000000000000000000 ),
 .UNSPECIFIED. ) ;
#7607=VERTEX_POINT ( 'NONE', #28332 ) ;
#7608=CARTESIAN_POINT ( 'NONE',  ( 12.43151381881690476, 11.65737597917811996, 18.35377592296120497 ) ) ;
#7611=CARTESIAN_POINT ( 'NONE',  ( -9.002647793593395065, -14.45788447640154395, 5.796888747622817029 ) ) ;
#7612=ORIENTED_EDGE ( 'NONE', *, *, #19112, .T. ) ;
#7613=CIRCLE ( 'NONE', #15579, 1.000000000000007772 ) ;
#7614=CARTESIAN_POINT ( 'NONE',  ( 15.81416324982725818, -6.360572704771151997, 18.34798005862662507 ) ) ;
#7615=CARTESIAN_POINT ( 'NONE',  ( 19.72311808385370213, 3.421819763545495441, 18.37415474056476938 ) ) ;
#7618=CARTESIAN_POINT ( 'NONE',  ( 15.70571165148985315, -6.606148062277499733, 20.32222155561919053 ) ) ;
#7619=ORIENTED_EDGE ( 'NONE', *, *, #8476, .F. ) ;
#7622=CARTESIAN_POINT ( 'NONE',  ( -5.974095823819627782, 15.97878383974769179, 18.44527579819791185 ) ) ;
#7623=CARTESIAN_POINT ( 'NONE',  ( -13.30548897721377699, 10.64932510079500538, 20.34789198813115263 ) ) ;
#7624=CIRCLE ( 'NONE', #4547, 9.482273699623480212 ) ;
#7625=CARTESIAN_POINT ( 'NONE',  ( -9.646222981487634129, -17.54010295177085155, 19.25672174529527325 ) ) ;
#7627=CIRCLE ( 'NONE', #18099, 9.482273699623480212 ) ;
#7630=ORIENTED_EDGE ( 'NONE', *, *, #26922, .T. ) ;
#7633=CARTESIAN_POINT ( 'NONE',  ( 9.135582339684649611, -14.36547911245298259, 7.176035686813569292 ) ) ;
#7635=CARTESIAN_POINT ( 'NONE',  ( 9.439370189418465174, -14.17768557490432002, 5.774779864094943704 ) ) ;
#7636=EDGE_CURVE ( 'NONE', #16019, #25635, #16723, .T. ) ;
#7642=CARTESIAN_POINT ( 'NONE',  ( 18.67144399175157687, -7.167977615171057693, 19.85730954408919757 ) ) ;
#7644=DIRECTION ( 'NONE',  ( -1.000000000000000000, 0.000000000000000000, 0.000000000000000000 ) ) ;
#7647=ADVANCED_FACE ( 'NONE', ( #30807 ), #20566, .F. ) ;
#7651=ADVANCED_FACE ( 'NONE', ( #7253 ), #8723, .T. ) ;
#7653=CARTESIAN_POINT ( 'NONE',  ( 9.634323311075775109, 1.438332125858202692, 21.50000000000000000 ) ) ;
#7667=DIRECTION ( 'NONE',  ( 1.000000000000000000, 0.000000000000000000, 0.000000000000000000 ) ) ;
#7668=DIRECTION ( 'NONE',  ( 0.1423148382732889461, 0.9898214418809321291, 0.000000000000000000 ) ) ;
#7669=CARTESIAN_POINT ( 'NONE',  ( 10.58066667298599661, -16.99307187112385265, 20.12545155307891065 ) ) ;
#7684=ADVANCED_FACE ( 'NONE', ( #19889 ), #852, .F. ) ;
#7689=CARTESIAN_POINT ( 'NONE',  ( -13.00999358272542494, -0.8602714556717691030, 24.50000000000000000 ) ) ;
#7698=FACE_OUTER_BOUND ( 'NONE', #26120, .T. ) ;
#7701=CARTESIAN_POINT ( 'NONE',  ( 12.24063095261064404, 4.490763173670002217, 1.500000000000001332 ) ) ;
#7704=ORIENTED_EDGE ( 'NONE', *, *, #28663, .T. ) ;
#7705=DIRECTION ( 'NONE',  ( 0.2817325568414296710, 0.9594929736144973687, -0.000000000000000000 ) ) ;
#7707=EDGE_CURVE ( 'NONE', #27411, #26330, #700, .T. ) ;
#7711=CARTESIAN_POINT ( 'NONE',  ( 4.299378382534714937, 16.48726736029805195, 18.37259980046034613 ) ) ;
#7716=CARTESIAN_POINT ( 'NONE',  ( 1.230359340266124146, -17.01462811240320150, 5.749491821935610147 ) ) ;
#7721=CARTESIAN_POINT ( 'NONE',  ( -17.63988435498683671, -9.462624493092876676, 6.233981582756856987 ) ) ;
#7722=CARTESIAN_POINT ( 'NONE',  ( -6.065925884476026653, 15.94726461227263847, 5.810767894563978686 ) ) ;
#7724=CARTESIAN_POINT ( 'NONE',  ( -18.24419300814588851, -8.237927942618480159, 18.44501272782439827 ) ) ;
#7725=DIRECTION ( 'NONE',  ( 1.000000000000000000, 0.000000000000000000, 0.000000000000000000 ) ) ;
#7727=VERTEX_POINT ( 'NONE', #2895 ) ;
#7729=AXIS2_PLACEMENT_3D ( 'NONE', #19426, #19893, #22383 ) ;
#7732=CARTESIAN_POINT ( 'NONE',  ( 9.454746441592959627, -0.7220001660362819207, 21.50000000000000000 ) ) ;
#7735=CARTESIAN_POINT ( 'NONE',  ( -2.094186647214675734, 9.248129367672088819, 1.500000000000001332 ) ) ;
#7739=CARTESIAN_POINT ( 'NONE',  ( 19.74328841314634886, 3.194145055459934213, 20.34789198813115263 ) ) ;
#7740=CARTESIAN_POINT ( 'NONE',  ( -8.546423435383418976, -14.74799740001549786, 18.34798005863078885 ) ) ;
#7742=ORIENTED_EDGE ( 'NONE', *, *, #14489, .F. ) ;
#7743=CARTESIAN_POINT ( 'NONE',  ( 11.77411685406913477, -16.16721897189998103, 6.037995405461183296 ) ) ;
#7744=EDGE_CURVE ( 'NONE', #6719, #10258, #21528, .T. ) ;
#7746=CARTESIAN_POINT ( 'NONE',  ( 11.23874228076938664, -11.06161525231356713, -0.6213203435596476032 ) ) ;
#7748=CARTESIAN_POINT ( 'NONE',  ( -18.15569024355515282, -8.431866758338669499, 5.670038381137163519 ) ) ;
#7751=CARTESIAN_POINT ( 'NONE',  ( 0.4458717728788724188, -17.03078575579515430, 5.701226463332907279 ) ) ;
#7752=CARTESIAN_POINT ( 'NONE',  ( -10.00000000000004263, 1.387778780781445676E-14, 24.50000000000000000 ) ) ;
#7754=FACE_OUTER_BOUND ( 'NONE', #2542, .T. ) ;
#7755=CARTESIAN_POINT ( 'NONE',  ( 10.47960520055065992, -7.757439966934453146, 24.50000000000000000 ) ) ;
#7759=ORIENTED_EDGE ( 'NONE', *, *, #23066, .F. ) ;
#7760=ORIENTED_EDGE ( 'NONE', *, *, #8775, .F. ) ;
#7764=CARTESIAN_POINT ( 'NONE',  ( 15.45595318746689273, 12.72131790141721375, 18.80699882434806369 ) ) ;
#7765=AXIS2_PLACEMENT_3D ( 'NONE', #2840, #30762, #2219 ) ;
#7766=CARTESIAN_POINT ( 'NONE',  ( -9.081360402260859388, -14.40588898056578060, 5.862424720655265098 ) ) ;
#7768=CARTESIAN_POINT ( 'NONE',  ( -19.73500371898429862, 3.353449004226453312, 7.176035686813569292 ) ) ;
#7769=CARTESIAN_POINT ( 'NONE',  ( 18.12921809165263198, -8.446683920555065228, 5.775318986477952166 ) ) ;
#7773=VERTEX_POINT ( 'NONE', #5536 ) ;
#7775=VERTEX_POINT ( 'NONE', #7732 ) ;
#7777=CARTESIAN_POINT ( 'NONE',  ( -6.803558837019167527, 18.82611028990652713, 18.82680253904184298 ) ) ;
#7778=CARTESIAN_POINT ( 'NONE',  ( -15.20706373417739599, 13.01805446572691594, 20.32842677360128292 ) ) ;
#7783=DIRECTION ( 'NONE',  ( -0.9898214418809327952, -0.1423148382732853101, 0.000000000000000000 ) ) ;
#7784=VERTEX_POINT ( 'NONE', #24551 ) ;
#7786=AXIS2_PLACEMENT_3D ( 'NONE', #16437, #25951, #11924 ) ;
#7787=CARTESIAN_POINT ( 'NONE',  ( 9.436006877828926775, -14.17980878077545981, 7.526951045817043884 ) ) ;
#7790=CARTESIAN_POINT ( 'NONE',  ( -4.668110441710642711, -19.44758969394387194, 1.500000000000001332 ) ) ;
#7791=CARTESIAN_POINT ( 'NONE',  ( 10.88769261259305310, -16.77715788799338625, 7.626647697317580743 ) ) ;
#7792=CARTESIAN_POINT ( 'NONE',  ( 16.16296542101254730, 5.939519782021115191, -0.6213203435596476032 ) ) ;
#7794=AXIS2_PLACEMENT_3D ( 'NONE', #10081, #12124, #21778 ) ;
#7797=CARTESIAN_POINT ( 'NONE',  ( 6.070111251556830290, 19.05682731086507076, 7.267242832833948896 ) ) ;
#7802=CARTESIAN_POINT ( 'NONE',  ( 16.79425489945617400, 2.861376016183142745, 7.595116371587256054 ) ) ;
#7803=ORIENTED_EDGE ( 'NONE', *, *, #5583, .T. ) ;
#7804=AXIS2_PLACEMENT_3D ( 'NONE', #14616, #567, #22246 ) ;
#7805=CARTESIAN_POINT ( 'NONE',  ( 15.37106698384762993, 12.82394120857653874, 7.359006845440219102 ) ) ;
#7806=ORIENTED_EDGE ( 'NONE', *, *, #11146, .F. ) ;
#7808=CIRCLE ( 'NONE', #5833, 1.000000000000008438 ) ;
#7809=CARTESIAN_POINT ( 'NONE',  ( -7.028330626922778990, 10.93629592680536788, 1.500000000000001332 ) ) ;
#7811=DIRECTION ( 'NONE',  ( -0.000000000000000000, -0.000000000000000000, -1.000000000000000000 ) ) ;
#7817=CARTESIAN_POINT ( 'NONE',  ( -9.824744466605366711, -8.513189541288717521, 24.50000000000000000 ) ) ;
#7820=CARTESIAN_POINT ( 'NONE',  ( -13.89991139849285773, 7.447222512978775022, 1.500000000000001332 ) ) ;
#7822=FACE_OUTER_BOUND ( 'NONE', #11714, .T. ) ;
#7825=AXIS2_PLACEMENT_3D ( 'NONE', #22961, #3959, #18460 ) ;
#7826=CARTESIAN_POINT ( 'NONE',  ( -13.77701868333377178, 10.07013474916661266, 20.13759033520874908 ) ) ;
#7828=ORIENTED_EDGE ( 'NONE', *, *, #26922, .F. ) ;
#7836=CARTESIAN_POINT ( 'NONE',  ( 7.724883619896791842, 5.687793815610376669, 21.50000000000000000 ) ) ;
#7839=EDGE_LOOP ( 'NONE', ( #18769, #882 ) ) ;
#7844=CARTESIAN_POINT ( 'NONE',  ( -18.04365185506139113, -8.627086862512678422, 20.34789198813115263 ) ) ;
#7846=EDGE_CURVE ( 'NONE', #1564, #26699, #18165, .T. ) ;
#7855=ADVANCED_FACE ( 'NONE', ( #20346, #27981, #25494 ), #25170, .T. ) ;
#7857=EDGE_CURVE ( 'NONE', #4888, #13891, #13495, .T. ) ;
#7868=EDGE_CURVE ( 'NONE', #12720, #21119, #16627, .T. ) ;
#7870=B_SPLINE_CURVE_WITH_KNOTS ( 'NONE', 3,
 ( #27952, #1739, #30729, #23547, #7029, #20752, #30433, #13615, #9377, #1894, #25754, #4384, #19040, #18733, #28247, #6581, #6876, #16391 ),
 .UNSPECIFIED., .F., .F.,
 ( 4, 2, 2, 2, 2, 2, 2, 2, 4 ),
 ( 0.000000000000000000, 0.0003967869494442868004, 0.0007935738988885736008, 0.001190360848332860455, 0.001587147797777147202, 0.001983934747221434165, 0.002380721696665720911, 0.002777508646110007657, 0.003174295595554294403 ),
 .UNSPECIFIED. ) ;
#7872=AXIS2_PLACEMENT_3D ( 'NONE', #13814, #16302, #16753 ) ;
#7874=CARTESIAN_POINT ( 'NONE',  ( -5.694318326875604797, 16.07090250511087604, 5.661398277488801867 ) ) ;
#7877=CARTESIAN_POINT ( 'NONE',  ( -18.32390295431236282, -8.059524160852181041, 18.55820869691756769 ) ) ;
#7881=ORIENTED_EDGE ( 'NONE', *, *, #8042, .F. ) ;
#7883=DIRECTION ( 'NONE',  ( 0.000000000000000000, 0.000000000000000000, 1.000000000000000000 ) ) ;
#7892=CIRCLE ( 'NONE', #5900, 1.000000000000007772 ) ;
#7893=ORIENTED_EDGE ( 'NONE', *, *, #8454, .F. ) ;
#7894=CARTESIAN_POINT ( 'NONE',  ( -10.00000000000004263, 1.387778780781445676E-14, 24.50000000000000000 ) ) ;
#7895=EDGE_CURVE ( 'NONE', #27782, #4693, #11294, .T. ) ;
#7896=B_SPLINE_SURFACE_WITH_KNOTS ( 'NONE', 3, 1, ( 
 ( #22780, #18434 ),
 ( #27627, #27475 ),
 ( #6563, #25124 ),
 ( #25444, #15931 ),
 ( #20448, #24970 ),
 ( #8606, #5953 ),
 ( #25591, #1273 ),
 ( #27324, #15451 ),
 ( #13596, #23074 ),
 ( #11237, #8910 ),
 ( #6251, #30264 ),
 ( #3608, #11402 ),
 ( #29656, #1722 ),
 ( #20732, #30113 ),
 ( #16075, #15761 ),
 ( #3929, #3766 ),
 ( #22932, #13285 ),
 ( #13129, #22623 ),
 ( #1435, #11094 ),
 ( #10781, #27785 ),
 ( #20588, #20296 ),
 ( #8293, #29822 ),
 ( #4211, #8744 ),
 ( #6096, #23224 ),
 ( #10950, #15606 ),
 ( #8464, #1878 ),
 ( #17809, #18264 ),
 ( #17966, #13887 ),
 ( #14492, #4982 ),
 ( #23534, #9201 ),
 ( #28539, #23993 ) ),
 .UNSPECIFIED., .F., .F., .F.,
 ( 4, 3, 3, 3, 3, 3, 3, 3, 3, 3, 4 ),
 ( 2, 2 ),
 ( 0.000000000000000000, 0.05425176834609633791, 0.1085332949128352958, 0.1623767749169382768, 0.2157504826133063158, 0.2688657508888171455, 0.3218907763505476360, 0.3749548578363336993, 0.4282048033836242107, 0.4818374082110501444, 0.4999999999131659045 ),
 ( 0.000000000000000000, 1.000000000000000000 ),
 .UNSPECIFIED. ) ;
#7897=CIRCLE ( 'NONE', #25320, 0.7500000000000006661 ) ;
#7899=AXIS2_PLACEMENT_3D ( 'NONE', #24312, #2963, #17609 ) ;
#7900=CARTESIAN_POINT ( 'NONE',  ( -7.671651850954195773, -15.25824679864874511, 19.28454053338349183 ) ) ;
#7902=ORIENTED_EDGE ( 'NONE', *, *, #4599, .T. ) ;
#7903=CARTESIAN_POINT ( 'NONE',  ( 11.62196639741666004, -16.27693748946514418, 5.853797745100183469 ) ) ;
#7907=CARTESIAN_POINT ( 'NONE',  ( -19.82747825358059401, 2.624647641736350234, 18.34726407865098707 ) ) ;
#7908=EDGE_LOOP ( 'NONE', ( #13926, #2087, #8958, #6171 ) ) ;
#7909=DIRECTION ( 'NONE',  ( 0.000000000000000000, -0.000000000000000000, -1.000000000000000000 ) ) ;
#7910=CARTESIAN_POINT ( 'NONE',  ( -4.163336342344337027E-14, 1.387778780781445676E-14, 24.50000000000000000 ) ) ;
#7911=CARTESIAN_POINT ( 'NONE',  ( 15.91781874854195422, -6.122627424449554212, 7.652108011868850035 ) ) ;
#7912=EDGE_CURVE ( 'NONE', #13171, #14352, #29592, .T. ) ;
#7914=CARTESIAN_POINT ( 'NONE',  ( -12.24063095261064227, 4.490763173670005770, 1.500000000000001332 ) ) ;
#7917=DIRECTION ( 'NONE',  ( -0.000000000000000000, -0.000000000000000000, 1.000000000000000000 ) ) ;
#7919=CIRCLE ( 'NONE', #13403, 9.482273699623480212 ) ;
#7920=CARTESIAN_POINT ( 'NONE',  ( 8.840471615930072247, -1.687027447297460236, 21.50000000000000000 ) ) ;
#7921=LINE ( 'NONE', #12746, #18572 ) ;
#7924=AXIS2_PLACEMENT_3D ( 'NONE', #27488, #17980, #15463 ) ;
#7929=ORIENTED_EDGE ( 'NONE', *, *, #4703, .F. ) ;
#7931=AXIS2_PLACEMENT_3D ( 'NONE', #24645, #19813, #7981 ) ;
#7933=CARTESIAN_POINT ( 'NONE',  ( 12.35522127274689375, 11.74279147932066003, 18.34798005862930736 ) ) ;
#7935=CARTESIAN_POINT ( 'NONE',  ( -16.82936799811533035, 2.561302842313196049, 7.080843742048788414 ) ) ;
#7936=CARTESIAN_POINT ( 'NONE',  ( 16.63252861691851692, 3.817440173033144202, 20.13759033520874908 ) ) ;
#7938=VERTEX_POINT ( 'NONE', #10674 ) ;
#7939=DIRECTION ( 'NONE',  ( -0.9096319953545183301, -0.4154150130018863796, -0.000000000000000000 ) ) ;
#7944=ORIENTED_EDGE ( 'NONE', *, *, #18508, .T. ) ;
#7947=CARTESIAN_POINT ( 'NONE',  ( 16.60164139905475267, 3.971857776421113595, 7.280727868105637768 ) ) ;
#7948=CARTESIAN_POINT ( 'NONE',  ( -14.72475726066618051, 13.56098618572340619, 19.00652017443069752 ) ) ;
#7950=DIRECTION ( 'NONE',  ( -0.000000000000000000, -0.000000000000000000, 1.000000000000000000 ) ) ;
#7954=ORIENTED_EDGE ( 'NONE', *, *, #8534, .F. ) ;
#7955=CARTESIAN_POINT ( 'NONE',  ( -19.92178149465837578, 1.957245511797580217, 5.810767894563978686 ) ) ;
#7962=DIRECTION ( 'NONE',  ( 0.1423148382732746797, -0.9898214418809342385, 0.000000000000000000 ) ) ;
#7964=CARTESIAN_POINT ( 'NONE',  ( 18.67280747382547190, -7.164419611389371667, 18.84486140012301547 ) ) ;
#7965=EDGE_LOOP ( 'NONE', ( #19488, #8423 ) ) ;
#7968=EDGE_CURVE ( 'NONE', #12097, #2241, #13336, .T. ) ;
#7970=CARTESIAN_POINT ( 'NONE',  ( 6.962021646281529641, 6.437683520590196551, 13.00000000000000178 ) ) ;
#7972=CARTESIAN_POINT ( 'NONE',  ( -10.29013980557132690, -17.15015428632898775, 20.32200205377525393 ) ) ;
#7974=CARTESIAN_POINT ( 'NONE',  ( 11.72050123711542113, 12.41739018441317910, 6.233981582756856987 ) ) ;
#7975=CARTESIAN_POINT ( 'NONE',  ( 19.76130408545751749, 3.194145055459935101, 7.652108011868850035 ) ) ;
#7977=CARTESIAN_POINT ( 'NONE',  ( -5.604556300746500241, -15.53790034020399169, -0.6213203435596476032 ) ) ;
#7979=DIRECTION ( 'NONE',  ( 1.000000000000000000, 1.734723475976805517E-15, 0.000000000000000000 ) ) ;
#7981=DIRECTION ( 'NONE',  ( -1.000000000000000000, 0.000000000000000000, 0.000000000000000000 ) ) ;
#7983=CARTESIAN_POINT ( 'NONE',  ( 3.685570353517261477, -16.10136545388692397, 1.500000000000000000 ) ) ;
#7984=EDGE_LOOP ( 'NONE', ( #26934, #11570, #12128, #27524 ) ) ;
#7990=CARTESIAN_POINT ( 'NONE',  ( 10.92346103252092604, -16.77505673787610974, 20.32842677360128292 ) ) ;
#7991=ORIENTED_EDGE ( 'NONE', *, *, #15918, .F. ) ;
#7995=CARTESIAN_POINT ( 'NONE',  ( -13.59632618586111619, 10.29740991163845010, 18.39992786714538298 ) ) ;
#8000=DIRECTION ( 'NONE',  ( -0.5406408174555976665, 0.8412535328311812055, 0.000000000000000000 ) ) ;
#8004=EDGE_CURVE ( 'NONE', #7607, #26631, #25022, .T. ) ;
#8014=CARTESIAN_POINT ( 'NONE',  ( -9.982956658368037139, -17.33059308371925766, 7.454606537396337274 ) ) ;
#8023=DIRECTION ( 'NONE',  ( -0.000000000000000000, -0.000000000000000000, 1.000000000000000000 ) ) ;
#8025=FACE_OUTER_BOUND ( 'NONE', #6084, .T. ) ;
#8028=CARTESIAN_POINT ( 'NONE',  ( -18.06093561247157808, -8.632161831585827727, 7.652108011868850035 ) ) ;
#8029=CARTESIAN_POINT ( 'NONE',  ( -6.737371319102178013, 18.84978071134531064, 6.041646659195333058 ) ) ;
#8030=CARTESIAN_POINT ( 'NONE',  ( 10.46384303394386528, -13.48464439008897919, 5.951255046771932733 ) ) ;
#8031=EDGE_CURVE ( 'NONE', #14465, #681, #10766, .T. ) ;
#8034=AXIS2_PLACEMENT_3D ( 'NONE', #1656, #22692, #22546 ) ;
#8038=DIRECTION ( 'NONE',  ( -0.2817325568414292825, -0.9594929736144974797, 0.000000000000000000 ) ) ;
#8040=DIRECTION ( 'NONE',  ( 0.000000000000000000, 0.000000000000000000, -1.000000000000000000 ) ) ;
#8041=CARTESIAN_POINT ( 'NONE',  ( -13.02951369420309469, 10.96858531083378452, 5.796888747622817029 ) ) ;
#8042=EDGE_CURVE ( 'NONE', #12536, #17576, #20937, .T. ) ;
#8043=CARTESIAN_POINT ( 'NONE',  ( -0.02788623102222363703, -17.02558298240596102, 7.267659094423557953 ) ) ;
#8044=VERTEX_POINT ( 'NONE', #30771 ) ;
#8045=PLANE ( 'NONE',  #2952 ) ;
#8046=CARTESIAN_POINT ( 'NONE',  ( 9.958038337755681368, 17.34466697471553331, 24.50000000000000000 ) ) ;
#8050=CARTESIAN_POINT ( 'NONE',  ( -7.695850205855595760, -15.24499612925306913, 19.61324152429826739 ) ) ;
#8052=ORIENTED_EDGE ( 'NONE', *, *, #24489, .F. ) ;
#8054=ADVANCED_FACE ( 'NONE', ( #23902 ), #18773, .F. ) ;
#8055=AXIS2_PLACEMENT_3D ( 'NONE', #13151, #22642, #17993 ) ;
#8060=CARTESIAN_POINT ( 'NONE',  ( 13.01334791338956975, 10.97165762312710946, 19.21496526180054332 ) ) ;
#8061=CARTESIAN_POINT ( 'NONE',  ( 16.14871318124067301, -5.543368461261742652, 6.147510495896839622 ) ) ;
#8078=ADVANCED_FACE ( 'NONE', ( #21407, #2226, #25795 ), #30461, .T. ) ;
#8079=CIRCLE ( 'NONE', #22016, 0.7500000000000006661 ) ;
#8080=CARTESIAN_POINT ( 'NONE',  ( 6.778663211761462470, -6.630478080506934546, 13.00000000000000178 ) ) ;
#8081=EDGE_CURVE ( 'NONE', #19471, #29398, #25940, .T. ) ;
#8082=ORIENTED_EDGE ( 'NONE', *, *, #29543, .F. ) ;
#8084=CARTESIAN_POINT ( 'NONE',  ( -19.70934530863873135, 3.501268498360765147, 6.755862304746362845 ) ) ;
#8087=ORIENTED_EDGE ( 'NONE', *, *, #25559, .T. ) ;
#8088=CARTESIAN_POINT ( 'NONE',  ( -5.292460273040080487, 16.19569186415849060, 20.32222155561919053 ) ) ;
#8089=EDGE_LOOP ( 'NONE', ( #11121, #17191, #27616, #29872 ) ) ;
#8096=CARTESIAN_POINT ( 'NONE',  ( 16.63252861691852758, 3.817440173033142425, 7.441806358946449151 ) ) ;
#8097=DIRECTION ( 'NONE',  ( 0.000000000000000000, 0.000000000000000000, -1.000000000000000000 ) ) ;
#8099=CARTESIAN_POINT ( 'NONE',  ( -8.172867764805138435, -14.97344430594795739, 20.25542030744407640 ) ) ;
#8104=CARTESIAN_POINT ( 'NONE',  ( 9.048061653868893828, -14.41834352799975960, 6.974106381145714018 ) ) ;
#8110=AXIS2_PLACEMENT_3D ( 'NONE', #5386, #12413, #10061 ) ;
#8114=CARTESIAN_POINT ( 'NONE',  ( -5.865338193562681823, 19.13956943172005865, 7.652108011868850035 ) ) ;
#8120=ORIENTED_EDGE ( 'NONE', *, *, #1967, .T. ) ;
#8121=CARTESIAN_POINT ( 'NONE',  ( -9.819201815016002755, -17.42389611976320296, 19.96797677718663522 ) ) ;
#8123=CARTESIAN_POINT ( 'NONE',  ( 16.83427080350348248, 2.570616772381430604, 5.862424720655265098 ) ) ;
#8129=VERTEX_POINT ( 'NONE', #12205 ) ;
#8131=CARTESIAN_POINT ( 'NONE',  ( 4.782940318440153327, 19.43789448792816543, 7.500147780736496017 ) ) ;
#8139=CARTESIAN_POINT ( 'NONE',  ( 10.68464666747176750, -16.90719797777717304, 18.47110296274026098 ) ) ;
#8140=ORIENTED_EDGE ( 'NONE', *, *, #30686, .F. ) ;
#8142=B_SPLINE_CURVE_WITH_KNOTS ( 'NONE', 3,
 ( #13165, #6289, #13488, #24868, #27663, #15802, #3505, #29692, #22506, #20634, #3802, #30152, #8339, #8781, #18308, #20336, #5679, #15175, #1150, #17853 ),
 .UNSPECIFIED., .F., .F.,
 ( 4, 2, 2, 2, 2, 2, 2, 2, 2, 4 ),
 ( 0.000000000000000000, 0.06250000000000044409, 0.1250000000000008882, 0.1875000000000013323, 0.2187500000000013600, 0.2500000000000013878, 0.3125000000000010547, 0.3750000000000007216, 0.4375000000000003886, 0.5000000000000000000 ),
 .UNSPECIFIED. ) ;
#8143=CARTESIAN_POINT ( 'NONE',  ( -15.89252301733159989, 12.17122019226247431, 19.89182036555910571 ) ) ;
#8146=ORIENTED_EDGE ( 'NONE', *, *, #28220, .F. ) ;
#8149=B_SPLINE_SURFACE_WITH_KNOTS ( 'NONE', 3, 1, ( 
 ( #17907, #12756 ),
 ( #22565, #26808 ),
 ( #10718, #15391 ),
 ( #24447, #24915 ),
 ( #3395, #3088 ),
 ( #3712, #1060 ),
 ( #10248, #13225 ),
 ( #22713, #29133 ),
 ( #24595, #12923 ),
 ( #7768, #3552 ),
 ( #17275, #7935 ),
 ( #19762, #12609 ),
 ( #17441, #22259 ),
 ( #8084, #30056 ),
 ( #18517, #4475 ),
 ( #8847, #13834 ),
 ( #6798, #3860 ),
 ( #27883, #20980 ),
 ( #11033, #18662 ),
 ( #28168, #16323 ),
 ( #6504, #6352 ),
 ( #18207, #18054 ),
 ( #15700, #15865 ),
 ( #28018, #30365 ),
 ( #9146, #13384 ),
 ( #13687, #22875 ),
 ( #1824, #11346 ),
 ( #4303, #25681 ),
 ( #6197, #25841 ),
 ( #6651, #20681 ),
 ( #18372, #23018 ) ),
 .UNSPECIFIED., .F., .F., .F.,
 ( 4, 3, 3, 3, 3, 3, 3, 3, 3, 3, 4 ),
 ( 2, 2 ),
 ( 0.000000000000000000, 0.05425176834609633791, 0.1085332949128352958, 0.1623767749169382768, 0.2157504826133063158, 0.2688657508888171455, 0.3218907763505476360, 0.3749548578363336993, 0.4282048033836242107, 0.4818374082110501444, 0.4999999999131655715 ),
 ( 0.000000000000000000, 1.000000000000000000 ),
 .UNSPECIFIED. ) ;
#8150=CARTESIAN_POINT ( 'NONE',  ( 12.76513901707091492, 11.27219777367672648, 7.453286057244485008 ) ) ;
#8153=CARTESIAN_POINT ( 'NONE',  ( 6.974883619896790954, 5.687793815610376669, 1.500000000000001332 ) ) ;
#8154=CYLINDRICAL_SURFACE ( 'NONE', #18864, 0.7500000000000007772 ) ;
#8156=CARTESIAN_POINT ( 'NONE',  ( 16.78403870108500584, 2.933703390053540527, 7.626437579292367097 ) ) ;
#8160=DIRECTION ( 'NONE',  ( 0.000000000000000000, 0.000000000000000000, 1.000000000000000000 ) ) ;
#8163=ORIENTED_EDGE ( 'NONE', *, *, #16475, .T. ) ;
#8164=CARTESIAN_POINT ( 'NONE',  ( -8.499586724479453181, -2.959227181723774525, 1.500000000000001332 ) ) ;
#8165=VERTEX_POINT ( 'NONE', #29201 ) ;
#8167=CARTESIAN_POINT ( 'NONE',  ( -15.34618031767422863, 12.82553819247483951, 5.652196082369963293 ) ) ;
#8170=DIRECTION ( 'NONE',  ( 0.000000000000000000, 0.000000000000000000, 1.000000000000000000 ) ) ;
#8173=CARTESIAN_POINT ( 'NONE',  ( 3.474270935886293543, -15.38174572367601911, 1.500000000000001332 ) ) ;
#8174=CARTESIAN_POINT ( 'NONE',  ( -2.810445847081922022, -9.056208293496300854, 1.500000000000001332 ) ) ;
#8176=VECTOR ( 'NONE', #30316, 1000.000000000000000 ) ;
#8179=CARTESIAN_POINT ( 'NONE',  ( -5.973959739936658409, 19.10558604466630328, 7.652108011868850035 ) ) ;
#8180=CARTESIAN_POINT ( 'NONE',  ( 10.39243974596413445, -13.53611166824776646, 5.872146474157316831 ) ) ;
#8184=ORIENTED_EDGE ( 'NONE', *, *, #21177, .T. ) ;
#8185=DIRECTION ( 'NONE',  ( 0.000000000000000000, 0.000000000000000000, 1.000000000000000000 ) ) ;
#8187=CARTESIAN_POINT ( 'NONE',  ( -13.09601454503479268, 10.89247868135537267, 5.749228751562096562 ) ) ;
#8188=CARTESIAN_POINT ( 'NONE',  ( 2.703030265324084080, -12.75514121382991384, 1.500000000000001332 ) ) ;
#8191=CARTESIAN_POINT ( 'NONE',  ( 15.81223572262636878, -6.365019322297388094, 20.34789198813115263 ) ) ;
#8193=ORIENTED_EDGE ( 'NONE', *, *, #578, .T. ) ;
#8198=ORIENTED_EDGE ( 'NONE', *, *, #16853, .T. ) ;
#8199=CARTESIAN_POINT ( 'NONE',  ( 11.22181534970138905, -16.55562029408563163, 5.652912763329821288 ) ) ;
#8202=CARTESIAN_POINT ( 'NONE',  ( -1.246245039005656974, 2.728895986063601509, 24.50000000000000000 ) ) ;
#8204=ORIENTED_EDGE ( 'NONE', *, *, #13955, .F. ) ;
#8206=CARTESIAN_POINT ( 'NONE',  ( -1.246245039005721811, -2.728895986063572643, 24.50000000000000000 ) ) ;
#8207=DIRECTION ( 'NONE',  ( -0.000000000000000000, -0.000000000000000000, -1.000000000000000000 ) ) ;
#8215=ORIENTED_EDGE ( 'NONE', *, *, #25909, .T. ) ;
#8216=CARTESIAN_POINT ( 'NONE',  ( 7.974144905643786529, 5.130938270761634890, 21.50000000000000000 ) ) ;
#8217=CARTESIAN_POINT ( 'NONE',  ( 4.512576344050363453, 19.48449473338812510, 7.272192800924343281 ) ) ;
#8220=ORIENTED_EDGE ( 'NONE', *, *, #26378, .F. ) ;
#8226=CARTESIAN_POINT ( 'NONE',  ( -5.549075634136965363, 16.11684027513961226, 18.34798005863078885 ) ) ;
#8227=CARTESIAN_POINT ( 'NONE',  ( 12.82328378257164303, 11.20259424400690840, 18.63641924841378028 ) ) ;
#8230=LINE ( 'NONE', #24750, #9804 ) ;
#8231=CARTESIAN_POINT ( 'NONE',  ( 19.70572240696341382, 3.522277800415037685, 20.29915277494337644 ) ) ;
#8234=CARTESIAN_POINT ( 'NONE',  ( -5.296822449995211457, 16.19439135686744180, 18.37259980046033547 ) ) ;
#8235=AXIS2_PLACEMENT_3D ( 'NONE', #12843, #4087, #2194 ) ;
#8238=ADVANCED_FACE ( 'NONE', ( #26563 ), #26878, .T. ) ;
#8243=EDGE_CURVE ( 'NONE', #3557, #28757, #19639, .T. ) ;
#8245=CARTESIAN_POINT ( 'NONE',  ( 16.57326105224178647, 4.109591991357616436, 6.233981582756856987 ) ) ;
#8246=CARTESIAN_POINT ( 'NONE',  ( -14.88989150774293790, 13.37932992012220623, 18.63641924841378028 ) ) ;
#8248=EDGE_CURVE ( 'NONE', #10258, #30397, #7483, .T. ) ;
#8250=CARTESIAN_POINT ( 'NONE',  ( -10.47960520055065636, -7.757439966934454034, 24.50000000000000000 ) ) ;
#8251=FACE_OUTER_BOUND ( 'NONE', #1674, .T. ) ;
#8254=DIRECTION ( 'NONE',  ( 0.7557495743542581579, 0.6548607339452852116, 0.000000000000000000 ) ) ;
#8255=CARTESIAN_POINT ( 'NONE',  ( 9.991354877675737711, -13.81564317159775257, 18.35718225375110180 ) ) ;
#8257=VERTEX_POINT ( 'NONE', #16835 ) ;
#8261=CARTESIAN_POINT ( 'NONE',  ( 17.96688762764192759, -8.785985129476815203, 18.84056766331480404 ) ) ;
#8263=CARTESIAN_POINT ( 'NONE',  ( -5.025762778208111570, 19.37674427759095508, 6.864725433338323413 ) ) ;
#8264=EDGE_LOOP ( 'NONE', ( #10443, #30740, #10239, #21563 ) ) ;
#8267=CARTESIAN_POINT ( 'NONE',  ( -4.622016212553093695, -12.19167610014704906, 1.500000000000001332 ) ) ;
#8268=ORIENTED_EDGE ( 'NONE', *, *, #4112, .T. ) ;
#8269=DIRECTION ( 'NONE',  ( 0.000000000000000000, 0.000000000000000000, -1.000000000000000000 ) ) ;
#8271=CYLINDRICAL_SURFACE ( 'NONE', #2274, 0.7500000000000006661 ) ;
#8272=CARTESIAN_POINT ( 'NONE',  ( 16.86926274317445618, 2.283828795636142495, 7.080843742048788414 ) ) ;
#8273=ORIENTED_EDGE ( 'NONE', *, *, #4791, .F. ) ;
#8274=CARTESIAN_POINT ( 'NONE',  ( 12.50580948684386406, 11.57370347876661576, 5.670038381137163519 ) ) ;
#8278=ADVANCED_FACE ( 'NONE', ( #28688 ), #28848, .F. ) ;
#8281=EDGE_CURVE ( 'NONE', #1147, #22188, #22493, .T. ) ;
#8284=CARTESIAN_POINT ( 'NONE',  ( 4.339153914952783353, 19.54170514621186783, 6.892848776733236704 ) ) ;
#8289=CARTESIAN_POINT ( 'NONE',  ( 9.669732009941350626, -14.02977311367122937, 20.32842677360128292 ) ) ;
#8290=CARTESIAN_POINT ( 'NONE',  ( 16.74328840634221649, 3.194145055459935101, 20.34789198813115263 ) ) ;
#8293=CARTESIAN_POINT ( 'NONE',  ( 18.05613910678267331, -8.642405844459421616, 5.940635272151477686 ) ) ;
#8294=CARTESIAN_POINT ( 'NONE',  ( -15.40675500887359384, 12.78077869785448151, 18.34838970509067479 ) ) ;
#8297=LINE ( 'NONE', #27327, #28840 ) ;
#8301=DIRECTION ( 'NONE',  ( -0.000000000000000000, -0.000000000000000000, 1.000000000000000000 ) ) ;
#8302=CARTESIAN_POINT ( 'NONE',  ( -5.548724899233042684, 19.23375410423648191, 20.25336174263950184 ) ) ;
#8313=ORIENTED_EDGE ( 'NONE', *, *, #5986, .T. ) ;
#8315=ORIENTED_EDGE ( 'NONE', *, *, #24835, .T. ) ;
#8317=CARTESIAN_POINT ( 'NONE',  ( -9.131494062835630032, -2.555255504830938218, 1.500000000000001332 ) ) ;
#8318=CARTESIAN_POINT ( 'NONE',  ( -19.93457197822651850, 1.617270501065022126, 19.85730954408917981 ) ) ;
#8319=VECTOR ( 'NONE', #24229, 1000.000000000000000 ) ;
#8321=ORIENTED_EDGE ( 'NONE', *, *, #578, .F. ) ;
#8326=DIRECTION ( 'NONE',  ( 0.000000000000000000, 0.000000000000000000, 1.000000000000000000 ) ) ;
#8327=VECTOR ( 'NONE', #27068, 1000.000000000000000 ) ;
#8329=VECTOR ( 'NONE', #29722, 1000.000000000000000 ) ;
#8331=LINE ( 'NONE', #29227, #10616 ) ;
#8332=CARTESIAN_POINT ( 'NONE',  ( 0.6919288935074161540, -20.00608154967866881, 5.704143890883081269 ) ) ;
#8337=CARTESIAN_POINT ( 'NONE',  ( -10.81179434590808697, -16.84691785479785864, 20.29090034784956131 ) ) ;
#8338=CARTESIAN_POINT ( 'NONE',  ( -14.75084321123812003, -8.599826344683139112, 7.098451512883313441 ) ) ;
#8339=CARTESIAN_POINT ( 'NONE',  ( -4.600690885565751564, 16.38836304891476914, 6.385774490351136201 ) ) ;
#8340=CARTESIAN_POINT ( 'NONE',  ( 11.94785300146925522, -16.06093515404948135, 6.560937769032974209 ) ) ;
#8350=CARTESIAN_POINT ( 'NONE',  ( 3.094187858404264357, 16.79444423853821533, 6.392658652357121163 ) ) ;
#8351=VECTOR ( 'NONE', #23518, 1000.000000000000000 ) ;
#8353=CARTESIAN_POINT ( 'NONE',  ( -11.36561296172221169, -16.47845303048202936, 6.530762810602277924 ) ) ;
#8359=CARTESIAN_POINT ( 'NONE',  ( 19.56075217167569846, 4.168887357664726068, 19.08830981656264214 ) ) ;
#8361=CARTESIAN_POINT ( 'NONE',  ( 11.91611018267553490, -16.06265986513585275, 6.919864475265772974 ) ) ;
#8366=ORIENTED_EDGE ( 'NONE', *, *, #28881, .T. ) ;
#8367=LINE ( 'NONE', #27398, #19290 ) ;
#8368=CARTESIAN_POINT ( 'NONE',  ( 17.75446986341059841, 9.207540381081344094, 24.50000000000000000 ) ) ;
#8370=DIRECTION ( 'NONE',  ( 1.000000000000000000, 0.000000000000000000, 0.000000000000000000 ) ) ;
#8371=VECTOR ( 'NONE', #22422, 1000.000000000000000 ) ;
#8376=CYLINDRICAL_SURFACE ( 'NONE', #27845, 1.000000000000011324 ) ;
#8379=CARTESIAN_POINT ( 'NONE',  ( -9.288552932812276453, -14.26664216879104430, 18.83976166372255534 ) ) ;
#8381=EDGE_LOOP ( 'NONE', ( #16352, #19369, #22133, #11079 ) ) ;
#8384=VECTOR ( 'NONE', #758, 1000.000000000000000 ) ;
#8394=EDGE_CURVE ( 'NONE', #20108, #19511, #30426, .T. ) ;
#8398=CARTESIAN_POINT ( 'NONE',  ( 14.96983285839275268, 13.26353275515934982, 7.652108011868850035 ) ) ;
#8401=PLANE ( 'NONE',  #5377 ) ;
#8402=ORIENTED_EDGE ( 'NONE', *, *, #25241, .T. ) ;
#8405=CARTESIAN_POINT ( 'NONE',  ( -6.096671963363472280, 19.04856480014127840, 20.34789198813115618 ) ) ;
#8408=CARTESIAN_POINT ( 'NONE',  ( 19.59127448685153539, 4.109591991357616436, 6.233981582756856987 ) ) ;
#8410=VECTOR ( 'NONE', #8023, 1000.000000000000000 ) ;
#8415=CARTESIAN_POINT ( 'NONE',  ( -19.93913687200723572, 1.772791844786497872, 18.64703902303423178 ) ) ;
#8416=LINE ( 'NONE', #13556, #9866 ) ;
#8418=PLANE ( 'NONE',  #16776 ) ;
#8419=CARTESIAN_POINT ( 'NONE',  ( 11.48757468322166986, -16.39371511241313328, 18.44527579819791185 ) ) ;
#8422=ORIENTED_EDGE ( 'NONE', *, *, #20630, .F. ) ;
#8423=ORIENTED_EDGE ( 'NONE', *, *, #13745, .T. ) ;
#8425=EDGE_CURVE ( 'NONE', #8747, #29572, #20995, .T. ) ;
#8426=CARTESIAN_POINT ( 'NONE',  ( 11.11118051879627799, -16.62953239715189824, 5.652196082369963293 ) ) ;
#8428=B_SPLINE_CURVE_WITH_KNOTS ( 'NONE', 3,
 ( #30501, #23479, #27571, #10881, #20392, #1975, #29914, #30207, #8551, #25216, #11185, #1525, #27720, #25381, #13537, #20535, #4011, #16014 ),
 .UNSPECIFIED., .F., .F.,
 ( 4, 2, 2, 2, 2, 2, 2, 2, 4 ),
 ( 0.003174295595554272285, 0.003570702171545501145, 0.003967108747536730005, 0.004363515323527957998, 0.004759921899519186858, 0.005156328475510415718, 0.005552735051501644578, 0.005949141627492873438, 0.006345548203484102298 ),
 .UNSPECIFIED. ) ;
#8429=CARTESIAN_POINT ( 'NONE',  ( -4.573183673931451310, 16.39543396787673402, 6.755862304746362845 ) ) ;
#8433=B_SPLINE_CURVE_WITH_KNOTS ( 'NONE', 3,
 ( #16556, #24031, #19203, #2677, #26073, #23886, #9856, #28572, #7524, #13922, #16411, #9398, #21223, #4708, #2058, #11581, #21073, #30596, #7202, #23567 ),
 .UNSPECIFIED., .F., .F.,
 ( 4, 2, 2, 2, 2, 2, 2, 2, 2, 4 ),
 ( 0.000000000000000000, 0.06250000000000076328, 0.1250000000000012212, 0.1875000000000016653, 0.2187500000000017208, 0.2500000000000017764, 0.3125000000000014433, 0.3750000000000010547, 0.4375000000000007216, 0.5000000000000000000 ),
 .UNSPECIFIED. ) ;
#8436=DIRECTION ( 'NONE',  ( -0.000000000000000000, -0.000000000000000000, 1.000000000000000000 ) ) ;
#8437=ORIENTED_EDGE ( 'NONE', *, *, #26378, .T. ) ;
#8443=CARTESIAN_POINT ( 'NONE',  ( 19.79689803950977378, 2.967719242317201633, 7.632642797338977658 ) ) ;
#8445=CARTESIAN_POINT ( 'NONE',  ( 14.94527285076313916, 13.31737086058187458, 5.653912893140659257 ) ) ;
#8451=AXIS2_PLACEMENT_3D ( 'NONE', #6106, #13463, #18584 ) ;
#8454=EDGE_CURVE ( 'NONE', #13705, #21089, #15014, .T. ) ;
#8455=CARTESIAN_POINT ( 'NONE',  ( 4.313865120791889218, 19.54726060313607050, 6.560937769032974209 ) ) ;
#8461=CARTESIAN_POINT ( 'NONE',  ( -2.662523238938575343, -12.47340865698848056, 1.500000000000001332 ) ) ;
#8463=CARTESIAN_POINT ( 'NONE',  ( -19.77136997667518514, 3.131761183015793204, 20.12545155307891065 ) ) ;
#8464=CARTESIAN_POINT ( 'NONE',  ( 18.21588581002256646, -8.300927319590593711, 5.701226463332907279 ) ) ;
#8465=CARTESIAN_POINT ( 'NONE',  ( -15.98876933090332919, 12.04425525511918238, 19.25672174529527325 ) ) ;
#8468=VERTEX_POINT ( 'NONE', #20698 ) ;
#8469=EDGE_CURVE ( 'NONE', #30552, #17265, #13554, .T. ) ;
#8470=CARTESIAN_POINT ( 'NONE',  ( -15.34307810681595718, 12.82926163924266483, 7.652108011868850035 ) ) ;
#8472=CARTESIAN_POINT ( 'NONE',  ( -5.544451646083596863, 16.11829163520481956, 20.34789198813115263 ) ) ;
#8476=EDGE_CURVE ( 'NONE', #1130, #17481, #27454, .T. ) ;
#8480=EDGE_CURVE ( 'NONE', #18371, #9025, #27275, .T. ) ;
#8482=DIRECTION ( 'NONE',  ( 1.000000000000000000, 0.000000000000000000, 0.000000000000000000 ) ) ;
#8483=DIRECTION ( 'NONE',  ( 1.000000000000000000, 0.000000000000000000, 0.000000000000000000 ) ) ;
#8488=CARTESIAN_POINT ( 'NONE',  ( -19.69679205574296788, 3.469720661875622891, 6.913388067999415298 ) ) ;
#8490=EDGE_LOOP ( 'NONE', ( #7893, #13931, #15623, #23623 ) ) ;
#8493=CARTESIAN_POINT ( 'NONE',  ( -0.1262659238204836554, -8.999114229549588728, 21.50000000000000000 ) ) ;
#8495=VECTOR ( 'NONE', #13470, 1000.000000000000000 ) ;
#8496=CARTESIAN_POINT ( 'NONE',  ( -5.549074438232175055, 16.11683645458453995, 18.34798005862662507 ) ) ;
#8498=CARTESIAN_POINT ( 'NONE',  ( 11.10715495309692891, -16.63223102436628409, 7.652108011868850035 ) ) ;
#8500=CARTESIAN_POINT ( 'NONE',  ( -16.94861615807197097, 1.782241101862044319, 7.652108011868850923 ) ) ;
#8501=ORIENTED_EDGE ( 'NONE', *, *, #21277, .T. ) ;
#8505=CARTESIAN_POINT ( 'NONE',  ( -9.159129059799163031, -14.35414742152909362, 20.05479082170252525 ) ) ;
#8506=CARTESIAN_POINT ( 'NONE',  ( -17.86647173498021246, -9.028149653223252358, 7.559636331181775581 ) ) ;
#8507=CARTESIAN_POINT ( 'NONE',  ( -6.290842788517061912, 19.00387417064636253, 7.603368798681074736 ) ) ;
#8508=CARTESIAN_POINT ( 'NONE',  ( 11.56680498864186291, -16.33760111733342413, 5.810767894563978686 ) ) ;
#8511=VERTEX_POINT ( 'NONE', #30074 ) ;
#8521=CARTESIAN_POINT ( 'NONE',  ( -11.19942626343432046, -16.59192963269641652, 7.272049892295485485 ) ) ;
#8526=DIRECTION ( 'NONE',  ( -0.000000000000000000, -0.000000000000000000, 1.000000000000000000 ) ) ;
#8531=CIRCLE ( 'NONE', #15995, 0.7500000000000004441 ) ;
#8532=CARTESIAN_POINT ( 'NONE',  ( -17.02500080809207361, 1.126395502097476520, 5.759928666072748449 ) ) ;
#8534=EDGE_CURVE ( 'NONE', #14561, #17054, #20010, .T. ) ;
#8538=CARTESIAN_POINT ( 'NONE',  ( 9.860909914091287476, -13.90333503830274609, 7.652108011868850923 ) ) ;
#8539=DIRECTION ( 'NONE',  ( 1.000000000000000000, 0.000000000000000000, 0.000000000000000000 ) ) ;
#8545=DIRECTION ( 'NONE',  ( -0.000000000000000000, -0.000000000000000000, 1.000000000000000000 ) ) ;
#8548=DIRECTION ( 'NONE',  ( 0.000000000000000000, 0.000000000000000000, 1.000000000000000000 ) ) ;
#8551=CARTESIAN_POINT ( 'NONE',  ( -11.35999944890269830, -16.46057145267183586, 19.47728749465736442 ) ) ;
#8552=CARTESIAN_POINT ( 'NONE',  ( -8.550548372801090480, -14.74545326687210434, 20.34789198813115263 ) ) ;
#8553=AXIS2_PLACEMENT_3D ( 'NONE', #6781, #4455, #13963 ) ;
#8554=CARTESIAN_POINT ( 'NONE',  ( -10.55542352351189095, -17.00870908956209249, 18.34777357837151968 ) ) ;
#8557=CARTESIAN_POINT ( 'NONE',  ( 8.413215745754998309, -3.196529495465417980, 1.500000000000001332 ) ) ;
#8561=VERTEX_POINT ( 'NONE', #1390 ) ;
#8562=CARTESIAN_POINT ( 'NONE',  ( -6.102995743689038299, 19.04655207687856233, 18.34869673959211767 ) ) ;
#8566=CARTESIAN_POINT ( 'NONE',  ( -13.23566211985188446, 10.73140863935235600, 18.36582235739946611 ) ) ;
#8567=CARTESIAN_POINT ( 'NONE',  ( 1.590931199584701305, -16.99685872687011212, 6.037360021877312910 ) ) ;
#8569=CARTESIAN_POINT ( 'NONE',  ( -19.87079772360653607, 2.422354609568011519, 18.34838970509067479 ) ) ;
#8578=DIRECTION ( 'NONE',  ( -0.4154150130018840481, 0.9096319953545194403, 0.000000000000000000 ) ) ;
#8579=CARTESIAN_POINT ( 'NONE',  ( -5.762218391735200562, 19.17087124927422437, 5.670038381137163519 ) ) ;
#8580=VERTEX_POINT ( 'NONE', #23804 ) ;
#8582=CARTESIAN_POINT ( 'NONE',  ( -12.84881549437216819, 11.17046077493017897, 7.267659094423557065 ) ) ;
#8584=EDGE_LOOP ( 'NONE', ( #30779, #9816, #12208, #17630 ) ) ;
#8585=VECTOR ( 'NONE', #29474, 1000.000000000000227 ) ;
#8587=CARTESIAN_POINT ( 'NONE',  ( 14.39714448835432670, 13.90806243540158071, 5.951255046771932733 ) ) ;
#8589=ORIENTED_EDGE ( 'NONE', *, *, #24863, .F. ) ;
#8595=CARTESIAN_POINT ( 'NONE',  ( 4.678038002344204749, 19.46363151887951659, 5.872146474157316831 ) ) ;
#8597=CARTESIAN_POINT ( 'NONE',  ( 6.139601762201234436, 19.03438667047814903, 18.84056766331482535 ) ) ;
#8601=CARTESIAN_POINT ( 'NONE',  ( 19.89797503522100541, 2.188012981718272076, 19.33715507985239412 ) ) ;
#8602=EDGE_LOOP ( 'NONE', ( #26174, #7630, #16944, #26807 ) ) ;
#8603=EDGE_CURVE ( 'NONE', #28210, #2701, #13058, .T. ) ;
#8604=AXIS2_PLACEMENT_3D ( 'NONE', #14146, #21631, #30673 ) ;
#8606=CARTESIAN_POINT ( 'NONE',  ( 18.12620810650619418, -8.494884113463655240, 7.500898271101006820 ) ) ;
#8607=CARTESIAN_POINT ( 'NONE',  ( -13.78503626495109913, 10.05991541429405167, 5.872146474157316831 ) ) ;
#8608=CARTESIAN_POINT ( 'NONE',  ( 3.835725748988828787, 16.61467071301743559, 20.32367522806703874 ) ) ;
#8609=ORIENTED_EDGE ( 'NONE', *, *, #27567, .F. ) ;
#8611=CARTESIAN_POINT ( 'NONE',  ( 12.93167884982522153, 11.07185515092108297, 6.143977687428010981 ) ) ;
#8613=EDGE_CURVE ( 'NONE', #18506, #7773, #10554, .T. ) ;
#8614=DIRECTION ( 'NONE',  ( -0.000000000000000000, -0.000000000000000000, 1.000000000000000000 ) ) ;
#8617=ORIENTED_EDGE ( 'NONE', *, *, #20863, .T. ) ;
#8619=DIRECTION ( 'NONE',  ( -0.000000000000000000, -0.000000000000000000, 1.000000000000000000 ) ) ;
#8620=CARTESIAN_POINT ( 'NONE',  ( 1.000000000000008438, 17.23749217771910480, 1.500000000000000000 ) ) ;
#8621=ORIENTED_EDGE ( 'NONE', *, *, #12266, .T. ) ;
#8626=DIRECTION ( 'NONE',  ( 1.000000000000000000, 0.000000000000000000, 0.000000000000000000 ) ) ;
#8628=CARTESIAN_POINT ( 'NONE',  ( 0.08889351957746359501, -20.00017437841852441, 7.626647697317581631 ) ) ;
#8638=CARTESIAN_POINT ( 'NONE',  ( 0.5710336623368666986, -20.00960304012540547, 7.627891251804737927 ) ) ;
#8640=ORIENTED_EDGE ( 'NONE', *, *, #18628, .T. ) ;
#8645=CARTESIAN_POINT ( 'NONE',  ( -6.044935790874364834, 19.08338196164711320, 7.652108011868850035 ) ) ;
#8647=CARTESIAN_POINT ( 'NONE',  ( 10.04466414020357057, -13.77914355952372638, 7.627891251804737927 ) ) ;
#8648=EDGE_CURVE ( 'NONE', #29085, #18738, #11516, .T. ) ;
#8650=B_SPLINE_CURVE_WITH_KNOTS ( 'NONE', 3,
 ( #17101, #22690, #8532, #25191, #30037, #17887, #3836, #3536, #27551, #27402, #17568, #13361, #1342, #22855, #1506, #10860 ),
 .UNSPECIFIED., .F., .F.,
 ( 4, 2, 2, 2, 2, 2, 2, 4 ),
 ( 0.5000000000000000000, 0.6250000000000002220, 0.6875000000000004441, 0.7187500000000005551, 0.7500000000000006661, 0.8125000000000004441, 0.8750000000000002220, 1.000000000000000000 ),
 .UNSPECIFIED. ) ;
#8657=CARTESIAN_POINT ( 'NONE',  ( -5.976020107417634009, 19.08630880174946043, 5.652196082369965069 ) ) ;
#8659=CARTESIAN_POINT ( 'NONE',  ( 3.537840656620562019, 16.69140805417697138, 5.759928666072750225 ) ) ;
#8663=VECTOR ( 'NONE', #14482, 1000.000000000000000 ) ;
#8664=CARTESIAN_POINT ( 'NONE',  ( 2.878478920843542177, 0.8451976705242683074, 24.50000000000000000 ) ) ;
#8666=ORIENTED_EDGE ( 'NONE', *, *, #14717, .F. ) ;
#8669=EDGE_CURVE ( 'NONE', #23120, #24284, #7136, .T. ) ;
#8671=EDGE_CURVE ( 'NONE', #20089, #7538, #108, .T. ) ;
#8672=CARTESIAN_POINT ( 'NONE',  ( 4.622016212553096359, -12.19167610014704906, 24.50000000000000000 ) ) ;
#8674=DIRECTION ( 'NONE',  ( 0.000000000000000000, 0.000000000000000000, 1.000000000000000000 ) ) ;
#8676=CARTESIAN_POINT ( 'NONE',  ( 1.239979252855711866, -19.96159058730291136, 18.84486140012300126 ) ) ;
#8680=DIRECTION ( 'NONE',  ( -0.000000000000000000, -0.000000000000000000, 1.000000000000000000 ) ) ;
#8689=DIRECTION ( 'NONE',  ( 0.6548607339452889864, 0.7557495743542548272, 0.000000000000000000 ) ) ;
#8690=ORIENTED_EDGE ( 'NONE', *, *, #8004, .F. ) ;
#8692=DIRECTION ( 'NONE',  ( 0.000000000000000000, 0.000000000000000000, 1.000000000000000000 ) ) ;
#8693=EDGE_CURVE ( 'NONE', #13794, #624, #2286, .T. ) ;
#8694=VERTEX_POINT ( 'NONE', #28654 ) ;
#8695=ORIENTED_EDGE ( 'NONE', *, *, #11159, .T. ) ;
#8696=CARTESIAN_POINT ( 'NONE',  ( -15.71962203721309592, -1.249857212218242974, 1.500000000000001332 ) ) ;
#8698=CARTESIAN_POINT ( 'NONE',  ( -8.546421330728131593, -14.74799399454104076, 18.34798005862930381 ) ) ;
#8700=EDGE_LOOP ( 'NONE', ( #28361, #11221, #16200, #23914 ) ) ;
#8702=VERTEX_POINT ( 'NONE', #7284 ) ;
#8705=VERTEX_POINT ( 'NONE', #16342 ) ;
#8709=CARTESIAN_POINT ( 'NONE',  ( 16.71904594334104388, 3.341332093703274442, 7.643931100913408550 ) ) ;
#8710=CARTESIAN_POINT ( 'NONE',  ( -8.266165397079788590, -14.91833037834293307, 20.29915277494337644 ) ) ;
#8713=DIRECTION ( 'NONE',  ( -0.000000000000000000, -0.000000000000000000, -1.000000000000000000 ) ) ;
#8715=CARTESIAN_POINT ( 'NONE',  ( 11.77505735701808121, -16.18809529858903673, 18.73743063545763121 ) ) ;
#8718=ORIENTED_EDGE ( 'NONE', *, *, #5583, .F. ) ;
#8722=ORIENTED_EDGE ( 'NONE', *, *, #26877, .F. ) ;
#8723=CYLINDRICAL_SURFACE ( 'NONE', #5677, 20.00000000000000000 ) ;
#8724=DIRECTION ( 'NONE',  ( 0.000000000000000000, 0.000000000000000000, 1.000000000000000000 ) ) ;
#8725=CIRCLE ( 'NONE', #12716, 0.7499999999999997780 ) ;
#8735=CARTESIAN_POINT ( 'NONE',  ( -5.130938270761554065, 7.974144905643839820, 13.00000000000000178 ) ) ;
#8741=FACE_OUTER_BOUND ( 'NONE', #5416, .T. ) ;
#8743=CARTESIAN_POINT ( 'NONE',  ( -16.93532286002824350, 1.879651667671730531, 20.32842677360128292 ) ) ;
#8744=CARTESIAN_POINT ( 'NONE',  ( 15.55167013926946673, -6.938753487154071919, 5.862424720655265098 ) ) ;
#8745=CARTESIAN_POINT ( 'NONE',  ( -13.52555592105307980, 10.38406032642568277, 5.678370764302467677 ) ) ;
#8746=CARTESIAN_POINT ( 'NONE',  ( 4.330755352941443093, 19.54356050811956180, 19.14333282897057842 ) ) ;
#8747=VERTEX_POINT ( 'NONE', #21625 ) ;
#8748=ORIENTED_EDGE ( 'NONE', *, *, #7912, .T. ) ;
#8750=CARTESIAN_POINT ( 'NONE',  ( 10.08428597738326893, -13.75408489947211521, 5.653604225791663218 ) ) ;
#8752=CARTESIAN_POINT ( 'NONE',  ( -5.055631408663415094, 19.36903233965648141, 19.00652017443069752 ) ) ;
#8753=DIRECTION ( 'NONE',  ( 0.000000000000000000, -0.000000000000000000, -1.000000000000000000 ) ) ;
#8757=CARTESIAN_POINT ( 'NONE',  ( -19.92072812706008023, 1.967956072006117996, 7.500147780736496017 ) ) ;
#8759=CARTESIAN_POINT ( 'NONE',  ( 19.83258132550258424, 2.584089194578470750, 18.54479204710284179 ) ) ;
#8760=EDGE_LOOP ( 'NONE', ( #5225, #26507, #22110, #10840 ) ) ;
#8764=CARTESIAN_POINT ( 'NONE',  ( -19.84344116185557283, 2.497567387674354489, 7.652108011868850035 ) ) ;
#8765=EDGE_CURVE ( 'NONE', #14232, #21410, #16028, .T. ) ;
#8767=CARTESIAN_POINT ( 'NONE',  ( -19.91153203745398770, 1.881428233485403556, 20.15039051365863543 ) ) ;
#8774=VECTOR ( 'NONE', #7950, 1000.000000000000000 ) ;
#8775=EDGE_CURVE ( 'NONE', #1242, #28669, #17778, .T. ) ;
#8778=ORIENTED_EDGE ( 'NONE', *, *, #12803, .F. ) ;
#8781=CARTESIAN_POINT ( 'NONE',  ( -4.699300155672233359, 16.36248368692520927, 6.143977687428009204 ) ) ;
#8782=AXIS2_PLACEMENT_3D ( 'NONE', #19992, #27172, #5800 ) ;
#8788=ORIENTED_EDGE ( 'NONE', *, *, #16599, .F. ) ;
#8790=CARTESIAN_POINT ( 'NONE',  ( -0.4553004113513210993, -19.99503986737292038, 19.96302680909624527 ) ) ;
#8796=DIRECTION ( 'NONE',  ( 1.000000000000000000, 0.000000000000000000, 0.000000000000000000 ) ) ;
#8798=CARTESIAN_POINT ( 'NONE',  ( 3.264443111031099409, 16.75603743214636765, 7.269896094239229889 ) ) ;
#8799=ORIENTED_EDGE ( 'NONE', *, *, #7282, .T. ) ;
#8812=CIRCLE ( 'NONE', #29716, 0.7500000000000006661 ) ;
#8815=ADVANCED_FACE ( 'NONE', ( #1959 ), #8418, .F. ) ;
#8819=CARTESIAN_POINT ( 'NONE',  ( 16.59744209610425614, 3.993643014774751698, 6.037360021877315575 ) ) ;
#8824=CARTESIAN_POINT ( 'NONE',  ( 18.33599632111990729, -7.986941774664182425, 20.34789198813115263 ) ) ;
#8828=CARTESIAN_POINT ( 'NONE',  ( 9.248129367672065726, 2.094186647214772989, 21.50000000000000000 ) ) ;
#8830=CARTESIAN_POINT ( 'NONE',  ( -9.225205623866960636, -14.30976465319822211, 18.72771030977187223 ) ) ;
#8832=VERTEX_POINT ( 'NONE', #13094 ) ;
#8833=VECTOR ( 'NONE', #22076, 1000.000000000000000 ) ;
#8836=EDGE_CURVE ( 'NONE', #18738, #13283, #22587, .T. ) ;
#8837=CARTESIAN_POINT ( 'NONE',  ( -11.86767874445213167, -1.850092897552710225, 1.500000000000001332 ) ) ;
#8838=EDGE_CURVE ( 'NONE', #1929, #13391, #10299, .T. ) ;
#8843=EDGE_CURVE ( 'NONE', #14509, #6239, #4377, .T. ) ;
#8844=CARTESIAN_POINT ( 'NONE',  ( 9.439370189418763601, -14.17768557490412640, 18.47056384035244037 ) ) ;
#8847=CARTESIAN_POINT ( 'NONE',  ( -19.71077436674131178, 3.493128416889931032, 6.530762810602277924 ) ) ;
#8848=EDGE_CURVE ( 'NONE', #13827, #7538, #3827, .T. ) ;
#8850=VECTOR ( 'NONE', #9126, 1000.000000000000000 ) ;
#8852=FACE_OUTER_BOUND ( 'NONE', #25630, .T. ) ;
#8859=DIRECTION ( 'NONE',  ( 1.000000000000000000, 0.000000000000000000, 0.000000000000000000 ) ) ;
#8860=AXIS2_PLACEMENT_3D ( 'NONE', #7977, #19971, #22452 ) ;
#8874=EDGE_CURVE ( 'NONE', #22820, #1637, #27749, .T. ) ;
#8875=AXIS2_PLACEMENT_3D ( 'NONE', #2334, #26362, #23688 ) ;
#8877=CARTESIAN_POINT ( 'NONE',  ( 10.14446381905444561, -13.71082019663804452, 18.39992786714538298 ) ) ;
#8879=AXIS2_PLACEMENT_3D ( 'NONE', #21933, #562, #19595 ) ;
#8881=ORIENTED_EDGE ( 'NONE', *, *, #22169, .F. ) ;
#8882=CARTESIAN_POINT ( 'NONE',  ( -5.549074438707202184, 16.11683645443577717, 5.652196082367002106 ) ) ;
#8883=EDGE_LOOP ( 'NONE', ( #11950, #11373 ) ) ;
#8884=CARTESIAN_POINT ( 'NONE',  ( 11.77411685406914188, -16.16721897189997037, 18.73377938172349033 ) ) ;
#8886=CARTESIAN_POINT ( 'NONE',  ( -13.04869608158528393, 10.94699654828723645, 7.526951045817045660 ) ) ;
#8894=ORIENTED_EDGE ( 'NONE', *, *, #19817, .T. ) ;
#8897=VECTOR ( 'NONE', #1503, 1000.000000000000000 ) ;
#8899=AXIS2_PLACEMENT_3D ( 'NONE', #27164, #27014, #22162 ) ;
#8902=CARTESIAN_POINT ( 'NONE',  ( -17.59389297287863485, -9.510918850537244396, 6.392525840300348428 ) ) ;
#8907=CARTESIAN_POINT ( 'NONE',  ( 16.77888236039447278, 2.967719242317201633, 20.32842677360128292 ) ) ;
#8908=VERTEX_POINT ( 'NONE', #9735 ) ;
#8909=CARTESIAN_POINT ( 'NONE',  ( -19.81587719261256453, 2.836291464538557516, 20.29090034784956131 ) ) ;
#8910=CARTESIAN_POINT ( 'NONE',  ( 15.45190528822776344, -7.145941350103559131, 7.176035686813569292 ) ) ;
#8912=CARTESIAN_POINT ( 'NONE',  ( -14.01100295375882965, 9.765235586930179679, 6.672349528511551497 ) ) ;
#8913=CARTESIAN_POINT ( 'NONE',  ( 3.424309912165880210, 16.71834993634869448, 18.56793045041961321 ) ) ;
#8915=ORIENTED_EDGE ( 'NONE', *, *, #12643, .F. ) ;
#8919=CARTESIAN_POINT ( 'NONE',  ( 15.53710936759973116, 12.59357901975564076, 19.21471108562413832 ) ) ;
#8920=B_SPLINE_SURFACE_WITH_KNOTS ( 'NONE', 3, 1, ( 
 ( #5982, #8496 ),
 ( #27358, #22649 ),
 ( #17999, #13481 ),
 ( #22962, #24459 ),
 ( #17129, #2207 ),
 ( #23561, #7622 ),
 ( #14639, #28420 ),
 ( #19620, #19474 ),
 ( #28988, #24141 ),
 ( #29142, #17287 ),
 ( #7777, #4549 ),
 ( #14789, #16552 ),
 ( #9233, #23417 ),
 ( #18748, #7043 ),
 ( #3102, #26820 ),
 ( #26651, #24306 ),
 ( #2789, #12308 ),
 ( #21810, #452 ),
 ( #2053, #2956 ),
 ( #12474, #25770 ),
 ( #28265, #5282 ),
 ( #21964, #4400 ),
 ( #18604, #592 ),
 ( #5445, #14948 ),
 ( #9970, #10110 ),
 ( #11576, #11725 ),
 ( #12621, #30446 ),
 ( #6891, #21216 ),
 ( #9087, #28115 ),
 ( #6737, #16248 ),
 ( #21070, #30592 ) ),
 .UNSPECIFIED., .F., .F., .F.,
 ( 4, 3, 3, 3, 3, 3, 3, 3, 3, 3, 4 ),
 ( 2, 2 ),
 ( 0.4999999998345686092, 0.5360336730431939367, 0.5907651151589012883, 0.6456034593241830599, 0.6998270958050434309, 0.7529536536315937223, 0.8052385063053260073, 0.8575343587103997356, 0.9106564858195042023, 0.9648414833209685293, 1.000000006602610236 ),
 ( 0.000000000000000000, 1.000000000000000000 ),
 .UNSPECIFIED. ) ;
#8921=CARTESIAN_POINT ( 'NONE',  ( -4.721574378597740207, 16.35655934831870084, 18.80699882434806369 ) ) ;
#8922=CYLINDRICAL_SURFACE ( 'NONE', #22723, 9.482273699623480212 ) ;
#8928=EDGE_LOOP ( 'NONE', ( #14893, #24086, #11584, #18136 ) ) ;
#8929=CARTESIAN_POINT ( 'NONE',  ( -17.06646200723453433, 0.6378183210065198061, 6.560937769032974209 ) ) ;
#8931=DIRECTION ( 'NONE',  ( 0.000000000000000000, 0.000000000000000000, 1.000000000000000000 ) ) ;
#8943=LINE ( 'NONE', #29997, #14342 ) ;
#8946=CARTESIAN_POINT ( 'NONE',  ( -12.24063095261064227, 4.490763173670005770, 24.50000000000000000 ) ) ;
#8947=CARTESIAN_POINT ( 'NONE',  ( 1.792916928892099859, -16.98383425522535006, 6.782048567692550378 ) ) ;
#8952=ORIENTED_EDGE ( 'NONE', *, *, #5385, .T. ) ;
#8958=ORIENTED_EDGE ( 'NONE', *, *, #23694, .F. ) ;
#8959=CARTESIAN_POINT ( 'NONE',  ( -0.1550506074450101746, -19.99977091204052115, 20.22277707861862339 ) ) ;
#8962=DIRECTION ( 'NONE',  ( 0.000000000000000000, 0.000000000000000000, -1.000000000000000000 ) ) ;
#8964=FACE_BOUND ( 'NONE', #669, .T. ) ;
#8970=ORIENTED_EDGE ( 'NONE', *, *, #21099, .T. ) ;
#8971=DIRECTION ( 'NONE',  ( 1.000000000000000000, 0.000000000000000000, 0.000000000000000000 ) ) ;
#8975=CARTESIAN_POINT ( 'NONE',  ( 12.17894461864673517, 11.93905285490450119, 18.34938820207544907 ) ) ;
#8976=CARTESIAN_POINT ( 'NONE',  ( 16.74250988114178185, 3.198928528055117848, 5.652196082368483587 ) ) ;
#8981=EDGE_CURVE ( 'NONE', #16618, #7784, #7323, .T. ) ;
#8989=CARTESIAN_POINT ( 'NONE',  ( -18.46427634282259334, -7.732205987805708780, 19.56050940960062690 ) ) ;
#8992=ORIENTED_EDGE ( 'NONE', *, *, #24601, .T. ) ;
#8994=DIRECTION ( 'NONE',  ( 0.000000000000000000, 0.000000000000000000, -1.000000000000000000 ) ) ;
#8996=ADVANCED_FACE ( 'NONE', ( #27054 ), #17871, .T. ) ;
#8998=ORIENTED_EDGE ( 'NONE', *, *, #5777, .F. ) ;
#9000=CARTESIAN_POINT ( 'NONE',  ( 15.40685886292496676, -7.237730981567044530, 19.66989035740801839 ) ) ;
#9004=VERTEX_POINT ( 'NONE', #20488 ) ;
#9005=DIRECTION ( 'NONE',  ( 1.000000000000000000, 0.000000000000000000, 0.000000000000000000 ) ) ;
#9006=CARTESIAN_POINT ( 'NONE',  ( 15.28716501070585387, 12.89617714416415239, 5.849008070840543638 ) ) ;
#9007=CARTESIAN_POINT ( 'NONE',  ( 0.000000000000000000, 0.000000000000000000, 21.50000000000000000 ) ) ;
#9011=AXIS2_PLACEMENT_3D ( 'NONE', #9007, #16018, #30059 ) ;
#9019=CARTESIAN_POINT ( 'NONE',  ( -0.5696721008582752432, -20.00987732873323566, 7.080843742048788414 ) ) ;
#9020=ADVANCED_FACE ( 'NONE', ( #6749 ), #18389, .T. ) ;
#9021=EDGE_CURVE ( 'NONE', #18086, #1853, #28431, .T. ) ;
#9023=CARTESIAN_POINT ( 'NONE',  ( -17.06430796155045115, 0.6673913134545759185, 19.61324152429826739 ) ) ;
#9025=VERTEX_POINT ( 'NONE', #12050 ) ;
#9027=DIRECTION ( 'NONE',  ( 0.9594929736144974797, 0.2817325568414297265, 0.000000000000000000 ) ) ;
#9029=ORIENTED_EDGE ( 'NONE', *, *, #9021, .T. ) ;
#9032=DIRECTION ( 'NONE',  ( 0.000000000000000000, 0.000000000000000000, 1.000000000000000000 ) ) ;
#9038=LINE ( 'NONE', #1855, #5447 ) ;
#9049=CARTESIAN_POINT ( 'NONE',  ( -17.58178100985202619, -9.533151461302367125, 6.788986777570709563 ) ) ;
#9050=AXIS2_PLACEMENT_3D ( 'NONE', #23555, #2201, #30738 ) ;
#9053=CARTESIAN_POINT ( 'NONE',  ( 19.77267785325472005, 3.123260753354262231, 18.34969686940296185 ) ) ;
#9054=ORIENTED_EDGE ( 'NONE', *, *, #28685, .T. ) ;
#9055=CARTESIAN_POINT ( 'NONE',  ( -19.78525473782456956, 3.044038662852082133, 20.19668224736330941 ) ) ;
#9057=CARTESIAN_POINT ( 'NONE',  ( -15.84987138805249707, 12.22653209092614901, 7.280727868105637768 ) ) ;
#9058=CARTESIAN_POINT ( 'NONE',  ( 4.866781629985560187, 19.41732998781225916, 18.44527579819791185 ) ) ;
#9060=VERTEX_POINT ( 'NONE', #19376 ) ;
#9062=CARTESIAN_POINT ( 'NONE',  ( 10.58819075804203891, -13.39403179698335045, 6.147510495896841398 ) ) ;
#9064=CARTESIAN_POINT ( 'NONE',  ( 15.40745978470623356, 12.75221478727799784, 18.72886616302734453 ) ) ;
#9065=CARTESIAN_POINT ( 'NONE',  ( -5.869193111140220687, 19.13804834536702160, 18.35377592296120497 ) ) ;
#9070=EDGE_LOOP ( 'NONE', ( #26684, #11491 ) ) ;
#9072=CARTESIAN_POINT ( 'NONE',  ( 1.340340228783115428, -19.95510490826381655, 6.919864475265769421 ) ) ;
#9073=DIRECTION ( 'NONE',  ( -0.5406408174555974444, -0.8412535328311813165, -0.000000000000000000 ) ) ;
#9074=CARTESIAN_POINT ( 'NONE',  ( 19.85594780280176153, 2.397944088302077503, 18.72886616302735519 ) ) ;
#9077=VERTEX_POINT ( 'NONE', #19209 ) ;
#9078=EDGE_CURVE ( 'NONE', #18371, #28054, #28737, .T. ) ;
#9079=CARTESIAN_POINT ( 'NONE',  ( 15.84452017418782432, -6.290821626254208709, 5.652605728828373977 ) ) ;
#9080=FACE_OUTER_BOUND ( 'NONE', #2681, .T. ) ;
#9084=B_SPLINE_CURVE_WITH_KNOTS ( 'NONE', 3,
 ( #4792, #2151, #28367, #6990, #21634, #9485, #7147, #9174, #16658, #2465, #11983, #11527, #21475, #117, #9637, #13863, #14466, #6826 ),
 .UNSPECIFIED., .F., .F.,
 ( 4, 2, 2, 2, 2, 2, 2, 2, 4 ),
 ( 0.000000000000000000, 0.0003967869494442882641, 0.0007935738988885765281, 0.001190360848332864792, 0.001587147797777153056, 0.001983934747221441537, 0.002380721696665729584, 0.002777508646110017632, 0.003174295595554306113 ),
 .UNSPECIFIED. ) ;
#9086=DIRECTION ( 'NONE',  ( 0.000000000000000000, 1.000000000000000000, 0.000000000000000000 ) ) ;
#9087=CARTESIAN_POINT ( 'NONE',  ( -6.116198564155506112, 19.06064343544020190, 20.33971507717571114 ) ) ;
#9088=DIRECTION ( 'NONE',  ( 0.9594929736144992560, 0.2817325568414232317, 0.000000000000000000 ) ) ;
#9089=CARTESIAN_POINT ( 'NONE',  ( -16.93068695965898840, 1.913742347956913115, 7.626437579292364433 ) ) ;
#9091=DIRECTION ( 'NONE',  ( 0.000000000000000000, 0.000000000000000000, 1.000000000000000000 ) ) ;
#9093=ORIENTED_EDGE ( 'NONE', *, *, #5765, .T. ) ;
#9095=CARTESIAN_POINT ( 'NONE',  ( 9.922755320353061848, -13.86203410616582232, 7.652108011868850035 ) ) ;
#9096=DIRECTION ( 'NONE',  ( 1.000000000000000000, 0.000000000000000000, 0.000000000000000000 ) ) ;
#9099=CARTESIAN_POINT ( 'NONE',  ( 0.08889351957746016719, -20.00017437841852441, 20.32243167357988511 ) ) ;
#9101=AXIS2_PLACEMENT_3D ( 'NONE', #7363, #11574, #28723 ) ;
#9105=CIRCLE ( 'NONE', #13102, 0.7500000000000011102 ) ;
#9107=CARTESIAN_POINT ( 'NONE',  ( 6.437683520590175235, -6.962021646281549181, 21.50000000000000000 ) ) ;
#9119=CARTESIAN_POINT ( 'NONE',  ( 12.76326067947990772, 11.27442216569340161, 18.54473042795395088 ) ) ;
#9123=CIRCLE ( 'NONE', #14602, 0.7500000000000006661 ) ;
#9124=CARTESIAN_POINT ( 'NONE',  ( -9.248129367672078160, -2.094186647214714814, 21.50000000000000000 ) ) ;
#9125=LINE ( 'NONE', #18645, #22749 ) ;
#9126=DIRECTION ( 'NONE',  ( -0.000000000000000000, -0.000000000000000000, 1.000000000000000000 ) ) ;
#9128=CARTESIAN_POINT ( 'NONE',  ( 3.113107691796848542, 16.79024107225415463, 19.02573955821369722 ) ) ;
#9133=ORIENTED_EDGE ( 'NONE', *, *, #26906, .T. ) ;
#9140=CARTESIAN_POINT ( 'NONE',  ( -6.507434545313869556, 15.78991698230835716, 19.47952243369111258 ) ) ;
#9142=EDGE_CURVE ( 'NONE', #2810, #8702, #21233, .T. ) ;
#9146=CARTESIAN_POINT ( 'NONE',  ( -19.80175191879421348, 2.933369436805203900, 5.749228751562096562 ) ) ;
#9152=EDGE_LOOP ( 'NONE', ( #8970, #16522 ) ) ;
#9156=CARTESIAN_POINT ( 'NONE',  ( -14.76380438154529173, 13.49194818783279537, 6.144783687052509435 ) ) ;
#9158=CARTESIAN_POINT ( 'NONE',  ( 16.87575838019316876, 2.225846228041723940, 19.60617949693493500 ) ) ;
#9159=DIRECTION ( 'NONE',  ( 0.9898214418809327952, -0.1423148382732850048, 0.000000000000000000 ) ) ;
#9161=CARTESIAN_POINT ( 'NONE',  ( 16.70665413472817562, 3.412884783584984927, 7.627891251804737927 ) ) ;
#9166=CARTESIAN_POINT ( 'NONE',  ( 8.884323311075775109, 1.438332125858202692, 1.500000000000001332 ) ) ;
#9168=ORIENTED_EDGE ( 'NONE', *, *, #13955, .T. ) ;
#9169=CIRCLE ( 'NONE', #28025, 0.7499999999999997780 ) ;
#9170=CARTESIAN_POINT ( 'NONE',  ( -6.315055774899184904, 15.86014940733236678, 6.037360021877316463 ) ) ;
#9174=CARTESIAN_POINT ( 'NONE',  ( 4.333676792162787450, 19.52490442444424801, 19.08830981656264214 ) ) ;
#9181=EDGE_CURVE ( 'NONE', #4023, #20845, #15779, .T. ) ;
#9182=CARTESIAN_POINT ( 'NONE',  ( -15.66719571743413120, 12.43196305300236659, 18.47531940416306284 ) ) ;
#9187=ORIENTED_EDGE ( 'NONE', *, *, #14304, .F. ) ;
#9190=ORIENTED_EDGE ( 'NONE', *, *, #414, .F. ) ;
#9192=EDGE_CURVE ( 'NONE', #2008, #30491, #15768, .T. ) ;
#9195=CARTESIAN_POINT ( 'NONE',  ( -17.98413878735053117, -8.751483025296225904, 5.652912763329821288 ) ) ;
#9199=CARTESIAN_POINT ( 'NONE',  ( 16.84421249428843126, 2.491431357970652183, 18.63641924841378028 ) ) ;
#9201=CARTESIAN_POINT ( 'NONE',  ( 15.79886199502269761, -6.395730384537285040, 5.651989602109219746 ) ) ;
#9202=CARTESIAN_POINT ( 'NONE',  ( -13.38159811071079552, 10.55828946507379307, 5.652196082364323360 ) ) ;
#9203=LINE ( 'NONE', #28227, #4823 ) ;
#9205=ORIENTED_EDGE ( 'NONE', *, *, #20023, .F. ) ;
#9209=CARTESIAN_POINT ( 'NONE',  ( 15.28831480992544201, 12.89481865072259303, 20.14992337338001960 ) ) ;
#9214=DIRECTION ( 'NONE',  ( 1.000000000000000000, 0.000000000000000000, 0.000000000000000000 ) ) ;
#9215=VERTEX_POINT ( 'NONE', #27793 ) ;
#9217=CARTESIAN_POINT ( 'NONE',  ( -19.93005420669540584, 1.873390432278239315, 7.441806358946449151 ) ) ;
#9220=CARTESIAN_POINT ( 'NONE',  ( 19.86476987328768118, 2.322391784566624207, 18.84056766331482180 ) ) ;
#9221=EDGE_LOOP ( 'NONE', ( #20868, #29223, #1693, #10615 ) ) ;
#9224=CARTESIAN_POINT ( 'NONE',  ( 18.68320837179354044, -7.186693706611501753, 6.131018562779544823 ) ) ;
#9233=CARTESIAN_POINT ( 'NONE',  ( -6.889674169070711507, 18.79461648230378401, 19.03762469184452755 ) ) ;
#9235=DIRECTION ( 'NONE',  ( -0.000000000000000000, -0.000000000000000000, 1.000000000000000000 ) ) ;
#9241=EDGE_LOOP ( 'NONE', ( #21328, #9561, #13650, #21153 ) ) ;
#9244=CARTESIAN_POINT ( 'NONE',  ( -20.00000000000004263, 1.387778780781445676E-14, 1.500000000000000000 ) ) ;
#9248=LINE ( 'NONE', #14390, #20080 ) ;
#9250=DIRECTION ( 'NONE',  ( -0.000000000000000000, -0.000000000000000000, -1.000000000000000000 ) ) ;
#9254=DIRECTION ( 'NONE',  ( -0.000000000000000000, -0.000000000000000000, 1.000000000000000000 ) ) ;
#9257=CARTESIAN_POINT ( 'NONE',  ( -13.71336669122886853, 10.15199454957378578, 5.759928666072749337 ) ) ;
#9259=LINE ( 'NONE', #18627, #6471 ) ;
#9261=ORIENTED_EDGE ( 'NONE', *, *, #12043, .F. ) ;
#9265=CARTESIAN_POINT ( 'NONE',  ( -0.08542884365699984772, -20.01766063302414622, 18.44501272782439827 ) ) ;
#9266=CARTESIAN_POINT ( 'NONE',  ( -7.692543755867215616, -15.24678548464671479, 6.892848776733236704 ) ) ;
#9268=CARTESIAN_POINT ( 'NONE',  ( 1.082887659287351312, -19.98847979319446821, 18.64703902303423178 ) ) ;
#9271=CARTESIAN_POINT ( 'NONE',  ( 16.56213591300094379, 4.162091996070008904, 6.392658652357122939 ) ) ;
#9273=CARTESIAN_POINT ( 'NONE',  ( -2.662523238938575343, -12.47340865698848056, 24.50000000000000000 ) ) ;
#9275=CIRCLE ( 'NONE', #15754, 0.7500000000000006661 ) ;
#9276=CARTESIAN_POINT ( 'NONE',  ( -15.22000698778095540, -7.667275871987174973, 18.34727598691068096 ) ) ;
#9277=DIRECTION ( 'NONE',  ( 0.9096319953545183301, 0.4154150130018864906, 0.000000000000000000 ) ) ;
#9282=CARTESIAN_POINT ( 'NONE',  ( -11.40980092660686829, 6.310027164379044429, 24.50000000000000000 ) ) ;
#9290=EDGE_LOOP ( 'NONE', ( #22075, #18250, #20237, #22957 ) ) ;
#9291=CARTESIAN_POINT ( 'NONE',  ( 18.01689225005682005, -8.724154469992756233, 19.96783386855779341 ) ) ;
#9292=CARTESIAN_POINT ( 'NONE',  ( 4.994189150946234612, 16.27260345083324822, 6.864725433338323413 ) ) ;
#9295=CIRCLE ( 'NONE', #12289, 0.7500000000000006661 ) ;
#9296=CARTESIAN_POINT ( 'NONE',  ( 12.25849595087226973, 11.84990609407551077, 7.643931100913408550 ) ) ;
#9300=ORIENTED_EDGE ( 'NONE', *, *, #16599, .T. ) ;
#9304=AXIS2_PLACEMENT_3D ( 'NONE', #5990, #22367, #10362 ) ;
#9305=ORIENTED_EDGE ( 'NONE', *, *, #2427, .T. ) ;
#9308=CARTESIAN_POINT ( 'NONE',  ( 16.76361099856289982, 3.068725842123817493, 18.34727598691067740 ) ) ;
#9311=CARTESIAN_POINT ( 'NONE',  ( 19.76130184095197606, 3.194145055459935101, 7.652108011868850035 ) ) ;
#9316=CARTESIAN_POINT ( 'NONE',  ( -6.187077094091591789, 11.47693674426096955, 1.500000000000001332 ) ) ;
#9320=CARTESIAN_POINT ( 'NONE',  ( 10.56600709331201315, -13.41035981659391751, 19.89182036555910571 ) ) ;
#9321=B_SPLINE_CURVE_WITH_KNOTS ( 'NONE', 3,
 ( #11723, #21214, #30744, #26218, #14203, #23712, #16869, #2362, #11889, #21384, #19051, #28567, #14372, #23880, #2523, #12038 ),
 .UNSPECIFIED., .F., .F.,
 ( 4, 2, 2, 2, 2, 2, 2, 4 ),
 ( 0.4999999999999997224, 0.6250000000000018874, 0.6875000000000026645, 0.7187500000000028866, 0.7500000000000031086, 0.8125000000000019984, 0.8750000000000006661, 1.000000000000000000 ),
 .UNSPECIFIED. ) ;
#9323=DIRECTION ( 'NONE',  ( -1.000000000000000000, 0.000000000000000000, 0.000000000000000000 ) ) ;
#9326=CARTESIAN_POINT ( 'NONE',  ( -15.85201432996392867, 12.19518096057846179, 6.037995405461184184 ) ) ;
#9329=ORIENTED_EDGE ( 'NONE', *, *, #26648, .F. ) ;
#9330=AXIS2_PLACEMENT_3D ( 'NONE', #19667, #29189, #17338 ) ;
#9337=ORIENTED_EDGE ( 'NONE', *, *, #18628, .F. ) ;
#9338=AXIS2_PLACEMENT_3D ( 'NONE', #26140, #29104, #4937 ) ;
#9343=ORIENTED_EDGE ( 'NONE', *, *, #20455, .F. ) ;
#9344=VECTOR ( 'NONE', #16477, 1000.000000000000114 ) ;
#9346=B_SPLINE_CURVE_WITH_KNOTS ( 'NONE', 3,
 ( #2097, #4594, #11620, #27699, #3993, #23000, #6325, #20819, #30341, #21111, #14096, #13961, #4284, #4139, #30631, #15840, #25820, #13813, #9276, #25516 ),
 .UNSPECIFIED., .F., .F.,
 ( 4, 2, 2, 2, 2, 2, 2, 2, 2, 4 ),
 ( 0.000000000000000000, 0.06250000000000184575, 0.1250000000000036915, 0.1875000000000055511, 0.2187500000000056621, 0.2500000000000057732, 0.3125000000000043299, 0.3750000000000028866, 0.4375000000000013878, 0.4999999999999999445 ),
 .UNSPECIFIED. ) ;
#9351=DIRECTION ( 'NONE',  ( 0.000000000000000000, 0.000000000000000000, 1.000000000000000000 ) ) ;
#9352=LINE ( 'NONE', #23386, #12888 ) ;
#9354=ORIENTED_EDGE ( 'NONE', *, *, #23258, .F. ) ;
#9355=CARTESIAN_POINT ( 'NONE',  ( -19.74686063004096326, 3.283826233409515183, 18.71435384576123440 ) ) ;
#9358=DIRECTION ( 'NONE',  ( 0.000000000000000000, 0.000000000000000000, 1.000000000000000000 ) ) ;
#9359=CARTESIAN_POINT ( 'NONE',  ( 0.000000000000000000, 0.000000000000000000, 1.500000000000001332 ) ) ;
#9366=CARTESIAN_POINT ( 'NONE',  ( -5.512483845762027102, 16.12829592175436133, 18.34777357837151968 ) ) ;
#9369=CARTESIAN_POINT ( 'NONE',  ( -5.849168665050585858, 19.12602664087013693, 5.651480102388686255 ) ) ;
#9374=CARTESIAN_POINT ( 'NONE',  ( -19.95549607358725908, 1.576375212833063921, 6.233981582756856987 ) ) ;
#9376=AXIS2_PLACEMENT_3D ( 'NONE', #20102, #12940, #3415 ) ;
#9377=CARTESIAN_POINT ( 'NONE',  ( 14.18307372309187109, 14.10107868313152224, 19.21940439362673914 ) ) ;
#9379=ORIENTED_EDGE ( 'NONE', *, *, #29953, .T. ) ;
#9381=CARTESIAN_POINT ( 'NONE',  ( 8.480328572437745294, -4.608906612435629491, 1.500000000000001332 ) ) ;
#9382=ORIENTED_EDGE ( 'NONE', *, *, #13036, .F. ) ;
#9383=DIRECTION ( 'NONE',  ( 0.8412535328311813165, -0.5406408174555974444, 0.000000000000000000 ) ) ;
#9385=CARTESIAN_POINT ( 'NONE',  ( -4.102102735472399786, 8.549050687778207092, 1.500000000000001332 ) ) ;
#9398=CARTESIAN_POINT ( 'NONE',  ( 15.38611090871063070, -7.279566334535291894, 6.519181285484530797 ) ) ;
#9400=AXIS2_PLACEMENT_3D ( 'NONE', #7598, #7917, #12743 ) ;
#9402=CIRCLE ( 'NONE', #13405, 0.7499999999999997780 ) ;
#9404=EDGE_CURVE ( 'NONE', #4276, #3697, #23539, .T. ) ;
#9408=DIRECTION ( 'NONE',  ( 1.000000000000000000, 0.000000000000000000, 0.000000000000000000 ) ) ;
#9412=CIRCLE ( 'NONE', #5914, 20.00000000000000000 ) ;
#9414=CARTESIAN_POINT ( 'NONE',  ( 0.2207535014603100587, -19.99921160563567568, 20.34789198813115618 ) ) ;
#9417=EDGE_CURVE ( 'NONE', #13589, #12796, #147, .T. ) ;
#9420=CARTESIAN_POINT ( 'NONE',  ( -13.38160118231794549, 10.55829203257430038, 5.652196082368482699 ) ) ;
#9425=LINE ( 'NONE', #7701, #14244 ) ;
#9428=VERTEX_POINT ( 'NONE', #5614 ) ;
#9429=CARTESIAN_POINT ( 'NONE',  ( 0.2775250113394547857, -20.01590685155468563, 18.34969686940295830 ) ) ;
#9431=EDGE_CURVE ( 'NONE', #1292, #8044, #2343, .T. ) ;
#9432=CARTESIAN_POINT ( 'NONE',  ( 4.967306913969569138, 16.28142803849144826, 19.66962785902261146 ) ) ;
#9433=AXIS2_PLACEMENT_3D ( 'NONE', #18549, #25567, #28053 ) ;
#9434=CARTESIAN_POINT ( 'NONE',  ( 1.350727940147186334, -19.97202376558939818, 19.14333282897057842 ) ) ;
#9439=CARTESIAN_POINT ( 'NONE',  ( -6.812559277181930106, 5.881244434206302607, 21.50000000000000000 ) ) ;
#9443=CARTESIAN_POINT ( 'NONE',  ( -14.92167319134950887, -8.273715889511855437, 5.810767894563978686 ) ) ;
#9447=CARTESIAN_POINT ( 'NONE',  ( -18.10021843967229316, -8.508777197197408881, 20.34789198813115974 ) ) ;
#9448=CARTESIAN_POINT ( 'NONE',  ( -15.21426671708081457, -7.679208962302482178, 20.34789198813115263 ) ) ;
#9451=ORIENTED_EDGE ( 'NONE', *, *, #21750, .T. ) ;
#9455=CARTESIAN_POINT ( 'NONE',  ( 11.62196639741666004, -16.27693748946513708, 18.54958172136248606 ) ) ;
#9458=AXIS2_PLACEMENT_3D ( 'NONE', #7219, #19540, #14402 ) ;
#9459=CARTESIAN_POINT ( 'NONE',  ( -6.476765594713846497, 15.80122980073391936, 19.08844262864050023 ) ) ;
#9460=CARTESIAN_POINT ( 'NONE',  ( 4.467866064779363988, 16.43745301482979926, 5.749228751562096562 ) ) ;
#9462=CARTESIAN_POINT ( 'NONE',  ( 0.3518703668723790479, -19.99690444156084013, 7.652108011868850035 ) ) ;
#9463=AXIS2_PLACEMENT_3D ( 'NONE', #30046, #15540, #18197 ) ;
#9464=CARTESIAN_POINT ( 'NONE',  ( -11.64054540341807353, 16.26338533980436907, 24.50000000000000000 ) ) ;
#9470=EDGE_CURVE ( 'NONE', #15693, #2154, #10124, .T. ) ;
#9471=ORIENTED_EDGE ( 'NONE', *, *, #21960, .F. ) ;
#9472=CARTESIAN_POINT ( 'NONE',  ( -18.29014699721056303, -8.135908015825709327, 7.500898271101006820 ) ) ;
#9473=CARTESIAN_POINT ( 'NONE',  ( 9.755064781586030520, 13.32952022457704544, 1.500000000000000000 ) ) ;
#9474=CARTESIAN_POINT ( 'NONE',  ( -0.1864951924744762124, -20.01724188655222747, 5.796888747622817029 ) ) ;
#9478=CARTESIAN_POINT ( 'NONE',  ( -19.93005420669540584, 1.873390432278237983, 20.13759033520874908 ) ) ;
#9481=DIRECTION ( 'NONE',  ( -0.2817325568414296710, 0.9594929736144973687, 0.000000000000000000 ) ) ;
#9484=ORIENTED_EDGE ( 'NONE', *, *, #22202, .T. ) ;
#9485=CARTESIAN_POINT ( 'NONE',  ( 4.507962051892417499, 19.48556068265256513, 18.73377938172347612 ) ) ;
#9486=CARTESIAN_POINT ( 'NONE',  ( 0.000000000000000000, 0.000000000000000000, 0.000000000000000000 ) ) ;
#9491=CARTESIAN_POINT ( 'NONE',  ( 18.73355814148580833, -7.053980495653730642, 19.36813350477385143 ) ) ;
#9492=CARTESIAN_POINT ( 'NONE',  ( 19.57830992477560272, 4.170884463584000557, 19.58863275299554019 ) ) ;
#9495=ORIENTED_EDGE ( 'NONE', *, *, #214, .F. ) ;
#9496=CARTESIAN_POINT ( 'NONE',  ( 15.44332723073812907, -7.163653983989226148, 18.83976166372256245 ) ) ;
#9498=EDGE_LOOP ( 'NONE', ( #18079, #8690, #23484, #21796 ) ) ;
#9500=CARTESIAN_POINT ( 'NONE',  ( -0.2303554413151768232, -17.01973167556347377, 19.41069149716888020 ) ) ;
#9501=CARTESIAN_POINT ( 'NONE',  ( 1.709141304117140825, -16.98942507101831367, 6.233981582756856987 ) ) ;
#9504=CARTESIAN_POINT ( 'NONE',  ( 16.75466217413941905, 3.123260753354262231, 18.34969686940296185 ) ) ;
#9507=CARTESIAN_POINT ( 'NONE',  ( 9.326937650406421199, -14.24778824691897761, 7.429667576816606278 ) ) ;
#9509=AXIS2_PLACEMENT_3D ( 'NONE', #12312, #15240, #26656 ) ;
#9514=CARTESIAN_POINT ( 'NONE',  ( -9.958038337755702685, 17.34466697471556529, 24.50000000000000000 ) ) ;
#9520=ORIENTED_EDGE ( 'NONE', *, *, #16757, .T. ) ;
#9521=CARTESIAN_POINT ( 'NONE',  ( -8.824744466605359605, -8.513189541288717521, 1.500000000000001332 ) ) ;
#9524=ORIENTED_EDGE ( 'NONE', *, *, #12819, .F. ) ;
#9525=CARTESIAN_POINT ( 'NONE',  ( 12.24063095261064404, 4.490763173670002217, 1.500000000000001332 ) ) ;
#9527=LINE ( 'NONE', #4092, #30367 ) ;
#9539=CARTESIAN_POINT ( 'NONE',  ( 10.88769261259305132, -16.77715788799338981, 20.32243167357988867 ) ) ;
#9540=VERTEX_POINT ( 'NONE', #7790 ) ;
#9545=LINE ( 'NONE', #497, #24235 ) ;
#9546=ORIENTED_EDGE ( 'NONE', *, *, #5401, .F. ) ;
#9547=DIRECTION ( 'NONE',  ( 1.000000000000000000, 0.000000000000000000, 0.000000000000000000 ) ) ;
#9549=CARTESIAN_POINT ( 'NONE',  ( -15.01939917408024527, -8.081071717223313300, 20.29915277494337644 ) ) ;
#9550=CARTESIAN_POINT ( 'NONE',  ( -9.131494062835631809, -2.555255504830934221, 21.50000000000000000 ) ) ;
#9552=VECTOR ( 'NONE', #17161, 1000.000000000000000 ) ;
#9555=CYLINDRICAL_SURFACE ( 'NONE', #17385, 9.482273699623480212 ) ;
#9561=ORIENTED_EDGE ( 'NONE', *, *, #14735, .T. ) ;
#9563=DIRECTION ( 'NONE',  ( 1.000000000000000000, 0.000000000000000000, 0.000000000000000000 ) ) ;
#9564=ORIENTED_EDGE ( 'NONE', *, *, #1798, .T. ) ;
#9565=EDGE_CURVE ( 'NONE', #22425, #4276, #26701, .T. ) ;
#9566=ORIENTED_EDGE ( 'NONE', *, *, #1395, .F. ) ;
#9567=ADVANCED_FACE ( 'NONE', ( #24155 ), #2803, .F. ) ;
#9568=DIRECTION ( 'NONE',  ( 1.000000000000000000, 0.000000000000000000, 0.000000000000000000 ) ) ;
#9569=CIRCLE ( 'NONE', #12566, 9.482273699623480212 ) ;
#9572=ORIENTED_EDGE ( 'NONE', *, *, #2848, .T. ) ;
#9574=CARTESIAN_POINT ( 'NONE',  ( 0.1486850733125462121, -17.02875910996195685, 18.55820869691756769 ) ) ;
#9576=CARTESIAN_POINT ( 'NONE',  ( -10.24254388992508602, -17.19919274694469280, 7.603368798681074736 ) ) ;
#9579=CARTESIAN_POINT ( 'NONE',  ( 1.111517487559788409, -17.01912455222412035, 20.29915277494337644 ) ) ;
#9583=FACE_OUTER_BOUND ( 'NONE', #8089, .T. ) ;
#9584=CARTESIAN_POINT ( 'NONE',  ( 11.77016209912415690, 12.36695356451125249, 19.89182036555910571 ) ) ;
#9589=CARTESIAN_POINT ( 'NONE',  ( 3.896869771148438577, -16.82098518409776489, -0.6213203435596476032 ) ) ;
#9592=CARTESIAN_POINT ( 'NONE',  ( -19.91153203745396993, 1.881428233485404666, 7.454606537396340826 ) ) ;
#9595=CARTESIAN_POINT ( 'NONE',  ( -15.19605639364643324, -7.717080560943919032, 18.34969686940295830 ) ) ;
#9599=ORIENTED_EDGE ( 'NONE', *, *, #11109, .F. ) ;
#9604=CARTESIAN_POINT ( 'NONE',  ( 11.33091155972627462, -16.48105488812121067, 18.37545668562167123 ) ) ;
#9607=CARTESIAN_POINT ( 'NONE',  ( 17.99235278053350839, -8.774603096602955787, 18.80699882434806369 ) ) ;
#9608=CARTESIAN_POINT ( 'NONE',  ( 5.303645853345009265, 19.30241027580586177, 7.652108011868850035 ) ) ;
#9611=CARTESIAN_POINT ( 'NONE',  ( 5.413395986729065079, 19.27227163692344902, 20.34789198813115263 ) ) ;
#9613=CARTESIAN_POINT ( 'NONE',  ( 11.81884104268967839, 12.31686436340674895, 7.280727868105637768 ) ) ;
#9614=CARTESIAN_POINT ( 'NONE',  ( -11.40980092660686829, 6.310027164379044429, 1.500000000000001332 ) ) ;
#9618=AXIS2_PLACEMENT_3D ( 'NONE', #22727, #10897, #20403 ) ;
#9622=CARTESIAN_POINT ( 'NONE',  ( -15.56928374346769850, -6.880100827600172941, 6.420335371522007506 ) ) ;
#9624=CARTESIAN_POINT ( 'NONE',  ( 14.18379620663259288, 14.10035196125401313, 6.788986777570696241 ) ) ;
#9625=CARTESIAN_POINT ( 'NONE',  ( -0.4401303402703778955, -20.01320326077421186, 6.018569869498933578 ) ) ;
#9629=CARTESIAN_POINT ( 'NONE',  ( -19.94392260440443110, 1.716525891962610961, 19.97651184436794125 ) ) ;
#9631=EDGE_LOOP ( 'NONE', ( #30102, #30694, #23612, #22766 ) ) ;
#9632=CARTESIAN_POINT ( 'NONE',  ( 11.29839223038184848, -16.52442514205455737, 20.32367522806703874 ) ) ;
#9633=CARTESIAN_POINT ( 'NONE',  ( 9.056208293496307959, -2.810445847081888715, 13.00000000000000178 ) ) ;
#9636=AXIS2_PLACEMENT_3D ( 'NONE', #18722, #302, #19339 ) ;
#9637=CARTESIAN_POINT ( 'NONE',  ( 4.805983152666241764, 19.41435796516023515, 20.22386025856690139 ) ) ;
#9638=EDGE_CURVE ( 'NONE', #24939, #12796, #29105, .T. ) ;
#9641=ORIENTED_EDGE ( 'NONE', *, *, #4026, .F. ) ;
#9645=CYLINDRICAL_SURFACE ( 'NONE', #5328, 20.00000000000000000 ) ;
#9646=CARTESIAN_POINT ( 'NONE',  ( -15.51115086193519055, 12.62612245312785575, 20.32200205377524327 ) ) ;
#9647=CARTESIAN_POINT ( 'NONE',  ( 0.000000000000000000, 0.000000000000000000, 21.50000000000000000 ) ) ;
#9649=CYLINDRICAL_SURFACE ( 'NONE', #5354, 20.00000000000000355 ) ;
#9653=CIRCLE ( 'NONE', #10655, 9.482273699623480212 ) ;
#9654=FACE_OUTER_BOUND ( 'NONE', #30462, .T. ) ;
#9655=CARTESIAN_POINT ( 'NONE',  ( -14.78913018809137192, 13.49064936509565982, 19.87181966307587544 ) ) ;
#9656=CARTESIAN_POINT ( 'NONE',  ( -10.05618025891932277, -17.30842068227157071, 18.50655187082627862 ) ) ;
#9658=CARTESIAN_POINT ( 'NONE',  ( 1.043163081497040290, -17.02278858106077308, 20.34789198813115263 ) ) ;
#9659=CARTESIAN_POINT ( 'NONE',  ( 16.80805182381674712, 2.764250834391621225, 18.44501272782439827 ) ) ;
#9660=EDGE_LOOP ( 'NONE', ( #19748, #13634, #3232, #15468 ) ) ;
#9663=CARTESIAN_POINT ( 'NONE',  ( -15.63429437150528756, 12.50148542865848356, 7.559636331181775581 ) ) ;
#9664=CARTESIAN_POINT ( 'NONE',  ( -2.703030265324078307, -12.75514121382991384, 1.500000000000001332 ) ) ;
#9671=CARTESIAN_POINT ( 'NONE',  ( 18.44250036706183593, -7.738792361249054785, 18.37545668562167123 ) ) ;
#9674=CARTESIAN_POINT ( 'NONE',  ( -5.723804255145592101, 19.16384832744316213, 5.676722608126686609 ) ) ;
#9679=DIRECTION ( 'NONE',  ( -0.000000000000000000, -0.000000000000000000, 1.000000000000000000 ) ) ;
#9680=ORIENTED_EDGE ( 'NONE', *, *, #6561, .F. ) ;
#9681=CARTESIAN_POINT ( 'NONE',  ( 18.65245237681030588, -7.265846841151808455, 7.280727868105637768 ) ) ;
#9692=DIRECTION ( 'NONE',  ( -0.000000000000000000, -0.000000000000000000, 1.000000000000000000 ) ) ;
#9698=ORIENTED_EDGE ( 'NONE', *, *, #8042, .T. ) ;
#9699=LINE ( 'NONE', #12049, #8585 ) ;
#9701=DIRECTION ( 'NONE',  ( 0.000000000000000000, 0.000000000000000000, 1.000000000000000000 ) ) ;
#9707=DIRECTION ( 'NONE',  ( 0.9096319953545185522, -0.4154150130018860465, 0.000000000000000000 ) ) ;
#9708=ORIENTED_EDGE ( 'NONE', *, *, #25458, .F. ) ;
#9711=CARTESIAN_POINT ( 'NONE',  ( 8.430595340551260364, -4.340342926364983533, 21.50000000000000000 ) ) ;
#9712=CARTESIAN_POINT ( 'NONE',  ( 11.82521593960875173, 5.400395169024529984, 1.500000000000001332 ) ) ;
#9714=VECTOR ( 'NONE', #1128, 1000.000000000000000 ) ;
#9716=CARTESIAN_POINT ( 'NONE',  ( -9.819201815016004531, -17.42389611976319941, 7.272192800924331735 ) ) ;
#9721=ADVANCED_FACE ( 'NONE', ( #555 ), #3210, .T. ) ;
#9722=CARTESIAN_POINT ( 'NONE',  ( -9.846411740200883500, -17.42855948811278566, 7.280727868105637768 ) ) ;
#9723=CARTESIAN_POINT ( 'NONE',  ( -9.471281197126605989, -0.4564504349074042788, 1.500000000000001332 ) ) ;
#9724=CARTESIAN_POINT ( 'NONE',  ( 1.224038712338731072, -19.98030457043141084, 18.82680253904184298 ) ) ;
#9725=ORIENTED_EDGE ( 'NONE', *, *, #14601, .F. ) ;
#9728=CARTESIAN_POINT ( 'NONE',  ( 14.66647055262615318, 13.62412221374329846, 18.39992786714538298 ) ) ;
#9729=DIRECTION ( 'NONE',  ( 0.000000000000000000, 0.000000000000000000, 1.000000000000000000 ) ) ;
#9731=EDGE_CURVE ( 'NONE', #5896, #6583, #3273, .T. ) ;
#9733=CARTESIAN_POINT ( 'NONE',  ( -17.86170306354900816, -9.037578821739909785, 5.749491821935610147 ) ) ;
#9734=CARTESIAN_POINT ( 'NONE',  ( -6.403603917672690216, 18.96607824920917551, 5.749491821935610147 ) ) ;
#9735=CARTESIAN_POINT ( 'NONE',  ( 2.555255504830965751, -9.131494062835621150, 1.500000000000001332 ) ) ;
#9739=CARTESIAN_POINT ( 'NONE',  ( -18.43314756787627928, -7.806103702558631952, 18.90679857307105749 ) ) ;
#9743=ADVANCED_FACE ( 'NONE', ( #15522 ), #29571, .T. ) ;
#9745=CARTESIAN_POINT ( 'NONE',  ( -13.30548897721377699, 10.64932510079500538, 7.652108011868850035 ) ) ;
#9750=CARTESIAN_POINT ( 'NONE',  ( 15.72291199960844743, -6.567794255929246816, 18.36582235739946611 ) ) ;
#9752=CARTESIAN_POINT ( 'NONE',  ( 5.016833900951458425, 16.26516650762553695, 6.755862304746362845 ) ) ;
#9753=ADVANCED_FACE ( 'NONE', ( #10542 ), #10224, .F. ) ;
#9756=CARTESIAN_POINT ( 'NONE',  ( 14.35775550668713407, 13.94852561378611533, 7.280727868105637768 ) ) ;
#9758=CYLINDRICAL_SURFACE ( 'NONE', #21792, 9.482273699623480212 ) ;
#9760=VERTEX_POINT ( 'NONE', #25183 ) ;
#9762=AXIS2_PLACEMENT_3D ( 'NONE', #23358, #9027, #9481 ) ;
#9767=ORIENTED_EDGE ( 'NONE', *, *, #18702, .F. ) ;
#9769=CARTESIAN_POINT ( 'NONE',  ( -4.163336342344337027E-14, 1.387778780781445676E-14, 21.50000000000000000 ) ) ;
#9770=CARTESIAN_POINT ( 'NONE',  ( 14.33033395197103843, 13.95171706641510490, 7.272192800924335288 ) ) ;
#9771=DIRECTION ( 'NONE',  ( 1.000000000000000000, 0.000000000000000000, 0.000000000000000000 ) ) ;
#9773=DIRECTION ( 'NONE',  ( 0.9096319953545185522, -0.4154150130018859910, -0.000000000000000000 ) ) ;
#9774=DIRECTION ( 'NONE',  ( -0.000000000000000000, -0.000000000000000000, 1.000000000000000000 ) ) ;
#9781=LINE ( 'NONE', #424, #28193 ) ;
#9782=CARTESIAN_POINT ( 'NONE',  ( 0.000000000000000000, 0.000000000000000000, 21.50000000000000000 ) ) ;
#9783=ORIENTED_EDGE ( 'NONE', *, *, #14133, .T. ) ;
#9790=ADVANCED_FACE ( 'NONE', ( #13663 ), #11314, .F. ) ;
#9793=CARTESIAN_POINT ( 'NONE',  ( 12.35846532919128116, 11.73919094318043399, 20.34789198813115263 ) ) ;
#9794=FACE_OUTER_BOUND ( 'NONE', #30531, .T. ) ;
#9796=ORIENTED_EDGE ( 'NONE', *, *, #6379, .F. ) ;
#9797=CARTESIAN_POINT ( 'NONE',  ( 16.11353791281286973, -5.634185590772404773, 19.97651184436794125 ) ) ;
#9798=CARTESIAN_POINT ( 'NONE',  ( 19.57381806301096105, 4.191719245021452878, 19.47783254395485031 ) ) ;
#9802=CARTESIAN_POINT ( 'NONE',  ( 15.81223572262636878, -6.365019322297388094, 20.34789198813115263 ) ) ;
#9804=VECTOR ( 'NONE', #14938, 1000.000000000000000 ) ;
#9805=EDGE_LOOP ( 'NONE', ( #5898, #25141, #6827, #24175 ) ) ;
#9806=CIRCLE ( 'NONE', #6796, 0.7500000000000002220 ) ;
#9809=CARTESIAN_POINT ( 'NONE',  ( -12.78170796079387017, 11.24374406685325489, 18.90679857307105749 ) ) ;
#9810=ADVANCED_FACE ( 'NONE', ( #3683 ), #5651, .T. ) ;
#9812=CARTESIAN_POINT ( 'NONE',  ( -9.833673822381070906, -17.43574673801737873, 18.73743063545763121 ) ) ;
#9814=CARTESIAN_POINT ( 'NONE',  ( 9.755064781586030520, 13.32952022457704544, -0.6213203435596476032 ) ) ;
#9816=ORIENTED_EDGE ( 'NONE', *, *, #12500, .T. ) ;
#9819=CARTESIAN_POINT ( 'NONE',  ( 14.96983285839274380, 13.26353275515934449, 20.34789198813115263 ) ) ;
#9820=AXIS2_PLACEMENT_3D ( 'NONE', #7489, #23536, #11697 ) ;
#9821=DIRECTION ( 'NONE',  ( 1.000000000000000000, 0.000000000000000000, 0.000000000000000000 ) ) ;
#9822=EDGE_LOOP ( 'NONE', ( #10659, #27977, #6308, #24137 ) ) ;
#9827=CARTESIAN_POINT ( 'NONE',  ( 18.70942253818555656, -7.068249826530433211, 19.08830981656266346 ) ) ;
#9828=CARTESIAN_POINT ( 'NONE',  ( 15.81416692036122917, -6.360574302898113430, 5.652196082368483587 ) ) ;
#9834=FACE_BOUND ( 'NONE', #29948, .T. ) ;
#9839=CIRCLE ( 'NONE', #24802, 9.482273699623480212 ) ;
#9840=CARTESIAN_POINT ( 'NONE',  ( 18.67779315278252383, -7.200759110456479206, 7.196036389296800451 ) ) ;
#9846=B_SPLINE_CURVE_WITH_KNOTS ( 'NONE', 3,
 ( #24055, #12068, #29059, #24523, #9877, #16901, #17046, #200, #15009, #28911, #3017, #19854, #9716, #8014, #17516, #12214, #26417, #354 ),
 .UNSPECIFIED., .F., .F.,
 ( 4, 2, 2, 2, 2, 2, 2, 2, 4 ),
 ( 0.000000000000000000, 0.0003967869494442862583, 0.0007935738988885725166, 0.001190360848332858721, 0.001587147797777145033, 0.001983934747221431129, 0.002380721696665717441, 0.002777508646110003754, 0.003174295595554290066 ),
 .UNSPECIFIED. ) ;
#9847=DIRECTION ( 'NONE',  ( -0.000000000000000000, -0.000000000000000000, 1.000000000000000000 ) ) ;
#9850=CARTESIAN_POINT ( 'NONE',  ( 0.9307681286968549905, -9.436481611552757442, 21.50000000000000000 ) ) ;
#9852=CARTESIAN_POINT ( 'NONE',  ( -10.51100883930069863, -17.01524884273342053, 5.652196082369965069 ) ) ;
#9855=ORIENTED_EDGE ( 'NONE', *, *, #3106, .T. ) ;
#9856=CARTESIAN_POINT ( 'NONE',  ( 15.44249669564394267, -7.165351778271005223, 7.156916968540301127 ) ) ;
#9866=VECTOR ( 'NONE', #10587, 1000.000000000000000 ) ;
#9874=CARTESIAN_POINT ( 'NONE',  ( 7.856594496258195726, 4.390207617113981442, 1.500000000000001332 ) ) ;
#9876=ORIENTED_EDGE ( 'NONE', *, *, #20952, .F. ) ;
#9877=CARTESIAN_POINT ( 'NONE',  ( -9.978083804712657212, -17.33339668284229163, 5.853797745100183469 ) ) ;
#9880=CARTESIAN_POINT ( 'NONE',  ( 0.1201197967225753199, -20.01774464624826777, 20.32842677360128292 ) ) ;
#9882=CARTESIAN_POINT ( 'NONE',  ( -9.772441304892778291, -17.47026709695450464, 6.131018562779544823 ) ) ;
#9884=CARTESIAN_POINT ( 'NONE',  ( 4.644508076436818733, 16.38413139296123688, 20.14907003336613300 ) ) ;
#9885=CARTESIAN_POINT ( 'NONE',  ( 1.208994807697891138, -19.98122169387827896, 19.89182036555910571 ) ) ;
#9887=ORIENTED_EDGE ( 'NONE', *, *, #28796, .T. ) ;
#9892=LINE ( 'NONE', #30791, #174 ) ;
#9893=ORIENTED_EDGE ( 'NONE', *, *, #3494, .F. ) ;
#9896=CARTESIAN_POINT ( 'NONE',  ( -17.91073422896667466, -8.940227287121103927, 5.704143890883081269 ) ) ;
#9897=CARTESIAN_POINT ( 'NONE',  ( -6.359874605901117306, 15.84393421166759097, 7.196036389296800451 ) ) ;
#9900=CARTESIAN_POINT ( 'NONE',  ( -7.869584159753960861, 10.39565510934976977, 24.50000000000000000 ) ) ;
#9901=CARTESIAN_POINT ( 'NONE',  ( 4.102102735472459294, -8.549050687778176894, 21.50000000000000000 ) ) ;
#9902=ORIENTED_EDGE ( 'NONE', *, *, #23266, .T. ) ;
#9906=PRODUCT_DEFINITION_FORMATION_WITH_SPECIFIED_SOURCE ( 'ANY', '', #23591, .NOT_KNOWN. ) ;
#9908=CARTESIAN_POINT ( 'NONE',  ( 0.6479391102675158276, -17.02974303764478137, 7.652108011868854476 ) ) ;
#9909=EDGE_LOOP ( 'NONE', ( #7350, #7394, #21128, #28372 ) ) ;
#9912=CIRCLE ( 'NONE', #19865, 9.482273699623480212 ) ;
#9915=CARTESIAN_POINT ( 'NONE',  ( 4.817555027346758223, 16.32979927342787718, 19.96783386855779341 ) ) ;
#9928=CARTESIAN_POINT ( 'NONE',  ( -15.55662731361435469, -6.910399801605406012, 6.310736198168394928 ) ) ;
#9932=EDGE_CURVE ( 'NONE', #24994, #22249, #2296, .T. ) ;
#9933=CARTESIAN_POINT ( 'NONE',  ( 0.3541519782205873601, -20.01464289576668065, 5.652196082367002994 ) ) ;
#9935=CYLINDRICAL_SURFACE ( 'NONE', #7794, 0.7500000000000002220 ) ;
#9936=FACE_OUTER_BOUND ( 'NONE', #7012, .T. ) ;
#9940=ADVANCED_FACE ( 'NONE', ( #10654 ), #24684, .F. ) ;
#9943=CARTESIAN_POINT ( 'NONE',  ( 5.169584817211991812, 19.32078214751396317, 7.652108011868850923 ) ) ;
#9944=EDGE_CURVE ( 'NONE', #7727, #30552, #22229, .T. ) ;
#9946=EDGE_LOOP ( 'NONE', ( #2581, #9190, #27744, #25880 ) ) ;
#9951=AXIS2_PLACEMENT_3D ( 'NONE', #21522, #21678, #14666 ) ;
#9952=CARTESIAN_POINT ( 'NONE',  ( 15.45804667738991967, 12.71867858434618093, 19.87181966307587544 ) ) ;
#9953=CARTESIAN_POINT ( 'NONE',  ( -11.24586906513001416, -16.56046035145272555, 6.111214848085761986 ) ) ;
#9955=CARTESIAN_POINT ( 'NONE',  ( 16.05603743463488797, -5.780788835868658992, 20.13759033520874908 ) ) ;
#9958=ORIENTED_EDGE ( 'NONE', *, *, #4028, .F. ) ;
#9959=DIRECTION ( 'NONE',  ( -0.8412535328311804284, 0.5406408174555987767, 0.000000000000000000 ) ) ;
#9965=EDGE_CURVE ( 'NONE', #17954, #12796, #14243, .T. ) ;
#9970=CARTESIAN_POINT ( 'NONE',  ( -6.485253725360694332, 18.93805017237212951, 20.19593175699879595 ) ) ;
#9971=CARTESIAN_POINT ( 'NONE',  ( -15.06643696584252190, 13.18059642443756907, 20.25336174263950184 ) ) ;
#9972=VECTOR ( 'NONE', #8994, 1000.000000000000000 ) ;
#9973=CARTESIAN_POINT ( 'NONE',  ( -8.257638164125266300, -14.92340941578111035, 18.39992786714538298 ) ) ;
#9974=EDGE_CURVE ( 'NONE', #28528, #17576, #27721, .T. ) ;
#9976=CARTESIAN_POINT ( 'NONE',  ( -15.75094665830067697, -12.32508334119358828, 24.50000000000000000 ) ) ;
#9978=ORIENTED_EDGE ( 'NONE', *, *, #2777, .T. ) ;
#9980=CARTESIAN_POINT ( 'NONE',  ( -16.96555893289282935, 1.647560171710579002, 5.652196082364320695 ) ) ;
#9982=DIRECTION ( 'NONE',  ( 1.000000000000000000, 0.000000000000000000, 0.000000000000000000 ) ) ;
#9983=CARTESIAN_POINT ( 'NONE',  ( 19.87646685382696177, 2.220054991963873903, 6.913388067999417963 ) ) ;
#9985=ORIENTED_EDGE ( 'NONE', *, *, #5345, .T. ) ;
#9986=CARTESIAN_POINT ( 'NONE',  ( 10.58781394000596165, -16.96782583993082483, 7.454139397117725885 ) ) ;
#9987=CARTESIAN_POINT ( 'NONE',  ( -5.279695238918636235, 19.30927203514150747, 7.359006845440219102 ) ) ;
#9988=CARTESIAN_POINT ( 'NONE',  ( 12.18183868330171826, 11.93592587879421174, 7.652108011868850923 ) ) ;
#9993=EDGE_CURVE ( 'NONE', #24284, #26415, #18254, .T. ) ;
#9996=DIRECTION ( 'NONE',  ( 1.000000000000000000, 0.000000000000000000, 0.000000000000000000 ) ) ;
#9997=EDGE_LOOP ( 'NONE', ( #15122, #4034, #26431, #16626 ) ) ;
#10001=CARTESIAN_POINT ( 'NONE',  ( 15.98415658701447839, -5.958736450466536105, 7.559636331181775581 ) ) ;
#10002=CARTESIAN_POINT ( 'NONE',  ( 16.58213327075252863, 4.067275193330053717, 18.84329447212444109 ) ) ;
#10003=DIRECTION ( 'NONE',  ( 0.000000000000000000, 0.000000000000000000, 1.000000000000000000 ) ) ;
#10005=CARTESIAN_POINT ( 'NONE',  ( 3.613053539807239645, 16.67204840528144061, 5.749491821935610147 ) ) ;
#10009=CIRCLE ( 'NONE', #29429, 9.482273699623480212 ) ;
#10011=CARTESIAN_POINT ( 'NONE',  ( 9.860909911264737815, -13.90333503211346944, 20.34789198813115263 ) ) ;
#10019=CARTESIAN_POINT ( 'NONE',  ( -14.88329716083760346, -8.348731837201613715, 20.13759033520874908 ) ) ;
#10020=CYLINDRICAL_SURFACE ( 'NONE', #805, 1.000000000000007772 ) ;
#10021=CARTESIAN_POINT ( 'NONE',  ( -15.01328179936713880, 13.21424408877643941, 20.22277707861862339 ) ) ;
#10022=CARTESIAN_POINT ( 'NONE',  ( 4.299378382534376541, 16.48726736029815143, 5.676815824193227833 ) ) ;
#10024=LINE ( 'NONE', #7689, #17454 ) ;
#10035=VERTEX_POINT ( 'NONE', #25315 ) ;
#10036=CYLINDRICAL_SURFACE ( 'NONE', #28718, 20.00000000000000000 ) ;
#10038=ORIENTED_EDGE ( 'NONE', *, *, #24867, .T. ) ;
#10042=CARTESIAN_POINT ( 'NONE',  ( -7.667077102831937552, 13.77986170986486592, -0.6213203435596476032 ) ) ;
#10043=DIRECTION ( 'NONE',  ( 1.000000000000000000, 0.000000000000000000, 0.000000000000000000 ) ) ;
#10044=EDGE_LOOP ( 'NONE', ( #10488, #23598, #27969, #8163 ) ) ;
#10046=DIRECTION ( 'NONE',  ( 0.000000000000000000, 0.000000000000000000, 1.000000000000000000 ) ) ;
#10047=CARTESIAN_POINT ( 'NONE',  ( 11.65981318837298453, 12.47865322263302446, 19.36813350477385143 ) ) ;
#10052=CARTESIAN_POINT ( 'NONE',  ( -17.96015518819250545, -8.839856506746546216, 5.678370764302467677 ) ) ;
#10053=CARTESIAN_POINT ( 'NONE',  ( -5.621668343899179909, 16.09410144477765314, 5.652605728828373977 ) ) ;
#10054=DIRECTION ( 'NONE',  ( 1.000000000000000000, 0.000000000000000000, 0.000000000000000000 ) ) ;
#10057=ORIENTED_EDGE ( 'NONE', *, *, #21373, .T. ) ;
#10058=DIRECTION ( 'NONE',  ( -0.7557495743542581579, -0.6548607339452852116, 0.000000000000000000 ) ) ;
#10060=CARTESIAN_POINT ( 'NONE',  ( -12.77302042131097792, 11.25334833650868838, 7.080843742048788414 ) ) ;
#10061=DIRECTION ( 'NONE',  ( 1.000000000000000000, 0.000000000000000000, 0.000000000000000000 ) ) ;
#10064=CARTESIAN_POINT ( 'NONE',  ( 15.91946090815430104, -6.118695897821246454, 18.34938820207545263 ) ) ;
#10066=VERTEX_POINT ( 'NONE', #25478 ) ;
#10069=AXIS2_PLACEMENT_3D ( 'NONE', #5314, #2986, #26384 ) ;
#10070=DIRECTION ( 'NONE',  ( 0.000000000000000000, 0.000000000000000000, 1.000000000000000000 ) ) ;
#10075=CARTESIAN_POINT ( 'NONE',  ( -19.69223482763159083, 3.495123391383816447, 19.21471108562415253 ) ) ;
#10076=ORIENTED_EDGE ( 'NONE', *, *, #16826, .F. ) ;
#10080=CARTESIAN_POINT ( 'NONE',  ( -0.5073662589470756545, -20.01152162034081883, 6.111214848085761986 ) ) ;
#10081=CARTESIAN_POINT ( 'NONE',  ( 0.1262659238204208167, 8.999114229549594057, 1.500000000000001332 ) ) ;
#10085=ORIENTED_EDGE ( 'NONE', *, *, #17938, .F. ) ;
#10086=DIRECTION ( 'NONE',  ( 1.000000000000000000, 0.000000000000000000, 0.000000000000000000 ) ) ;
#10087=DIRECTION ( 'NONE',  ( 0.000000000000000000, 0.000000000000000000, -1.000000000000000000 ) ) ;
#10089=ORIENTED_EDGE ( 'NONE', *, *, #24457, .F. ) ;
#10094=CARTESIAN_POINT ( 'NONE',  ( 12.95659581195170773, 11.04149104205339427, 19.77662771831109367 ) ) ;
#10096=VECTOR ( 'NONE', #21030, 1000.000000000000000 ) ;
#10098=ORIENTED_EDGE ( 'NONE', *, *, #14304, .T. ) ;
#10101=CARTESIAN_POINT ( 'NONE',  ( 18.73275811567551230, -7.056106374802665115, 19.47783254395485031 ) ) ;
#10102=CARTESIAN_POINT ( 'NONE',  ( 16.63005575832078975, 3.830191698062870742, 18.56793045041961321 ) ) ;
#10105=DIRECTION ( 'NONE',  ( -1.000000000000000000, 0.000000000000000000, 0.000000000000000000 ) ) ;
#10110=CARTESIAN_POINT ( 'NONE',  ( -6.055745631507631899, 15.95075576291064223, 20.19593175699879595 ) ) ;
#10111=CARTESIAN_POINT ( 'NONE',  ( -12.96319695304515207, 11.04295072071645656, 20.12545155307891065 ) ) ;
#10114=VECTOR ( 'NONE', #19773, 1000.000000000000227 ) ;
#10116=CARTESIAN_POINT ( 'NONE',  ( -13.00999358272542494, -0.8602714556717691030, 1.500000000000001332 ) ) ;
#10119=CARTESIAN_POINT ( 'NONE',  ( -16.98411243466784271, 1.496360031252973233, 5.661398277488801867 ) ) ;
#10121=CARTESIAN_POINT ( 'NONE',  ( 19.81826808356698422, 2.692791747024147142, 7.526993102356318133 ) ) ;
#10123=ORIENTED_EDGE ( 'NONE', *, *, #6675, .T. ) ;
#10124=LINE ( 'NONE', #10444, #25777 ) ;
#10127=CARTESIAN_POINT ( 'NONE',  ( -10.47960520055065636, -7.757439966934454034, 1.500000000000001332 ) ) ;
#10129=CARTESIAN_POINT ( 'NONE',  ( 18.38841581631819011, -7.866599884335181869, 20.34789198813115263 ) ) ;
#10130=CARTESIAN_POINT ( 'NONE',  ( -15.56507824124772554, -6.890134373246081800, 6.910395520694542881 ) ) ;
#10131=CARTESIAN_POINT ( 'NONE',  ( 5.881244434206234217, 6.812559277181991391, 21.50000000000000000 ) ) ;
#10132=CARTESIAN_POINT ( 'NONE',  ( 5.291489565152560637, 19.28730510418394317, 5.652196082369965069 ) ) ;
#10133=ORIENTED_EDGE ( 'NONE', *, *, #20391, .F. ) ;
#10136=CARTESIAN_POINT ( 'NONE',  ( 0.3518703668723787148, -19.99690444156084723, 7.652108011868850035 ) ) ;
#10137=CARTESIAN_POINT ( 'NONE',  ( -17.58129253318381657, -9.534052292972814868, 19.21940439362674624 ) ) ;
#10138=CARTESIAN_POINT ( 'NONE',  ( 16.76050819728945385, 3.085824932809442700, 5.657991946698900598 ) ) ;
#10139=EDGE_CURVE ( 'NONE', #19771, #28210, #1617, .T. ) ;
#10140=ORIENTED_EDGE ( 'NONE', *, *, #18356, .F. ) ;
#10141=CARTESIAN_POINT ( 'NONE',  ( 12.99901289864995668, 10.98932263627886563, 6.864725433338323413 ) ) ;
#10144=CARTESIAN_POINT ( 'NONE',  ( 18.73437065802030332, -7.051821425362959417, 6.560937769032974209 ) ) ;
#10148=EDGE_CURVE ( 'NONE', #13827, #27530, #15793, .T. ) ;
#10152=DIRECTION ( 'NONE',  ( 0.000000000000000000, 0.000000000000000000, 1.000000000000000000 ) ) ;
#10154=CARTESIAN_POINT ( 'NONE',  ( 11.01999061743883956, -16.71182566173002471, 20.34789198813115263 ) ) ;
#10157=DIRECTION ( 'NONE',  ( -0.8412535328311804284, 0.5406408174555987767, 0.000000000000000000 ) ) ;
#10159=CARTESIAN_POINT ( 'NONE',  ( -15.95709955354365484, 12.08619843917607817, 19.03762469184452755 ) ) ;
#10160=DIRECTION ( 'NONE',  ( 1.000000000000000000, 0.000000000000000000, 0.000000000000000000 ) ) ;
#10161=VECTOR ( 'NONE', #22056, 1000.000000000000000 ) ;
#10163=ADVANCED_FACE ( 'NONE', ( #30297 ), #8920, .T. ) ;
#10169=ADVANCED_FACE ( 'NONE', ( #26494 ), #14056, .F. ) ;
#10175=ORIENTED_EDGE ( 'NONE', *, *, #28970, .F. ) ;
#10177=CYLINDRICAL_SURFACE ( 'NONE', #9458, 9.482273699623480212 ) ;
#10181=FACE_OUTER_BOUND ( 'NONE', #16828, .T. ) ;
#10183=ORIENTED_EDGE ( 'NONE', *, *, #7846, .F. ) ;
#10187=DIRECTION ( 'NONE',  ( 1.000000000000000000, 0.000000000000000000, 0.000000000000000000 ) ) ;
#10192=CARTESIAN_POINT ( 'NONE',  ( -10.94312936609102849, -16.74105124841231529, 7.526993102356320797 ) ) ;
#10198=ADVANCED_FACE ( 'NONE', ( #25233 ), #29561, .T. ) ;
#10200=CARTESIAN_POINT ( 'NONE',  ( 18.33793066653144876, -7.982499537706464920, 18.34798005863226678 ) ) ;
#10201=CARTESIAN_POINT ( 'NONE',  ( -6.507320782993285313, 15.78995902672676976, 6.672349528511551497 ) ) ;
#10202=CARTESIAN_POINT ( 'NONE',  ( 11.11866356627124297, -16.64591798801203737, 5.652196082364323360 ) ) ;
#10207=CARTESIAN_POINT ( 'NONE',  ( 11.23874228076938842, -11.06161525231356713, 1.500000000000001332 ) ) ;
#10208=CIRCLE ( 'NONE', #27652, 0.7500000000000006661 ) ;
#10210=CARTESIAN_POINT ( 'NONE',  ( -13.33237335330699302, 10.61702797731129877, 5.653912893140659257 ) ) ;
#10211=CARTESIAN_POINT ( 'NONE',  ( -0.2303554413151975844, -17.01973167556347377, 6.714907520933423690 ) ) ;
#10213=CARTESIAN_POINT ( 'NONE',  ( 16.14871318123685384, -5.543368461271793279, 18.84329447212444464 ) ) ;
#10215=ORIENTED_EDGE ( 'NONE', *, *, #11824, .F. ) ;
#10224=CYLINDRICAL_SURFACE ( 'NONE', #6371, 1.000000000000007772 ) ;
#10236=DIRECTION ( 'NONE',  ( -0.000000000000000000, -0.000000000000000000, 1.000000000000000000 ) ) ;
#10239=ORIENTED_EDGE ( 'NONE', *, *, #30854, .T. ) ;
#10243=ORIENTED_EDGE ( 'NONE', *, *, #8603, .T. ) ;
#10245=CARTESIAN_POINT ( 'NONE',  ( 14.91976180470934743, 13.34593040386456586, 18.34777357837152323 ) ) ;
#10248=CARTESIAN_POINT ( 'NONE',  ( -19.77136997667518159, 3.131761183015793648, 7.429667576816606278 ) ) ;
#10253=DIRECTION ( 'NONE',  ( 0.000000000000000000, 0.000000000000000000, 1.000000000000000000 ) ) ;
#10258=VERTEX_POINT ( 'NONE', #22887 ) ;
#10260=CARTESIAN_POINT ( 'NONE',  ( 16.56029649016585026, 4.170884463583997892, 6.892848776733236704 ) ) ;
#10270=CARTESIAN_POINT ( 'NONE',  ( -19.88823125026085492, 2.273432466552572695, 5.678370764302467677 ) ) ;
#10273=AXIS2_PLACEMENT_3D ( 'NONE', #5891, #10571, #29135 ) ;
#10282=CARTESIAN_POINT ( 'NONE',  ( -15.57728904105047718, -6.860944617588216943, 6.519181285484531685 ) ) ;
#10284=DIRECTION ( 'NONE',  ( 0.000000000000000000, 0.000000000000000000, 1.000000000000000000 ) ) ;
#10288=CARTESIAN_POINT ( 'NONE',  ( -9.660978277356432997, -17.51194513905170069, 19.61564845152805248 ) ) ;
#10290=LINE ( 'NONE', #310, #1749 ) ;
#10291=CARTESIAN_POINT ( 'NONE',  ( 16.77888236039448344, 2.967719242317201633, 7.632642797338977658 ) ) ;
#10294=CARTESIAN_POINT ( 'NONE',  ( 12.98391214946238748, 11.00790965981589586, 6.974106381145714018 ) ) ;
#10296=CARTESIAN_POINT ( 'NONE',  ( 18.69797757513550351, -7.147916136757723748, 7.098451512883313441 ) ) ;
#10297=VECTOR ( 'NONE', #15677, 1000.000000000000227 ) ;
#10299=CIRCLE ( 'NONE', #29742, 9.482273699623480212 ) ;
#10300=ORIENTED_EDGE ( 'NONE', *, *, #23080, .F. ) ;
#10302=CARTESIAN_POINT ( 'NONE',  ( 9.755064781586030520, 13.32952022457704544, 24.50000000000000000 ) ) ;
#10306=ADVANCED_FACE ( 'NONE', ( #18390 ), #30323, .T. ) ;
#10314=AXIS2_PLACEMENT_3D ( 'NONE', #27217, #19579, #30131 ) ;
#10320=EDGE_CURVE ( 'NONE', #21915, #27180, #9295, .T. ) ;
#10327=EDGE_CURVE ( 'NONE', #1600, #20446, #16947, .T. ) ;
#10328=CARTESIAN_POINT ( 'NONE',  ( 16.87925085231059441, 2.194398682741079298, 6.519181285484532573 ) ) ;
#10329=AXIS2_PLACEMENT_3D ( 'NONE', #22877, #30369, #3714 ) ;
#10330=CARTESIAN_POINT ( 'NONE',  ( 19.59736455876165806, 3.994007928088042281, 6.037995405461185072 ) ) ;
#10331=ORIENTED_EDGE ( 'NONE', *, *, #96, .F. ) ;
#10334=ORIENTED_EDGE ( 'NONE', *, *, #20800, .T. ) ;
#10340=CIRCLE ( 'NONE', #25280, 10.00000000000000000 ) ;
#10343=ORIENTED_EDGE ( 'NONE', *, *, #4835, .F. ) ;
#10346=EDGE_CURVE ( 'NONE', #13230, #3110, #7808, .T. ) ;
#10352=ORIENTED_EDGE ( 'NONE', *, *, #15708, .T. ) ;
#10355=CARTESIAN_POINT ( 'NONE',  ( -13.68208811019134785, -10.53240720452297374, -0.6213203435596476032 ) ) ;
#10360=AXIS2_PLACEMENT_3D ( 'NONE', #23682, #9358, #9982 ) ;
#10361=AXIS2_PLACEMENT_3D ( 'NONE', #77, #4908, #23606 ) ;
#10362=DIRECTION ( 'NONE',  ( -1.000000000000000000, 0.000000000000000000, 0.000000000000000000 ) ) ;
#10364=CARTESIAN_POINT ( 'NONE',  ( 11.81973518349029284, -16.15564139912475028, 7.196036389296800451 ) ) ;
#10372=FACE_OUTER_BOUND ( 'NONE', #17669, .T. ) ;
#10373=CARTESIAN_POINT ( 'NONE',  ( 8.606594496258196614, 4.390207617113981442, 1.500000000000001332 ) ) ;
#10375=CARTESIAN_POINT ( 'NONE',  ( 0.2718907111903831053, -17.03030470364403470, 7.526951045817045660 ) ) ;
#10377=CARTESIAN_POINT ( 'NONE',  ( -2.810445847081919357, -9.056208293496299078, 21.50000000000000000 ) ) ;
#10378=DIRECTION ( 'NONE',  ( 1.000000000000000000, 0.000000000000000000, 0.000000000000000000 ) ) ;
#10382=CARTESIAN_POINT ( 'NONE',  ( 4.806943871629679066, 16.33324523791881688, 18.71435384576123440 ) ) ;
#10383=B_SPLINE_SURFACE_WITH_KNOTS ( 'NONE', 3, 1, ( 
 ( #17288, #24460 ),
 ( #26346, #7623 ),
 ( #7778, #26821 ),
 ( #12309, #21811 ),
 ( #9971, #5446 ),
 ( #5283, #12153 ),
 ( #12769, #10111 ),
 ( #14949, #135 ),
 ( #3103, #7322 ),
 ( #9655, #21652 ),
 ( #19475, #16831 ),
 ( #17130, #19321 ),
 ( #12622, #7478 ),
 ( #26652, #14790 ),
 ( #22115, #19775 ),
 ( #24307, #16976 ),
 ( #29307, #19621 ),
 ( #7948, #4975 ),
 ( #286, #9809 ),
 ( #12475, #21965 ),
 ( #593, #27272 ),
 ( #8246, #29928 ),
 ( #15404, #13241 ),
 ( #5903, #6212 ),
 ( #914, #27121 ),
 ( #11473, #1386 ),
 ( #20095, #8566 ),
 ( #29463, #10431 ),
 ( #13088, #23311 ),
 ( #22729, #16298 ),
 ( #27586, #19945 ) ),
 .UNSPECIFIED., .F., .F., .F.,
 ( 4, 3, 3, 3, 3, 3, 3, 3, 3, 3, 4 ),
 ( 2, 2 ),
 ( 0.000000000000000000, 0.05425176834609614362, 0.1085332949128348518, 0.1623767749169379715, 0.2157504826133058717, 0.2688657508888169789, 0.3218907763505471364, 0.3749548578363334772, 0.4282048033836237666, 0.4818374082110496448, 0.4999999999131653494 ),
 ( 0.000000000000000000, 1.000000000000000000 ),
 .UNSPECIFIED. ) ;
#10384=CIRCLE ( 'NONE', #4895, 0.7500000000000006661 ) ;
#10389=DIRECTION ( 'NONE',  ( 0.1423148382732889461, 0.9898214418809321291, 0.000000000000000000 ) ) ;
#10395=DIRECTION ( 'NONE',  ( 1.000000000000000000, 0.000000000000000000, 0.000000000000000000 ) ) ;
#10396=LINE ( 'NONE', #8368, #27337 ) ;
#10397=CARTESIAN_POINT ( 'NONE',  ( 16.01701959600647385, -5.879758784200290300, 7.545655578832112020 ) ) ;
#10398=CARTESIAN_POINT ( 'NONE',  ( 8.413215745754998309, -3.196529495465417980, 1.500000000000001332 ) ) ;
#10405=AXIS2_PLACEMENT_3D ( 'NONE', #24178, #18750, #28267 ) ;
#10406=FACE_OUTER_BOUND ( 'NONE', #9631, .T. ) ;
#10407=FACE_OUTER_BOUND ( 'NONE', #8883, .T. ) ;
#10408=CIRCLE ( 'NONE', #13877, 20.00000000000000000 ) ;
#10412=CARTESIAN_POINT ( 'NONE',  ( 7.869584159753955532, 10.39565510934977333, 1.500000000000001332 ) ) ;
#10415=CARTESIAN_POINT ( 'NONE',  ( 15.49551216414738875, 12.67315350590407697, 19.77662771831109367 ) ) ;
#10419=CARTESIAN_POINT ( 'NONE',  ( 17.96625477203413723, -8.787278772463418264, 7.156831654632803463 ) ) ;
#10422=CARTESIAN_POINT ( 'NONE',  ( -5.738360882150000286, -7.548823014270624299, 21.50000000000000000 ) ) ;
#10424=CARTESIAN_POINT ( 'NONE',  ( 0.000000000000000000, 0.000000000000000000, 1.500000000000001332 ) ) ;
#10426=AXIS2_PLACEMENT_3D ( 'NONE', #13030, #6304, #27676 ) ;
#10428=CARTESIAN_POINT ( 'NONE',  ( -6.813581335325351596, 18.80366338534911463, 18.84486140012300126 ) ) ;
#10430=CARTESIAN_POINT ( 'NONE',  ( 19.60273500773784505, 4.055073576757204812, 6.131018562779544823 ) ) ;
#10431=CARTESIAN_POINT ( 'NONE',  ( -13.30790957887532500, 10.64596135573642144, 18.35377592296120497 ) ) ;
#10432=AXIS2_PLACEMENT_3D ( 'NONE', #24792, #3429, #29327 ) ;
#10435=LINE ( 'NONE', #2962, #17992 ) ;
#10436=CARTESIAN_POINT ( 'NONE',  ( -2.523760598493608232, -1.621922452366769907, 24.50000000000000000 ) ) ;
#10438=CARTESIAN_POINT ( 'NONE',  ( 9.769531821641358249, -13.96399651007160791, 5.657991946698900598 ) ) ;
#10443=ORIENTED_EDGE ( 'NONE', *, *, #1622, .F. ) ;
#10444=CARTESIAN_POINT ( 'NONE',  ( -11.40980092660686829, 6.310027164379044429, 1.500000000000001332 ) ) ;
#10446=DIRECTION ( 'NONE',  ( 0.000000000000000000, 0.000000000000000000, 1.000000000000000000 ) ) ;
#10451=ORIENTED_EDGE ( 'NONE', *, *, #2165, .T. ) ;
#10454=CARTESIAN_POINT ( 'NONE',  ( 14.89413573707701488, 13.37445272932972706, 5.652196082364320695 ) ) ;
#10455=CARTESIAN_POINT ( 'NONE',  ( 19.89210292178043460, 2.240810012149825781, 6.974106381145714018 ) ) ;
#10457=CARTESIAN_POINT ( 'NONE',  ( 12.77210943289888334, 11.26383436979580921, 5.862424720655265098 ) ) ;
#10458=ORIENTED_EDGE ( 'NONE', *, *, #20999, .F. ) ;
#10462=ORIENTED_EDGE ( 'NONE', *, *, #20024, .T. ) ;
#10463=CARTESIAN_POINT ( 'NONE',  ( 3.905960108394948449, 16.59621863701448419, 7.643931100913408550 ) ) ;
#10466=EDGE_CURVE ( 'NONE', #29559, #11919, #8812, .T. ) ;
#10471=ORIENTED_EDGE ( 'NONE', *, *, #214, .T. ) ;
#10474=CARTESIAN_POINT ( 'NONE',  ( -15.98738144660410931, 12.04609795553197671, 19.36813350477385143 ) ) ;
#10476=DIRECTION ( 'NONE',  ( 1.000000000000000000, 0.000000000000000000, 0.000000000000000000 ) ) ;
#10488=ORIENTED_EDGE ( 'NONE', *, *, #30575, .F. ) ;
#10496=AXIS2_PLACEMENT_3D ( 'NONE', #11675, #12298, #19312 ) ;
#10497=SHAPE_REPRESENTATION ( 'Rotor', ( #7396 ), #26315 ) ;
#10504=DIRECTION ( 'NONE',  ( 1.000000000000000000, 0.000000000000000000, 0.000000000000000000 ) ) ;
#10510=EDGE_LOOP ( 'NONE', ( #28794, #20341, #21478, #7944 ) ) ;
#10512=CARTESIAN_POINT ( 'NONE',  ( -6.145639756558239242, 15.91995507688107736, 7.441806358946449151 ) ) ;
#10513=CARTESIAN_POINT ( 'NONE',  ( 10.69227409735890078, -13.31703061742499017, 6.672349528511551497 ) ) ;
#10519=CARTESIAN_POINT ( 'NONE',  ( 14.44122519041005681, -13.83658248990206729, 24.50000000000000000 ) ) ;
#10527=CARTESIAN_POINT ( 'NONE',  ( 3.062151163506454665, 16.80153468414595253, 6.588756557121049795 ) ) ;
#10528=ADVANCED_FACE ( 'NONE', ( #5867 ), #29577, .F. ) ;
#10531=CARTESIAN_POINT ( 'NONE',  ( 5.335947603960575769, 19.29354331951100576, 18.34777357837151612 ) ) ;
#10540=AXIS2_PLACEMENT_3D ( 'NONE', #14199, #28411, #19194 ) ;
#10542=FACE_OUTER_BOUND ( 'NONE', #30249, .T. ) ;
#10554=CIRCLE ( 'NONE', #19498, 9.482273699623480212 ) ;
#10555=DIRECTION ( 'NONE',  ( 0.000000000000000000, 0.000000000000000000, 1.000000000000000000 ) ) ;
#10557=ORIENTED_EDGE ( 'NONE', *, *, #24420, .F. ) ;
#10567=DIRECTION ( 'NONE',  ( 0.000000000000000000, 0.000000000000000000, -1.000000000000000000 ) ) ;
#10569=EDGE_LOOP ( 'NONE', ( #2477, #9337, #2400, #8915 ) ) ;
#10570=CARTESIAN_POINT ( 'NONE',  ( 18.48179574117062529, -7.690589227441820164, 20.29915277494337644 ) ) ;
#10571=DIRECTION ( 'NONE',  ( 0.000000000000000000, 0.000000000000000000, 1.000000000000000000 ) ) ;
#10573=VERTEX_POINT ( 'NONE', #30482 ) ;
#10575=CARTESIAN_POINT ( 'NONE',  ( -4.697473163589096501, 16.36296782917919757, 19.85270094495842130 ) ) ;
#10580=CARTESIAN_POINT ( 'NONE',  ( 9.958038337755681368, 17.34466697471553331, 1.500000000000001332 ) ) ;
#10582=CARTESIAN_POINT ( 'NONE',  ( 16.65022252850694429, 3.724077645907917677, 7.500147780736496017 ) ) ;
#10584=CARTESIAN_POINT ( 'NONE',  ( -8.550548368345316064, -14.74545326172986570, 20.34789198813115263 ) ) ;
#10586=CARTESIAN_POINT ( 'NONE',  ( -9.072316094091473104, -14.41194981475155679, 7.453286057244485008 ) ) ;
#10587=DIRECTION ( 'NONE',  ( 0.000000000000000000, 0.000000000000000000, 1.000000000000000000 ) ) ;
#10588=ORIENTED_EDGE ( 'NONE', *, *, #27858, .T. ) ;
#10590=DIRECTION ( 'NONE',  ( 0.6548607339452852116, -0.7557495743542581579, 0.000000000000000000 ) ) ;
#10591=EDGE_CURVE ( 'NONE', #13891, #29673, #16263, .T. ) ;
#10592=CARTESIAN_POINT ( 'NONE',  ( 11.87672590887049751, -16.11366389249060305, 18.92976555901915603 ) ) ;
#10596=CARTESIAN_POINT ( 'NONE',  ( 18.08053511453368500, -8.550039048713406586, 20.14992337338002670 ) ) ;
#10600=VECTOR ( 'NONE', #1691, 1000.000000000000000 ) ;
#10602=ORIENTED_EDGE ( 'NONE', *, *, #16569, .T. ) ;
#10604=CARTESIAN_POINT ( 'NONE',  ( -6.778663211761420726, 6.630478080506977179, 1.500000000000001332 ) ) ;
#10609=CARTESIAN_POINT ( 'NONE',  ( 19.89498243266959676, 2.215034284604906922, 6.420335371522007506 ) ) ;
#10611=CARTESIAN_POINT ( 'NONE',  ( 12.43151381881690831, 11.65737597917812529, 5.657991946698900598 ) ) ;
#10612=ORIENTED_EDGE ( 'NONE', *, *, #5961, .T. ) ;
#10613=CARTESIAN_POINT ( 'NONE',  ( -13.99459037270471029, 9.787106705871224221, 19.61324152429827450 ) ) ;
#10614=CARTESIAN_POINT ( 'NONE',  ( -8.637616862297814890, 3.912171961292036482, 1.500000000000001332 ) ) ;
#10615=ORIENTED_EDGE ( 'NONE', *, *, #1425, .F. ) ;
#10616=VECTOR ( 'NONE', #15327, 1000.000000000000000 ) ;
#10617=CARTESIAN_POINT ( 'NONE',  ( 4.376647981176111202, 19.53331152111370628, 6.995624166085161910 ) ) ;
#10618=VECTOR ( 'NONE', #29397, 1000.000000000000000 ) ;
#10619=LINE ( 'NONE', #8735, #10660 ) ;
#10620=CARTESIAN_POINT ( 'NONE',  ( 5.888181818956395475, 19.11381997051147863, 18.54479204710284890 ) ) ;
#10621=B_SPLINE_CURVE_WITH_KNOTS ( 'NONE', 3,
 ( #11383, #2010, #6684, #9182, #25713, #13869, #11534, #2306, #11991, #21484, #21801, #28831, #26333, #5271, #28676, #9646, #440, #2946 ),
 .UNSPECIFIED., .F., .F.,
 ( 4, 2, 2, 2, 2, 2, 2, 2, 4 ),
 ( 0.000000000000000000, 0.0003967869494442920046, 0.0007935738988885840091, 0.001190360848332876068, 0.001587147797777168018, 0.001983934747221460185, 0.002380721696665752136, 0.002777508646110044086, 0.003174295595554332567 ),
 .UNSPECIFIED. ) ;
#10625=ORIENTED_EDGE ( 'NONE', *, *, #5968, .T. ) ;
#10634=CARTESIAN_POINT ( 'NONE',  ( -14.76283269969004230, 13.49301113316030865, 19.85261563089511228 ) ) ;
#10641=ORIENTED_EDGE ( 'NONE', *, *, #1556, .F. ) ;
#10642=CARTESIAN_POINT ( 'NONE',  ( 2.810445847081854964, 9.056208293496318618, 21.50000000000000000 ) ) ;
#10643=VERTEX_POINT ( 'NONE', #9124 ) ;
#10647=LINE ( 'NONE', #20157, #29869 ) ;
#10650=LINE ( 'NONE', #22348, #4391 ) ;
#10653=CARTESIAN_POINT ( 'NONE',  ( -12.24063095261064227, 4.490763173670005770, 24.50000000000000000 ) ) ;
#10654=FACE_OUTER_BOUND ( 'NONE', #16004, .T. ) ;
#10655=AXIS2_PLACEMENT_3D ( 'NONE', #19887, #8040, #17542 ) ;
#10656=CARTESIAN_POINT ( 'NONE',  ( -10.51513057463695233, -17.01270198993486460, 7.652108011868850035 ) ) ;
#10659=ORIENTED_EDGE ( 'NONE', *, *, #18754, .F. ) ;
#10660=VECTOR ( 'NONE', #1107, 1000.000000000000000 ) ;
#10661=CARTESIAN_POINT ( 'NONE',  ( -9.396043825398766813, -14.19290753657279858, 19.45164628100866722 ) ) ;
#10662=CARTESIAN_POINT ( 'NONE',  ( -18.02885658979140260, -8.699255478180120349, 7.652108011868850035 ) ) ;
#10665=CARTESIAN_POINT ( 'NONE',  ( 11.86528446860016928, -16.12209958341615135, 7.098451512883313441 ) ) ;
#10673=CARTESIAN_POINT ( 'NONE',  ( -12.91351154505913357, 11.09846585523631468, 5.940635272151477686 ) ) ;
#10674=CARTESIAN_POINT ( 'NONE',  ( 0.4564504349074358647, -9.471281197126604212, 21.50000000000000000 ) ) ;
#10678=CARTESIAN_POINT ( 'NONE',  ( -9.378051617232568304, -14.20529941771991567, 6.420335371522007506 ) ) ;
#10680=ORIENTED_EDGE ( 'NONE', *, *, #26931, .F. ) ;
#10681=CARTESIAN_POINT ( 'NONE',  ( -18.04155359371238632, -8.631455508453164782, 5.652196082369963293 ) ) ;
#10682=DIRECTION ( 'NONE',  ( -0.9898214418809326842, -0.1423148382732852824, 0.000000000000000000 ) ) ;
#10683=CARTESIAN_POINT ( 'NONE',  ( 19.69872561633594188, 3.460482060625763800, 18.37545668562167478 ) ) ;
#10684=ORIENTED_EDGE ( 'NONE', *, *, #25744, .T. ) ;
#10685=CARTESIAN_POINT ( 'NONE',  ( 11.53007546964075836, -16.34234030559856166, 5.779535427900761135 ) ) ;
#10691=CARTESIAN_POINT ( 'NONE',  ( -18.05883950494725099, -8.636531109380518600, 5.652196082367002106 ) ) ;
#10693=EDGE_CURVE ( 'NONE', #7304, #26027, #2315, .T. ) ;
#10695=EDGE_CURVE ( 'NONE', #15672, #2397, #30339, .T. ) ;
#10701=FACE_OUTER_BOUND ( 'NONE', #22757, .T. ) ;
#10706=ORIENTED_EDGE ( 'NONE', *, *, #3854, .F. ) ;
#10708=CYLINDRICAL_SURFACE ( 'NONE', #28383, 20.00000000000000355 ) ;
#10716=ORIENTED_EDGE ( 'NONE', *, *, #6228, .F. ) ;
#10718=CARTESIAN_POINT ( 'NONE',  ( -19.83108769839776642, 2.729924941536435057, 7.632642797338977658 ) ) ;
#10719=CARTESIAN_POINT ( 'NONE',  ( 18.00031268893095771, -8.717656915646674776, 6.033082186765049926 ) ) ;
#10723=CARTESIAN_POINT ( 'NONE',  ( -5.062693764981720967, 16.26276758967388503, 18.47056384035244037 ) ) ;
#10726=CARTESIAN_POINT ( 'NONE',  ( -16.96496224101209194, 1.652369717150043549, 20.34789198813115263 ) ) ;
#10729=CARTESIAN_POINT ( 'NONE',  ( -6.565451881449789973, 18.89189346177362694, 18.54958172136247896 ) ) ;
#10732=CARTESIAN_POINT ( 'NONE',  ( 19.61674503250824841, 3.986191100139169663, 6.041646659195333058 ) ) ;
#10733=CARTESIAN_POINT ( 'NONE',  ( 6.962021646281533194, 6.437683520590192998, 1.500000000000001332 ) ) ;
#10738=CARTESIAN_POINT ( 'NONE',  ( -19.92178149465837578, 1.957245511797581106, 18.50655187082627862 ) ) ;
#10739=CYLINDRICAL_SURFACE ( 'NONE', #27311, 20.00000000000000000 ) ;
#10742=EDGE_CURVE ( 'NONE', #12572, #7313, #8433, .T. ) ;
#10743=CARTESIAN_POINT ( 'NONE',  ( 10.62299781869221604, -13.36838230995976495, 18.92976555901915603 ) ) ;
#10746=ORIENTED_EDGE ( 'NONE', *, *, #2894, .F. ) ;
#10747=AXIS2_PLACEMENT_3D ( 'NONE', #2269, #11790, #20982 ) ;
#10751=CARTESIAN_POINT ( 'NONE',  ( -5.205279254987321025, 19.32936484843851233, 7.272049892295485485 ) ) ;
#10753=CARTESIAN_POINT ( 'NONE',  ( -12.86767874445213877, -1.850092897552710225, 1.500000000000001332 ) ) ;
#10754=AXIS2_PLACEMENT_3D ( 'NONE', #24006, #12494, #2344 ) ;
#10755=CARTESIAN_POINT ( 'NONE',  ( -12.73345385815986397, 11.29622791818862915, 6.910395520694543769 ) ) ;
#10760=CARTESIAN_POINT ( 'NONE',  ( 14.19710122452048928, 14.11195047426184246, 6.560937769032974209 ) ) ;
#10761=CARTESIAN_POINT ( 'NONE',  ( 19.82606750293204456, 2.764250834391624334, 5.749228751562096562 ) ) ;
#10764=VERTEX_POINT ( 'NONE', #2213 ) ;
#10766=B_SPLINE_CURVE_WITH_KNOTS ( 'NONE', 3,
 ( #8657, #3975, #48, #16728, #2546, #7383, #26089, #12061, #11745, #4879, #13788, #18934, #4421, #2388, #30608, #11594, #16273, #21088 ),
 .UNSPECIFIED., .F., .F.,
 ( 4, 2, 2, 2, 2, 2, 2, 2, 4 ),
 ( 0.000000000000000000, 0.0003967869494442891856, 0.0007935738988885783713, 0.001190360848332867611, 0.001587147797777156743, 0.001983934747221445874, 0.002380721696665735222, 0.002777508646110024137, 0.003174295595554313485 ),
 .UNSPECIFIED. ) ;
#10767=DIRECTION ( 'NONE',  ( -0.000000000000000000, -0.000000000000000000, -1.000000000000000000 ) ) ;
#10771=VERTEX_POINT ( 'NONE', #4863 ) ;
#10774=CARTESIAN_POINT ( 'NONE',  ( 0.000000000000000000, 0.000000000000000000, 1.500000000000001332 ) ) ;
#10777=CARTESIAN_POINT ( 'NONE',  ( 10.39222174957287415, -17.10906616942579817, 18.80699882434806369 ) ) ;
#10778=CARTESIAN_POINT ( 'NONE',  ( 16.87408724266513360, 2.240810012149824892, 19.66989035740801839 ) ) ;
#10780=CARTESIAN_POINT ( 'NONE',  ( -2.352830851074174223, -9.185733585337903406, 1.500000000000001332 ) ) ;
#10781=CARTESIAN_POINT ( 'NONE',  ( 17.99235278053350839, -8.774603096602954011, 6.111214848085761986 ) ) ;
#10782=CARTESIAN_POINT ( 'NONE',  ( -13.95039892200172638, 9.845341970609696958, 19.79423548914561692 ) ) ;
#10783=VECTOR ( 'NONE', #9773, 1000.000000000000114 ) ;
#10785=VERTEX_POINT ( 'NONE', #17176 ) ;
#10790=CARTESIAN_POINT ( 'NONE',  ( -5.364573742045090299, 19.28565133533679088, 20.12545155307891065 ) ) ;
#10794=AXIS2_PLACEMENT_3D ( 'NONE', #883, #24119, #19921 ) ;
#10796=ORIENTED_EDGE ( 'NONE', *, *, #20599, .F. ) ;
#10799=CARTESIAN_POINT ( 'NONE',  ( 0.000000000000000000, 0.000000000000000000, 1.500000000000001332 ) ) ;
#10801=LINE ( 'NONE', #22483, #9714 ) ;
#10803=EDGE_LOOP ( 'NONE', ( #21642, #20968 ) ) ;
#10809=ORIENTED_EDGE ( 'NONE', *, *, #25773, .T. ) ;
#10813=CYLINDRICAL_SURFACE ( 'NONE', #25942, 0.7500000000000006661 ) ;
#10825=CARTESIAN_POINT ( 'NONE',  ( -11.19021577446867255, -16.59822551944401781, 18.71435384576123440 ) ) ;
#10826=CARTESIAN_POINT ( 'NONE',  ( -14.77756128048223694, -8.549967187541071212, 7.196036389296800451 ) ) ;
#10828=CARTESIAN_POINT ( 'NONE',  ( 11.90564931213029354, -16.09225693709294802, 6.341840715582230281 ) ) ;
#10834=EDGE_LOOP ( 'NONE', ( #13289, #10746 ) ) ;
#10837=CARTESIAN_POINT ( 'NONE',  ( -15.07239450771860056, 13.17334274624126067, 5.749228751562096562 ) ) ;
#10838=AXIS2_PLACEMENT_3D ( 'NONE', #7817, #26389, #14829 ) ;
#10840=ORIENTED_EDGE ( 'NONE', *, *, #13837, .F. ) ;
#10841=CARTESIAN_POINT ( 'NONE',  ( 3.188743458493628502, 16.77324615163092858, 6.147510495896841398 ) ) ;
#10844=CARTESIAN_POINT ( 'NONE',  ( -9.400432693290859731, -14.18986588558385620, 6.641371103590088865 ) ) ;
#10851=VECTOR ( 'NONE', #10682, 1000.000000000000114 ) ;
#10856=CARTESIAN_POINT ( 'NONE',  ( 13.00948632770055546, 10.97642674697629062, 19.47784884541372818 ) ) ;
#10857=CARTESIAN_POINT ( 'NONE',  ( 16.12090643789933253, -5.615848544355930727, 7.269896094239230777 ) ) ;
#10859=AXIS2_PLACEMENT_3D ( 'NONE', #2273, #11794, #30820 ) ;
#10860=CARTESIAN_POINT ( 'NONE',  ( -16.96496224101209194, 1.652369717150044659, 7.652108011868850923 ) ) ;
#10861=AXIS2_PLACEMENT_3D ( 'NONE', #28309, #23146, #11162 ) ;
#10863=DIRECTION ( 'NONE',  ( 1.000000000000000000, 0.000000000000000000, 0.000000000000000000 ) ) ;
#10868=ORIENTED_EDGE ( 'NONE', *, *, #11872, .F. ) ;
#10869=ORIENTED_EDGE ( 'NONE', *, *, #29608, .F. ) ;
#10878=CARTESIAN_POINT ( 'NONE',  ( 9.340794358644611606, -14.23940931090254125, 20.14907003336613300 ) ) ;
#10880=ORIENTED_EDGE ( 'NONE', *, *, #28486, .T. ) ;
#10881=CARTESIAN_POINT ( 'NONE',  ( -10.94312936609104270, -16.74105124841231529, 20.22277707861862339 ) ) ;
#10884=CARTESIAN_POINT ( 'NONE',  ( 15.40940123050674693, 12.74987339073084058, 7.267242832833945343 ) ) ;
#10887=ORIENTED_EDGE ( 'NONE', *, *, #27904, .F. ) ;
#10888=CARTESIAN_POINT ( 'NONE',  ( -4.769904382750534744, 16.34378370244061429, 19.96344307082653202 ) ) ;
#10889=ORIENTED_EDGE ( 'NONE', *, *, #20194, .F. ) ;
#10897=DIRECTION ( 'NONE',  ( -0.9594929736144974797, -0.2817325568414297265, 0.000000000000000000 ) ) ;
#10898=B_SPLINE_SURFACE_WITH_KNOTS ( 'NONE', 3, 1, ( 
 ( #7151, #14305 ),
 ( #2472, #21481 ),
 ( #122, #20499 ),
 ( #29130, #12293 ),
 ( #13181, #22523 ),
 ( #17117, #27385 ),
 ( #5268, #15510 ),
 ( #25025, #26640 ),
 ( #8521, #27533 ),
 ( #30022, #2942 ),
 ( #3086, #13032 ),
 ( #5432, #1171 ),
 ( #579, #18170 ),
 ( #12461, #21798 ),
 ( #3667, #10844 ),
 ( #8353, #1323 ),
 ( #20184, #10678 ),
 ( #27678, #14935 ),
 ( #437, #24127 ),
 ( #9953, #6306 ),
 ( #19460, #18022 ),
 ( #24445, #19610 ),
 ( #17868, #7766 ),
 ( #28976, #7611 ),
 ( #15660, #22672 ),
 ( #14774, #17273 ),
 ( #2779, #20351 ),
 ( #29880, #24293 ),
 ( #26806, #13341 ),
 ( #25173, #6154 ),
 ( #3818, #22838 ) ),
 .UNSPECIFIED., .F., .F., .F.,
 ( 4, 3, 3, 3, 3, 3, 3, 3, 3, 3, 4 ),
 ( 2, 2 ),
 ( 0.000000000000000000, 0.05425176834609633791, 0.1085332949128352958, 0.1623767749169382768, 0.2157504826133063158, 0.2688657508888171455, 0.3218907763505476360, 0.3749548578363336993, 0.4282048033836242107, 0.4818374082110501444, 0.4999999999131654604 ),
 ( 0.000000000000000000, 1.000000000000000000 ),
 .UNSPECIFIED. ) ;
#10899=CARTESIAN_POINT ( 'NONE',  ( 16.74250592927945647, 3.198927888044585721, 5.652196082364320695 ) ) ;
#10900=LINE ( 'NONE', #22577, #12130 ) ;
#10901=VECTOR ( 'NONE', #28763, 1000.000000000000000 ) ;
#10905=CARTESIAN_POINT ( 'NONE',  ( 1.795426799894640935, -16.98366215210794294, 6.588756557121054236 ) ) ;
#10910=CARTESIAN_POINT ( 'NONE',  ( 11.93399590641349484, -16.07127689286907568, 19.14333282897057842 ) ) ;
#10914=VERTEX_POINT ( 'NONE', #17808 ) ;
#10918=CARTESIAN_POINT ( 'NONE',  ( -5.216068956281040059, 19.32652695433949930, 6.018569869498933578 ) ) ;
#10919=ORIENTED_EDGE ( 'NONE', *, *, #2531, .T. ) ;
#10920=PLANE ( 'NONE',  #27570 ) ;
#10926=EDGE_CURVE ( 'NONE', #30839, #12572, #14678, .T. ) ;
#10928=AXIS2_PLACEMENT_3D ( 'NONE', #2881, #12405, #26271 ) ;
#10932=ORIENTED_EDGE ( 'NONE', *, *, #20024, .F. ) ;
#10934=CARTESIAN_POINT ( 'NONE',  ( -14.00715867683253357, 9.770345079983769665, 19.21769074125272780 ) ) ;
#10941=CARTESIAN_POINT ( 'NONE',  ( 4.330755352941445757, 19.54356050811955825, 6.447548852708279377 ) ) ;
#10944=VERTEX_POINT ( 'NONE', #5952 ) ;
#10946=CARTESIAN_POINT ( 'NONE',  ( 15.41296542101254552, 5.939519782021115191, -0.6213203435596476032 ) ) ;
#10947=CARTESIAN_POINT ( 'NONE',  ( 19.88727842228974652, 2.283828795636141162, 19.77662771831109367 ) ) ;
#10949=CARTESIAN_POINT ( 'NONE',  ( -16.83923888061477570, 2.503175730361749896, 19.87181966307587544 ) ) ;
#10950=CARTESIAN_POINT ( 'NONE',  ( 18.17321615974886129, -8.393345561651573306, 5.749228751562096562 ) ) ;
#10952=CARTESIAN_POINT ( 'NONE',  ( 5.089453839167152438, 19.35995229554825769, 20.32367522806703874 ) ) ;
#10954=ORIENTED_EDGE ( 'NONE', *, *, #22329, .T. ) ;
#10957=CARTESIAN_POINT ( 'NONE',  ( -4.573183673931448645, 16.39543396787672691, 19.45164628100866722 ) ) ;
#10958=FACE_OUTER_BOUND ( 'NONE', #9909, .T. ) ;
#10961=EDGE_CURVE ( 'NONE', #4691, #28054, #11093, .T. ) ;
#10962=CARTESIAN_POINT ( 'NONE',  ( 0.000000000000000000, 0.000000000000000000, 1.500000000000001332 ) ) ;
#10963=ORIENTED_EDGE ( 'NONE', *, *, #28970, .T. ) ;
#10965=AXIS2_PLACEMENT_3D ( 'NONE', #2736, #24398, #2582 ) ;
#10970=ORIENTED_EDGE ( 'NONE', *, *, #249, .T. ) ;
#10971=CARTESIAN_POINT ( 'NONE',  ( -19.82706496683076836, 2.627678016133613959, 7.652108011868850923 ) ) ;
#10973=VERTEX_POINT ( 'NONE', #3928 ) ;
#10974=CARTESIAN_POINT ( 'NONE',  ( -11.86767874445213167, -1.850092897552710225, 24.50000000000000000 ) ) ;
#10976=DIRECTION ( 'NONE',  ( -0.000000000000000000, 0.000000000000000000, -1.000000000000000000 ) ) ;
#10981=CARTESIAN_POINT ( 'NONE',  ( 1.303806812501129064, -19.97511938206332971, 6.995624166085161910 ) ) ;
#10982=CARTESIAN_POINT ( 'NONE',  ( -16.82262805706082531, 2.599658093664293457, 6.973843882838226094 ) ) ;
#10986=DIRECTION ( 'NONE',  ( 0.000000000000000000, 0.000000000000000000, 1.000000000000000000 ) ) ;
#10998=CIRCLE ( 'NONE', #26940, 0.7499999999999988898 ) ;
#11000=CARTESIAN_POINT ( 'NONE',  ( 7.562559277181973627, -5.881244434206257310, 21.50000000000000000 ) ) ;
#11003=CARTESIAN_POINT ( 'NONE',  ( 19.55539447853113799, 4.193631725790831766, 19.48477075383299351 ) ) ;
#11006=DIRECTION ( 'NONE',  ( 0.000000000000000000, 0.000000000000000000, 1.000000000000000000 ) ) ;
#11009=ORIENTED_EDGE ( 'NONE', *, *, #18721, .F. ) ;
#11010=CARTESIAN_POINT ( 'NONE',  ( 11.67912593704039637, 12.45929511323409855, 19.61324152429827095 ) ) ;
#11012=CARTESIAN_POINT ( 'NONE',  ( 0.9770435002939156233, -19.97634058022565995, 18.54958172136248251 ) ) ;
#11015=CARTESIAN_POINT ( 'NONE',  ( -6.974883619896829146, -5.687793815610328707, 1.500000000000001332 ) ) ;
#11017=LINE ( 'NONE', #15372, #27975 ) ;
#11019=CARTESIAN_POINT ( 'NONE',  ( 9.035144332694070357, -14.42607982873159678, 6.910395520694542881 ) ) ;
#11020=CARTESIAN_POINT ( 'NONE',  ( 0.000000000000000000, 0.000000000000000000, 1.500000000000001332 ) ) ;
#11023=VERTEX_POINT ( 'NONE', #10780 ) ;
#11027=CARTESIAN_POINT ( 'NONE',  ( 18.33599632111990374, -7.986941774664180649, 20.34789198813115263 ) ) ;
#11033=CARTESIAN_POINT ( 'NONE',  ( -19.72724879956886923, 3.398799651952292056, 6.211014596808754007 ) ) ;
#11042=CARTESIAN_POINT ( 'NONE',  ( -14.76516729829709007, -8.573104839208673056, 7.158811349119584833 ) ) ;
#11043=DIRECTION ( 'NONE',  ( 1.000000000000000000, 0.000000000000000000, 0.000000000000000000 ) ) ;
#11045=CARTESIAN_POINT ( 'NONE',  ( -6.933969404122160007, 18.75953273845654579, 19.48477075383299706 ) ) ;
#11048=CARTESIAN_POINT ( 'NONE',  ( 0.3493064693810319365, -20.01473674030432548, 7.652108011868850035 ) ) ;
#11049=CARTESIAN_POINT ( 'NONE',  ( -9.650234827617421018, -17.53789701089550590, 19.47783254395485031 ) ) ;
#11050=CARTESIAN_POINT ( 'NONE',  ( -17.02500080808232852, 1.126395502206346100, 18.45571264222803975 ) ) ;
#11051=CARTESIAN_POINT ( 'NONE',  ( -19.95113275051131652, 1.631914050426796381, 18.82680253904184298 ) ) ;
#11053=ORIENTED_EDGE ( 'NONE', *, *, #590, .T. ) ;
#11061=CARTESIAN_POINT ( 'NONE',  ( -4.163336342344337027E-14, 1.387778780781445676E-14, 24.50000000000000000 ) ) ;
#11062=ADVANCED_FACE ( 'NONE', ( #15759 ), #912, .T. ) ;
#11063=CARTESIAN_POINT ( 'NONE',  ( -4.581181804672376678, 16.39335237280002033, 6.530762810602277924 ) ) ;
#11066=CARTESIAN_POINT ( 'NONE',  ( -13.38160118231794549, 10.55829203257430038, 5.652196082368482699 ) ) ;
#11071=CARTESIAN_POINT ( 'NONE',  ( -8.478038329015333829, 15.04174200911163517, 24.50000000000000000 ) ) ;
#11072=ORIENTED_EDGE ( 'NONE', *, *, #11683, .F. ) ;
#11074=CARTESIAN_POINT ( 'NONE',  ( 12.40635649856746525, 11.68570839673119544, 5.653912893140659257 ) ) ;
#11075=ORIENTED_EDGE ( 'NONE', *, *, #14735, .F. ) ;
#11076=CARTESIAN_POINT ( 'NONE',  ( -13.93282946020425328, 9.868441342995359022, 18.84329447212443753 ) ) ;
#11079=ORIENTED_EDGE ( 'NONE', *, *, #18723, .F. ) ;
#11080=CARTESIAN_POINT ( 'NONE',  ( 3.283642163210882092, 16.75135354181592007, 7.280727868105637768 ) ) ;
#11082=CARTESIAN_POINT ( 'NONE',  ( 5.780652116621848968, 19.14677724775279088, 18.47110296274025387 ) ) ;
#11083=EDGE_LOOP ( 'NONE', ( #14442, #5664, #23489, #25449 ) ) ;
#11085=AXIS2_PLACEMENT_3D ( 'NONE', #17941, #27450, #23618 ) ;
#11088=CARTESIAN_POINT ( 'NONE',  ( 16.84609478243854852, 2.477959627222519057, 20.05479082170252525 ) ) ;
#11091=ADVANCED_FACE ( 'NONE', ( #21182 ), #15882, .T. ) ;
#11093=LINE ( 'NONE', #13449, #296 ) ;
#11094=CARTESIAN_POINT ( 'NONE',  ( 15.43168774359948969, -7.187270164670358952, 6.211014596808754007 ) ) ;
#11095=CARTESIAN_POINT ( 'NONE',  ( -15.35487439336962723, 12.84287527963943809, 20.34789198813115263 ) ) ;
#11096=CARTESIAN_POINT ( 'NONE',  ( 4.678038002344203861, 19.46363151887951659, 18.56793045041961321 ) ) ;
#11098=ORIENTED_EDGE ( 'NONE', *, *, #366, .F. ) ;
#11102=ADVANCED_FACE ( 'NONE', ( #28853 ), #11153, .T. ) ;
#11103=CARTESIAN_POINT ( 'NONE',  ( -5.435829780283180312, 16.15227280059887605, 20.34789198813115263 ) ) ;
#11106=EDGE_CURVE ( 'NONE', #25827, #25672, #28859, .T. ) ;
#11107=DIRECTION ( 'NONE',  ( 1.000000000000000000, 0.000000000000000000, 0.000000000000000000 ) ) ;
#11109=EDGE_CURVE ( 'NONE', #22249, #24431, #21515, .T. ) ;
#11111=CARTESIAN_POINT ( 'NONE',  ( -16.97424920726489717, 1.578583718960129945, 7.652108011868850035 ) ) ;
#11115=ORIENTED_EDGE ( 'NONE', *, *, #30760, .T. ) ;
#11118=CARTESIAN_POINT ( 'NONE',  ( -19.84404562991029763, 2.492760124447686465, 5.652196082369965069 ) ) ;
#11119=CIRCLE ( 'NONE', #7125, 9.482273699623480212 ) ;
#11120=CARTESIAN_POINT ( 'NONE',  ( -19.87571927687822892, 2.229464111918812552, 18.37545668562167478 ) ) ;
#11121=ORIENTED_EDGE ( 'NONE', *, *, #13206, .T. ) ;
#11122=LINE ( 'NONE', #29994, #16286 ) ;
#11125=CARTESIAN_POINT ( 'NONE',  ( 16.09518941752841670, 6.251081041772567737, 24.50000000000000000 ) ) ;
#11127=CARTESIAN_POINT ( 'NONE',  ( 10.47960520055065992, -7.757439966934453146, 1.500000000000001332 ) ) ;
#11137=CARTESIAN_POINT ( 'NONE',  ( -17.91073422896668177, -8.940227287121107480, 18.39992786714538298 ) ) ;
#11138=EDGE_CURVE ( 'NONE', #24968, #19771, #27698, .T. ) ;
#11139=CIRCLE ( 'NONE', #5656, 0.7500000000000006661 ) ;
#11143=FACE_OUTER_BOUND ( 'NONE', #5922, .T. ) ;
#11146=EDGE_CURVE ( 'NONE', #13891, #203, #14225, .T. ) ;
#11149=CARTESIAN_POINT ( 'NONE',  ( 15.91781874855163004, -6.122627424427364851, 20.34789198813115263 ) ) ;
#11151=DIRECTION ( 'NONE',  ( -0.000000000000000000, -0.000000000000000000, 1.000000000000000000 ) ) ;
#11153=B_SPLINE_SURFACE_WITH_KNOTS ( 'NONE', 3, 1, ( 
 ( #17612, #9980 ),
 ( #17138, #24314 ),
 ( #2964, #10119 ),
 ( #10270, #19626 ),
 ( #3112, #12632 ),
 ( #22121, #19783 ),
 ( #7955, #25612 ),
 ( #26055, #16232 ),
 ( #4534, #21198 ),
 ( #13748, #30579 ),
 ( #14190, #30728 ),
 ( #9374, #16389 ),
 ( #18894, #25904 ),
 ( #27951, #11252 ),
 ( #23546, #8929 ),
 ( #6580, #11564 ),
 ( #16091, #4226 ),
 ( #2039, #30432 ),
 ( #23242, #1893 ),
 ( #7028, #6875 ),
 ( #11419, #14042 ),
 ( #28404, #2193 ),
 ( #6721, #20751 ),
 ( #9217, #25461 ),
 ( #8757, #30281 ),
 ( #4382, #16537 ),
 ( #11711, #18448 ),
 ( #4688, #25753 ),
 ( #20607, #28245 ),
 ( #1603, #11111 ),
 ( #23404, #30127 ) ),
 .UNSPECIFIED., .F., .F., .F.,
 ( 4, 3, 3, 3, 3, 3, 3, 3, 3, 3, 4 ),
 ( 2, 2 ),
 ( 0.4999999998345684427, 0.5360336730431942698, 0.5907651151589017324, 0.6456034593241839481, 0.6998270958050443191, 0.7529536536315944995, 0.8052385063053264513, 0.8575343587103996246, 0.9106564858195047574, 0.9648414833209688624, 1.000000006602610014 ),
 ( 0.000000000000000000, 1.000000000000000000 ),
 .UNSPECIFIED. ) ;
#11155=CARTESIAN_POINT ( 'NONE',  ( 2.555255504830960867, -9.131494062835622927, 21.50000000000000000 ) ) ;
#11156=CARTESIAN_POINT ( 'NONE',  ( 19.69983030747900088, 3.454193845114029049, 20.32200205377523972 ) ) ;
#11158=CARTESIAN_POINT ( 'NONE',  ( 8.637616862297841536, -3.912171961291982747, 21.50000000000000000 ) ) ;
#11159=EDGE_CURVE ( 'NONE', #27228, #8044, #29696, .T. ) ;
#11162=DIRECTION ( 'NONE',  ( 1.000000000000000000, 0.000000000000000000, 0.000000000000000000 ) ) ;
#11165=CARTESIAN_POINT ( 'NONE',  ( 12.44336852771590962, 11.64466880974753416, 18.34727598691068096 ) ) ;
#11166=DIRECTION ( 'NONE',  ( 1.000000000000000000, 0.000000000000000000, 0.000000000000000000 ) ) ;
#11169=PLANE ( 'NONE',  #15310 ) ;
#11172=CARTESIAN_POINT ( 'NONE',  ( -6.187077094091591789, 11.47693674426096955, 1.500000000000001332 ) ) ;
#11175=ORIENTED_EDGE ( 'NONE', *, *, #4955, .T. ) ;
#11179=CARTESIAN_POINT ( 'NONE',  ( -7.869584159753960861, 10.39565510934976977, 1.500000000000001332 ) ) ;
#11185=CARTESIAN_POINT ( 'NONE',  ( -11.33743862782229250, -16.47619710613050970, 19.08232364404840098 ) ) ;
#11189=DIRECTION ( 'NONE',  ( -0.4154150130018972598, -0.9096319953545133341, 0.000000000000000000 ) ) ;
#11190=ORIENTED_EDGE ( 'NONE', *, *, #11504, .F. ) ;
#11193=ORIENTED_EDGE ( 'NONE', *, *, #13973, .F. ) ;
#11200=DIRECTION ( 'NONE',  ( 1.000000000000000000, 0.000000000000000000, 0.000000000000000000 ) ) ;
#11201=CARTESIAN_POINT ( 'NONE',  ( -19.95825857724417318, 1.540497788607360086, 19.03762469184452755 ) ) ;
#11209=CARTESIAN_POINT ( 'NONE',  ( 8.999114229549594057, -0.1262659238204522361, 1.500000000000001332 ) ) ;
#11210=CARTESIAN_POINT ( 'NONE',  ( -5.151082791877244382, 19.34385597943987989, 6.111214848085761986 ) ) ;
#11212=DIRECTION ( 'NONE',  ( 1.000000000000000000, 0.000000000000000000, 0.000000000000000000 ) ) ;
#11221=ORIENTED_EDGE ( 'NONE', *, *, #11867, .T. ) ;
#11226=CARTESIAN_POINT ( 'NONE',  ( -18.35575104603286078, -7.986347210076461423, 5.940635272151477686 ) ) ;
#11228=LINE ( 'NONE', #27316, #875 ) ;
#11233=CARTESIAN_POINT ( 'NONE',  ( 19.77948086832033425, 3.081792779576177033, 20.34789198813115263 ) ) ;
#11234=ORIENTED_EDGE ( 'NONE', *, *, #15708, .F. ) ;
#11236=CARTESIAN_POINT ( 'NONE',  ( -16.86183147812083760, 2.368508504629200484, 20.05479082170252525 ) ) ;
#11237=CARTESIAN_POINT ( 'NONE',  ( 17.99082164042340537, -8.777603813954270251, 7.176035686813569292 ) ) ;
#11238=CARTESIAN_POINT ( 'NONE',  ( -13.51981801095249835, 10.39108251695558316, 20.32367522806703874 ) ) ;
#11239=CARTESIAN_POINT ( 'NONE',  ( 5.159688198573267215, 19.34150021954530274, 20.33971507717571114 ) ) ;
#11240=VERTEX_POINT ( 'NONE', #17782 ) ;
#11245=CARTESIAN_POINT ( 'NONE',  ( -5.151082791877242606, 19.34385597943988344, 18.80699882434806369 ) ) ;
#11246=DIRECTION ( 'NONE',  ( -0.000000000000000000, -0.000000000000000000, 1.000000000000000000 ) ) ;
#11248=VECTOR ( 'NONE', #14483, 1000.000000000000114 ) ;
#11250=DIRECTION ( 'NONE',  ( 0.000000000000000000, 0.000000000000000000, 1.000000000000000000 ) ) ;
#11252=CARTESIAN_POINT ( 'NONE',  ( -17.06520330450695866, 0.6550632133703672144, 6.447548852708279377 ) ) ;
#11255=EDGE_LOOP ( 'NONE', ( #7759, #16311, #29229, #4696 ) ) ;
#11257=DIRECTION ( 'NONE',  ( -0.000000000000000000, -0.000000000000000000, 1.000000000000000000 ) ) ;
#11261=CARTESIAN_POINT ( 'NONE',  ( 18.48560952955220316, -7.681425967031917601, 5.704143890883081269 ) ) ;
#11274=CARTESIAN_POINT ( 'NONE',  ( 0.6820093937066838974, -20.00641896168558986, 7.603368798681074736 ) ) ;
#11276=EDGE_CURVE ( 'NONE', #29673, #13769, #22448, .T. ) ;
#11278=EDGE_CURVE ( 'NONE', #10066, #18622, #957, .T. ) ;
#11280=DIRECTION ( 'NONE',  ( -0.000000000000000000, -0.000000000000000000, 1.000000000000000000 ) ) ;
#11284=EDGE_CURVE ( 'NONE', #19542, #23909, #15426, .T. ) ;
#11285=CARTESIAN_POINT ( 'NONE',  ( -17.60607916434270237, -9.525343863633434438, 19.14333282897057842 ) ) ;
#11286=AXIS2_PLACEMENT_3D ( 'NONE', #13157, #22816, #1467 ) ;
#11291=LINE ( 'NONE', #23128, #1955 ) ;
#11294=LINE ( 'NONE', #20792, #8176 ) ;
#11296=B_SPLINE_CURVE_WITH_KNOTS ( 'NONE', 3,
 ( #16946, #29109, #21774, #12122, #24421, #2452, #26465, #23957, #17254, #9624, #413, #11803, #9770, #105, #5096, #19441, #28651, #14609 ),
 .UNSPECIFIED., .F., .F.,
 ( 4, 2, 2, 2, 2, 2, 2, 2, 4 ),
 ( 0.000000000000000000, 0.0003967869494442875051, 0.0007935738988885750102, 0.001190360848332862407, 0.001587147797777150020, 0.001983934747221437634, 0.002380721696665724814, 0.002777508646110012427, 0.003174295595554300041 ),
 .UNSPECIFIED. ) ;
#11297=CARTESIAN_POINT ( 'NONE',  ( -14.01114995435608179, 9.765040422203638215, 6.588756557121049795 ) ) ;
#11300=CIRCLE ( 'NONE', #28726, 0.7500000000000006661 ) ;
#11306=CARTESIAN_POINT ( 'NONE',  ( 19.56124041029250904, 4.166605025611204383, 19.61564845152807735 ) ) ;
#11312=AXIS2_PLACEMENT_3D ( 'NONE', #19413, #7411, #23608 ) ;
#11314=CYLINDRICAL_SURFACE ( 'NONE', #22296, 0.9999999999999983347 ) ;
#11316=CARTESIAN_POINT ( 'NONE',  ( 11.80353037513723713, 12.33292095759475338, 18.73314399819312115 ) ) ;
#11317=CARTESIAN_POINT ( 'NONE',  ( 16.55527708515956675, 4.194179076328800271, 6.588756557121050683 ) ) ;
#11319=EDGE_CURVE ( 'NONE', #16485, #11391, #3905, .T. ) ;
#11320=DIRECTION ( 'NONE',  ( 0.000000000000000000, 0.000000000000000000, -1.000000000000000000 ) ) ;
#11321=CIRCLE ( 'NONE', #19788, 9.482273699623480212 ) ;
#11328=CARTESIAN_POINT ( 'NONE',  ( -15.54251014615008941, -6.943938207015637687, 19.77662771831109367 ) ) ;
#11329=CARTESIAN_POINT ( 'NONE',  ( -8.658642353097244282, -14.67867993405429772, 18.34727598691068096 ) ) ;
#11335=CARTESIAN_POINT ( 'NONE',  ( -7.700393225236267902, -15.24241778594199737, 6.392658652357120275 ) ) ;
#11336=EDGE_CURVE ( 'NONE', #29934, #10944, #20202, .T. ) ;
#11342=CARTESIAN_POINT ( 'NONE',  ( 18.02181326450767784, -8.714141732420079833, 18.71435384576123440 ) ) ;
#11343=CARTESIAN_POINT ( 'NONE',  ( 9.118789845653434867, -14.37574228027166434, 18.83976166372255534 ) ) ;
#11346=CARTESIAN_POINT ( 'NONE',  ( -16.93638505691475871, 1.872096242067389227, 5.670038381137163519 ) ) ;
#11349=DIRECTION ( 'NONE',  ( 1.000000000000000000, 0.000000000000000000, 0.000000000000000000 ) ) ;
#11354=VECTOR ( 'NONE', #17957, 1000.000000000000114 ) ;
#11357=CIRCLE ( 'NONE', #26302, 9.482273699623480212 ) ;
#11362=CARTESIAN_POINT ( 'NONE',  ( 0.7788148816922453310, -17.02744011591805062, 7.652108011868850923 ) ) ;
#11365=CARTESIAN_POINT ( 'NONE',  ( -17.05632420042081776, 0.7692048344978460461, 18.84329447212444109 ) ) ;
#11366=DIRECTION ( 'NONE',  ( 0.000000000000000000, 0.000000000000000000, -1.000000000000000000 ) ) ;
#11370=AXIS2_PLACEMENT_3D ( 'NONE', #9769, #14454, #5095 ) ;
#11371=CARTESIAN_POINT ( 'NONE',  ( 10.30429258806635140, -13.59853737800766815, 20.19593175699879595 ) ) ;
#11373=ORIENTED_EDGE ( 'NONE', *, *, #3164, .T. ) ;
#11375=CARTESIAN_POINT ( 'NONE',  ( 0.000000000000000000, 0.000000000000000000, 21.50000000000000000 ) ) ;
#11376=EDGE_CURVE ( 'NONE', #8129, #28377, #12781, .T. ) ;
#11383=CARTESIAN_POINT ( 'NONE',  ( -15.34618562042307843, 12.82554431217322310, 18.34798005863227388 ) ) ;
#11384=LINE ( 'NONE', #13430, #19962 ) ;
#11391=VERTEX_POINT ( 'NONE', #16360 ) ;
#11393=ORIENTED_EDGE ( 'NONE', *, *, #19501, .T. ) ;
#11395=CARTESIAN_POINT ( 'NONE',  ( -18.04156136322729864, -8.631457789788587576, 5.652196082369963293 ) ) ;
#11402=CARTESIAN_POINT ( 'NONE',  ( 15.40685886292497386, -7.237730981567048083, 6.974106381145714018 ) ) ;
#11403=CARTESIAN_POINT ( 'NONE',  ( -15.98601489809224319, 12.04791232832105408, 6.782048567692550378 ) ) ;
#11404=CARTESIAN_POINT ( 'NONE',  ( 3.060137030613564235, 16.80197902060524484, 19.25672174529527325 ) ) ;
#11405=EDGE_LOOP ( 'NONE', ( #2862, #19933, #25941, #15651, #27631, #24934, #27079, #5451, #8321, #659, #2590, #14050, #7290, #15593, #7806, #14195, #7236, #28017, #11989, #20250, #9767, #8748, #14861, #11959, #25877, #2889, #2279, #5309, #8313, #15787, #30351, #30285, #8778, #5537, #17466, #30268, #20263, #13258, #29699, #9546, #12356, #28921, #14941, #2868, #12347, #22088, #16854, #25578, #2078, #10625, #23424, #15765, #2976, #13322, #7267, #8437, #28511, #17706, #17833, #7599, #133, #9187, #19536, #24547, #26616, #3716, #21084, #26179, #24583, #13905, #23017, #6225, #22681, #29519, #29476, #22059, #15747, #29058, #19107, #27067, #22011, #22089, #13599 ) ) ;
#11406=ORIENTED_EDGE ( 'NONE', *, *, #8081, .F. ) ;
#11408=CARTESIAN_POINT ( 'NONE',  ( -15.75339717617903545, 12.35099711776840081, 7.441806358946449151 ) ) ;
#11409=CARTESIAN_POINT ( 'NONE',  ( 10.69237140622465532, -13.31695822555149356, 6.783738457429053348 ) ) ;
#11410=B_SPLINE_SURFACE_WITH_KNOTS ( 'NONE', 3, 1, ( 
 ( #2728, #29081 ),
 ( #21736, #10053 ),
 ( #17065, #7874 ),
 ( #27052, #22047 ),
 ( #19877, #5524 ),
 ( #9734, #7410 ),
 ( #22205, #7722 ),
 ( #29394, #16918 ),
 ( #378, #26594 ),
 ( #8029, #15027 ),
 ( #19561, #24079 ),
 ( #5373, #24541 ),
 ( #3189, #17533 ),
 ( #14721, #14426 ),
 ( #684, #24230 ),
 ( #7563, #10201 ),
 ( #14880, #21901 ),
 ( #23929, #19709 ),
 ( #21588, #221 ),
 ( #19247, #26434 ),
 ( #5067, #9897 ),
 ( #19412, #28929 ),
 ( #2879, #529 ),
 ( #13016, #10512 ),
 ( #24694, #22824 ),
 ( #15495, #25012 ),
 ( #8507, #18009 ),
 ( #27518, #6137 ),
 ( #29541, #30008 ),
 ( #8645, #1005 ),
 ( #8179, #22969 ) ),
 .UNSPECIFIED., .F., .F., .F.,
 ( 4, 3, 3, 3, 3, 3, 3, 3, 3, 3, 4 ),
 ( 2, 2 ),
 ( 0.4999999998345681651, 0.5360336730431942698, 0.5907651151589017324, 0.6456034593241839481, 0.6998270958050443191, 0.7529536536315944995, 0.8052385063053264513, 0.8575343587103996246, 0.9106564858195047574, 0.9648414833209688624, 1.000000006602610014 ),
 ( 0.000000000000000000, 1.000000000000000000 ),
 .UNSPECIFIED. ) ;
#11411=CARTESIAN_POINT ( 'NONE',  ( 13.01350570279884700, 10.97146294988703907, 6.714907520933422802 ) ) ;
#11419=CARTESIAN_POINT ( 'NONE',  ( -19.94989956810792009, 1.646935350084929972, 7.196036389296800451 ) ) ;
#11422=CARTESIAN_POINT ( 'NONE',  ( 19.87646685382694756, 2.220054991963869462, 19.60917204426170457 ) ) ;
#11423=ORIENTED_EDGE ( 'NONE', *, *, #29576, .F. ) ;
#11443=DIRECTION ( 'NONE',  ( -0.000000000000000000, -0.000000000000000000, 1.000000000000000000 ) ) ;
#11444=CARTESIAN_POINT ( 'NONE',  ( -15.09693789817080223, -7.923486267757676060, 18.35718225375110180 ) ) ;
#11449=DIRECTION ( 'NONE',  ( 1.000000000000000000, 0.000000000000000000, 0.000000000000000000 ) ) ;
#11452=EDGE_CURVE ( 'NONE', #22188, #154, #9275, .T. ) ;
#11454=ORIENTED_EDGE ( 'NONE', *, *, #7084, .T. ) ;
#11455=LINE ( 'NONE', #24199, #22614 ) ;
#11465=CARTESIAN_POINT ( 'NONE',  ( 17.75446986341059841, 9.207540381081344094, 1.500000000000001332 ) ) ;
#11466=VECTOR ( 'NONE', #18654, 1000.000000000000227 ) ;
#11470=CARTESIAN_POINT ( 'NONE',  ( 11.75175153055562838, 12.38566219040472305, 19.85459532544248162 ) ) ;
#11471=CARTESIAN_POINT ( 'NONE',  ( 12.35522425158188931, 11.74279415389956327, 18.34798005863078885 ) ) ;
#11472=DIRECTION ( 'NONE',  ( 0.000000000000000000, 0.000000000000000000, 1.000000000000000000 ) ) ;
#11473=CARTESIAN_POINT ( 'NONE',  ( -15.13937296497744178, 13.09668952202109438, 18.39701043959520987 ) ) ;
#11476=CARTESIAN_POINT ( 'NONE',  ( -12.85122823560700134, 11.16779817461281432, 18.72771030977187579 ) ) ;
#11481=EDGE_CURVE ( 'NONE', #16205, #16378, #10621, .T. ) ;
#11482=CARTESIAN_POINT ( 'NONE',  ( -15.49606647121365555, -7.052879176030717900, 19.96783386855779341 ) ) ;
#11486=ORIENTED_EDGE ( 'NONE', *, *, #18356, .T. ) ;
#11487=CARTESIAN_POINT ( 'NONE',  ( 0.9307681286968548795, -9.436481611552755666, 13.00000000000000178 ) ) ;
#11488=CARTESIAN_POINT ( 'NONE',  ( -7.677470532978346363, -15.25505107809155980, 6.521906765011493690 ) ) ;
#11491=ORIENTED_EDGE ( 'NONE', *, *, #8476, .T. ) ;
#11493=CARTESIAN_POINT ( 'NONE',  ( 18.13085077595199834, -8.485104792618541225, 18.49267272388512140 ) ) ;
#11494=CARTESIAN_POINT ( 'NONE',  ( 5.828790066614889298, 19.15065750257362609, 7.500898271101006820 ) ) ;
#11496=ADVANCED_FACE ( 'NONE', ( #28374 ), #15092, .T. ) ;
#11498=CARTESIAN_POINT ( 'NONE',  ( 6.187077094091595342, 11.47693674426096599, 1.500000000000001332 ) ) ;
#11499=CARTESIAN_POINT ( 'NONE',  ( 11.75961732103506385, 12.37772240090666642, 6.131018562779544823 ) ) ;
#11502=ORIENTED_EDGE ( 'NONE', *, *, #30168, .T. ) ;
#11503=DIRECTION ( 'NONE',  ( 0.000000000000000000, 0.000000000000000000, -1.000000000000000000 ) ) ;
#11504=EDGE_CURVE ( 'NONE', #9025, #9060, #23706, .T. ) ;
#11507=CARTESIAN_POINT ( 'NONE',  ( -15.26094448139683202, 12.92753815214665103, 5.651480102388686255 ) ) ;
#11514=CARTESIAN_POINT ( 'NONE',  ( 0.5496282100021196992, -17.03044801512709938, 7.632642797338977658 ) ) ;
#11516=LINE ( 'NONE', #28503, #21987 ) ;
#11520=EDGE_CURVE ( 'NONE', #30839, #24164, #896, .T. ) ;
#11521=EDGE_CURVE ( 'NONE', #17261, #7784, #20226, .T. ) ;
#11522=CARTESIAN_POINT ( 'NONE',  ( -6.481689221553158298, 15.79948487157344772, 6.917457548096559883 ) ) ;
#11527=CARTESIAN_POINT ( 'NONE',  ( 4.437794406404234060, 19.50150518896417751, 19.85730954408918336 ) ) ;
#11534=CARTESIAN_POINT ( 'NONE',  ( -15.89797731339009523, 12.13494807016274635, 18.84486140012300837 ) ) ;
#11536=ORIENTED_EDGE ( 'NONE', *, *, #4028, .T. ) ;
#11537=ORIENTED_EDGE ( 'NONE', *, *, #19501, .F. ) ;
#11540=ORIENTED_EDGE ( 'NONE', *, *, #12204, .F. ) ;
#11546=DIRECTION ( 'NONE',  ( -0.000000000000000000, -0.000000000000000000, 1.000000000000000000 ) ) ;
#11548=CARTESIAN_POINT ( 'NONE',  ( 16.87335920545513801, 2.247671665613721004, 19.00652017443069752 ) ) ;
#11550=CARTESIAN_POINT ( 'NONE',  ( 9.252152043196041120, -14.29436518012015256, 7.359006845440219102 ) ) ;
#11552=CARTESIAN_POINT ( 'NONE',  ( -15.70110224921264930, 12.41706793386161323, 5.810767894563978686 ) ) ;
#11553=CARTESIAN_POINT ( 'NONE',  ( 3.352743984114606057, 16.73528478182340962, 20.06253562465620632 ) ) ;
#11558=CARTESIAN_POINT ( 'NONE',  ( -5.031059497539946079, 16.27164807758199672, 18.49267272388512140 ) ) ;
#11559=DIRECTION ( 'NONE',  ( 0.5406408174555974444, 0.8412535328311813165, 0.000000000000000000 ) ) ;
#11564=CARTESIAN_POINT ( 'NONE',  ( -17.06629068372215485, 0.6401188461407946173, 6.672349528511551497 ) ) ;
#11568=CARTESIAN_POINT ( 'NONE',  ( 18.65775367615955460, -7.252215724661030372, 6.041646659195333058 ) ) ;
#11570=ORIENTED_EDGE ( 'NONE', *, *, #45, .T. ) ;
#11574=DIRECTION ( 'NONE',  ( 0.000000000000000000, 0.000000000000000000, 1.000000000000000000 ) ) ;
#11575=FACE_OUTER_BOUND ( 'NONE', #28317, .T. ) ;
#11576=CARTESIAN_POINT ( 'NONE',  ( -6.393592071792286724, 18.96945647184856654, 20.25542030744407640 ) ) ;
#11579=DIRECTION ( 'NONE',  ( 0.9594929736144952592, -0.2817325568414371095, 0.000000000000000000 ) ) ;
#11581=CARTESIAN_POINT ( 'NONE',  ( 15.55762523212740689, -6.926306048626145184, 5.848946451764560628 ) ) ;
#11582=DIRECTION ( 'NONE',  ( 1.000000000000000000, 0.000000000000000000, 0.000000000000000000 ) ) ;
#11584=ORIENTED_EDGE ( 'NONE', *, *, #25747, .T. ) ;
#11586=CARTESIAN_POINT ( 'NONE',  ( 11.11463800144301750, -16.64861661464430043, 7.652108011868850035 ) ) ;
#11587=DIRECTION ( 'NONE',  ( 0.000000000000000000, 0.000000000000000000, -1.000000000000000000 ) ) ;
#11594=CARTESIAN_POINT ( 'NONE',  ( -6.222613296526849247, 19.00773140132665517, 7.626218077512939786 ) ) ;
#11595=VECTOR ( 'NONE', #10087, 1000.000000000000000 ) ;
#11599=FACE_BOUND ( 'NONE', #24599, .T. ) ;
#11605=CYLINDRICAL_SURFACE ( 'NONE', #22341, 0.7500000000000006661 ) ;
#11606=CARTESIAN_POINT ( 'NONE',  ( -10.39981488257415165, -17.10438141112844690, 7.643931100913408550 ) ) ;
#11608=CARTESIAN_POINT ( 'NONE',  ( 1.139261986572421614, -19.98520933375989728, 19.97651184436794125 ) ) ;
#11609=ORIENTED_EDGE ( 'NONE', *, *, #20455, .T. ) ;
#11612=ADVANCED_FACE ( 'NONE', ( #22876 ), #13538, .F. ) ;
#11613=DIRECTION ( 'NONE',  ( 0.000000000000000000, 0.000000000000000000, 1.000000000000000000 ) ) ;
#11616=EDGE_LOOP ( 'NONE', ( #3784, #6762, #22195, #23507 ) ) ;
#11618=AXIS2_PLACEMENT_3D ( 'NONE', #27057, #12407, #21904 ) ;
#11620=CARTESIAN_POINT ( 'NONE',  ( -15.27764744541513053, -7.543477926929822885, 20.32222155561918697 ) ) ;
#11621=CARTESIAN_POINT ( 'NONE',  ( -12.79952941388599896, 11.22436372989799125, 18.83976166372256245 ) ) ;
#11624=CARTESIAN_POINT ( 'NONE',  ( -18.37606348208443308, -7.894877446839454471, 18.72886616302736229 ) ) ;
#11625=CARTESIAN_POINT ( 'NONE',  ( -15.57452153527462535, -6.867569271111570117, 19.22654678686458141 ) ) ;
#11627=ORIENTED_EDGE ( 'NONE', *, *, #14133, .F. ) ;
#11632=ORIENTED_EDGE ( 'NONE', *, *, #22202, .F. ) ;
#11633=CARTESIAN_POINT ( 'NONE',  ( 15.71976421978570748, -6.574744378264570699, 20.32842677360128292 ) ) ;
#11634=CARTESIAN_POINT ( 'NONE',  ( 4.874170568648002799, 16.31160065975152307, 7.176035686813569292 ) ) ;
#11636=EDGE_LOOP ( 'NONE', ( #6577, #25246, #7102, #17987, #14295, #9520, #23695, #22183, #11632, #21537, #18251, #14921, #24602, #3262, #30238, #25832, #12078, #18611, #19345, #29958, #5732, #26137, #21633, #11115, #8788, #12048, #4498, #16155, #15538, #24092, #10557, #16078, #23549, #9093, #2596, #493, #14230, #22163, #6804, #24677, #22596, #19795, #2717, #24845, #2168, #14726, #27250, #1793, #15306, #27752, #11190, #17797, #20060, #12468, #29, #22343, #11502, #8140, #4892, #26663, #27875, #5661, #29604, #4736, #3120, #14148, #9566, #7110, #15980, #29119, #21389, #10796, #3137, #6508, #4004, #29904, #7003 ) ) ;
#11643=LINE ( 'NONE', #18667, #27293 ) ;
#11644=EDGE_CURVE ( 'NONE', #8908, #23909, #22715, .T. ) ;
#11647=CARTESIAN_POINT ( 'NONE',  ( -14.67655575066034856, 13.58671083542087921, 6.518927109361836614 ) ) ;
#11650=CARTESIAN_POINT ( 'NONE',  ( 12.72536390617885438, -2.839914339433650348, 1.500000000000001332 ) ) ;
#11654=CARTESIAN_POINT ( 'NONE',  ( -0.3742200966386526884, -20.01457288233325471, 7.359006845440219102 ) ) ;
#11658=CARTESIAN_POINT ( 'NONE',  ( -17.02496544227784270, 1.117683430491693386, 20.19593175699879595 ) ) ;
#11660=VERTEX_POINT ( 'NONE', #8552 ) ;
#11665=ORIENTED_EDGE ( 'NONE', *, *, #5417, .F. ) ;
#11673=ORIENTED_EDGE ( 'NONE', *, *, #17821, .T. ) ;
#11674=CARTESIAN_POINT ( 'NONE',  ( 8.430595340551260364, -4.340342926364983533, 13.00000000000000178 ) ) ;
#11675=CARTESIAN_POINT ( 'NONE',  ( -7.028330626922778990, 10.93629592680536788, 24.50000000000000000 ) ) ;
#11681=EDGE_CURVE ( 'NONE', #11902, #5590, #29204, .T. ) ;
#11682=ORIENTED_EDGE ( 'NONE', *, *, #9974, .F. ) ;
#11683=EDGE_CURVE ( 'NONE', #21119, #24968, #11767, .T. ) ;
#11688=CARTESIAN_POINT ( 'NONE',  ( -0.2301049870085050963, -17.01973991014545007, 19.21496526180055398 ) ) ;
#11690=CARTESIAN_POINT ( 'NONE',  ( 1.795304038745377362, -16.98367057141059888, 19.47952243369110548 ) ) ;
#11691=CARTESIAN_POINT ( 'NONE',  ( 19.89137488457043901, 2.247671665613721004, 19.00652017443069752 ) ) ;
#11693=EDGE_CURVE ( 'NONE', #28858, #154, #9425, .T. ) ;
#11696=CARTESIAN_POINT ( 'NONE',  ( -15.45023549775889116, 12.72816703665372096, 7.643931100913408550 ) ) ;
#11697=DIRECTION ( 'NONE',  ( 1.000000000000000000, 0.000000000000000000, 0.000000000000000000 ) ) ;
#11698=ORIENTED_EDGE ( 'NONE', *, *, #983, .F. ) ;
#11700=CIRCLE ( 'NONE', #7729, 0.7500000000000006661 ) ;
#11703=CARTESIAN_POINT ( 'NONE',  ( 15.45664188325222455, 12.69231265181875834, 19.85261563089510517 ) ) ;
#11704=CARTESIAN_POINT ( 'NONE',  ( -5.549074438707200407, 16.11683645443577362, 18.34798005862930381 ) ) ;
#11707=DIRECTION ( 'NONE',  ( 0.000000000000000000, 0.000000000000000000, -1.000000000000000000 ) ) ;
#11711=CARTESIAN_POINT ( 'NONE',  ( -19.89984252009588062, 2.172142757504855304, 7.603368798681074736 ) ) ;
#11713=DIRECTION ( 'NONE',  ( 0.000000000000000000, 0.000000000000000000, -1.000000000000000000 ) ) ;
#11714=EDGE_LOOP ( 'NONE', ( #2613, #8184, #25914, #20103 ) ) ;
#11715=DIRECTION ( 'NONE',  ( -0.000000000000000000, -0.000000000000000000, 1.000000000000000000 ) ) ;
#11718=LINE ( 'NONE', #23707, #5064 ) ;
#11723=CARTESIAN_POINT ( 'NONE',  ( 9.864937699929956949, -13.90063973435163724, 18.34798005863078885 ) ) ;
#11725=CARTESIAN_POINT ( 'NONE',  ( -5.964083977939224290, 15.98216206238707926, 20.25542030744407640 ) ) ;
#11728=CARTESIAN_POINT ( 'NONE',  ( 1.000000000000008438, 17.23749217771910480, -0.6213203435596476032 ) ) ;
#11729=ORIENTED_EDGE ( 'NONE', *, *, #9965, .T. ) ;
#11736=CARTESIAN_POINT ( 'NONE',  ( -17.82234029294485467, -9.114408740892777416, 20.19593175699879595 ) ) ;
#11737=CARTESIAN_POINT ( 'NONE',  ( 19.74328841314636307, 3.194145055459935101, 7.652108011868850035 ) ) ;
#11740=ORIENTED_EDGE ( 'NONE', *, *, #1567, .T. ) ;
#11742=VECTOR ( 'NONE', #7208, 1000.000000000000000 ) ;
#11745=CARTESIAN_POINT ( 'NONE',  ( -6.934930584103121909, 18.75917743548997763, 6.523620417364445423 ) ) ;
#11750=DIRECTION ( 'NONE',  ( -0.000000000000000000, -0.000000000000000000, -1.000000000000000000 ) ) ;
#11755=ORIENTED_EDGE ( 'NONE', *, *, #21277, .F. ) ;
#11756=CARTESIAN_POINT ( 'NONE',  ( 0.01636335959932410516, -20.01808238691632624, 18.39701043959520987 ) ) ;
#11757=CARTESIAN_POINT ( 'NONE',  ( -8.487288213245035351, -14.78455279991285920, 7.652108011868850035 ) ) ;
#11759=CARTESIAN_POINT ( 'NONE',  ( 1.497940275966472390, -17.00196529467651985, 20.06253562465620632 ) ) ;
#11760=ORIENTED_EDGE ( 'NONE', *, *, #25744, .F. ) ;
#11764=CARTESIAN_POINT ( 'NONE',  ( 14.79201625507351991, 13.48748956535167665, 18.35718225375110180 ) ) ;
#11765=CARTESIAN_POINT ( 'NONE',  ( -5.524309650260710747, 7.706848733601013635, 21.50000000000000000 ) ) ;
#11767=CIRCLE ( 'NONE', #23218, 0.7499999999999988898 ) ;
#11769=CARTESIAN_POINT ( 'NONE',  ( -12.71197447203568132, 11.31946111510424302, 19.21496526180054332 ) ) ;
#11771=CARTESIAN_POINT ( 'NONE',  ( -19.94482228061659512, 1.484609193405912464, 6.523620417364436541 ) ) ;
#11773=CARTESIAN_POINT ( 'NONE',  ( -15.43012792948217182, -7.204331193346493301, 20.12545155307891065 ) ) ;
#11776=ORIENTED_EDGE ( 'NONE', *, *, #16255, .F. ) ;
#11777=ORIENTED_EDGE ( 'NONE', *, *, #14308, .F. ) ;
#11780=DIRECTION ( 'NONE',  ( 0.9096319953545183301, 0.4154150130018865461, 0.000000000000000000 ) ) ;
#11784=CARTESIAN_POINT ( 'NONE',  ( 15.39622458953737372, -7.259188434806183921, 19.56050940960062690 ) ) ;
#11785=CARTESIAN_POINT ( 'NONE',  ( 4.564720541824407007, 16.40857754966928894, 5.796888747622817029 ) ) ;
#11788=CARTESIAN_POINT ( 'NONE',  ( 4.049916830765389442, 16.55712665160098851, 20.34789198813115263 ) ) ;
#11790=DIRECTION ( 'NONE',  ( -0.000000000000000000, -0.000000000000000000, 1.000000000000000000 ) ) ;
#11794=DIRECTION ( 'NONE',  ( -0.6548607339452851006, -0.7557495743542582689, 0.000000000000000000 ) ) ;
#11797=CARTESIAN_POINT ( 'NONE',  ( -14.81512577538153153, 13.43580467474268758, 6.033082186765052590 ) ) ;
#11799=ORIENTED_EDGE ( 'NONE', *, *, #7531, .T. ) ;
#11800=CARTESIAN_POINT ( 'NONE',  ( -18.47028637364415360, -7.717842544976232233, 6.530762810602277924 ) ) ;
#11803=CARTESIAN_POINT ( 'NONE',  ( 14.27661992934221402, 14.00645734016344157, 7.161525567826881655 ) ) ;
#11805=CIRCLE ( 'NONE', #23746, 9.482273699623480212 ) ;
#11806=DIRECTION ( 'NONE',  ( -0.000000000000000000, -0.000000000000000000, 1.000000000000000000 ) ) ;
#11809=CARTESIAN_POINT ( 'NONE',  ( -19.87001189204712759, 2.428856360474549003, 20.34789198813115263 ) ) ;
#11812=CARTESIAN_POINT ( 'NONE',  ( 11.76322808224952610, -16.19669642467958326, 19.97651184436794125 ) ) ;
#11817=CARTESIAN_POINT ( 'NONE',  ( -15.73346977245381240, 12.34774510571039130, 7.454606537396343491 ) ) ;
#11818=CIRCLE ( 'NONE', #15804, 0.7500000000000006661 ) ;
#11820=LINE ( 'NONE', #30679, #23808 ) ;
#11824=EDGE_CURVE ( 'NONE', #27003, #14619, #2703, .T. ) ;
#11825=CARTESIAN_POINT ( 'NONE',  ( 15.25711736267466634, 12.95927645368826653, 20.19668224736330941 ) ) ;
#11827=CLOSED_SHELL ( 'NONE', ( #14809, #5735, #11612, #10528, #3833, #28222, #23864, #9567, #25661, #27330, #23649, #11091, #10306, #23428, #18585, #17573, #16090, #20848, #22882, #20434, #30714, #28064, #21959, #29797, #2342, #13762, #20484, #15901, #397, #11062, #30476, #1165, #24220, #13439, #9940, #25912, #28067, #24983, #22588, #9753, #17524, #18028, #18542, #7651, #27128, #10169, #13069, #8078, #13107, #30554, #16827, #11862, #12093, #1402, #17975, #23500, #7855, #16233, #13832, #28621, #21281, #16333, #24647, #21669, #1355, #13602, #12852, #27333, #14102, #7463, #13216, #586, #29113, #8054, #30004, #29829, #22703, #2339, #4043, #2954, #5403, #1822, #14531, #12037, #9790, #20045, #5273, #4427, #5516, #2314, #16824, #5061, #29115, #7504, #8815, #7319, #20744, #1900, #6013, #14287, #17798, #7684, #6931, #26513, #20955, #29441, #632, #22695, #15333, #28589, #22889, #16215, #23462, #13242, #10198, #15494, #11496, #25175, #1491, #10163, #30515, #25013, #19512, #28450, #7002, #3377, #12542, #4820, #21162, #20388, #22923, #9020, #3446, #3549, #25597, #9810, #26404, #17793, #8238, #5549, #20314, #11102, #11865, #28466, #1374, #16991, #18587, #18545, #6138, #12086, #30305, #4271, #15151, #26298, #9721, #3457, #9743, #8996, #28815, #3896, #16436, #21323, #25605, #21853, #6619, #1204, #25030, #22498, #16651, #20418, #19435, #17002, #15511, #1198, #19833, #21212, #13017, #19900, #14722, #30726, #19462, #3670, #595, #1055, #3676, #24432, #19897, #4990, #13358, #22364, #28838, #12315, #4784, #1020, #16989, #7647, #13929, #29940, #2754, #23463, #19236, #4838, #21539, #5169, #17237, #28283, #1769, #6886, #23646, #5700, #4530, #27541, #13916, #2906, #23925, #29421, #23665, #8278, #17950, #951, #5426, #12538, #12215, #7072, #5747, #17410, #7068, #13237, #21937, #23696, #198 ) ) ;
#11828=ORIENTED_EDGE ( 'NONE', *, *, #11276, .T. ) ;
#11832=CARTESIAN_POINT ( 'NONE',  ( 19.68435877536853695, 3.639270104310703857, 18.44527579819791185 ) ) ;
#11833=AXIS2_PLACEMENT_3D ( 'NONE', #6396, #27920, #26028 ) ;
#11836=CIRCLE ( 'NONE', #20301, 0.7500000000000006661 ) ;
#11837=CARTESIAN_POINT ( 'NONE',  ( 15.60425753233939616, -6.827323759874019515, 20.22273502201483808 ) ) ;
#11839=EDGE_CURVE ( 'NONE', #8702, #14537, #28754, .T. ) ;
#11847=CARTESIAN_POINT ( 'NONE',  ( 1.279633210264037979, -19.97671948047977963, 6.233981582756856987 ) ) ;
#11850=CARTESIAN_POINT ( 'NONE',  ( 16.83427080350347183, 2.570616772381428383, 18.55820869691756769 ) ) ;
#11852=CARTESIAN_POINT ( 'NONE',  ( -16.95590486909633299, 1.723587065725477263, 18.34969686940296185 ) ) ;
#11855=CARTESIAN_POINT ( 'NONE',  ( 0.7220001660362450613, 9.454746441592961403, 1.500000000000001332 ) ) ;
#11862=ADVANCED_FACE ( 'NONE', ( #10181, #29211, #7546 ), #10036, .T. ) ;
#11865=ADVANCED_FACE ( 'NONE', ( #14859 ), #5506, .T. ) ;
#11867=EDGE_CURVE ( 'NONE', #357, #10573, #9846, .T. ) ;
#11870=AXIS2_PLACEMENT_3D ( 'NONE', #13421, #27290, #5921 ) ;
#11872=EDGE_CURVE ( 'NONE', #6239, #14509, #22098, .T. ) ;
#11880=DIRECTION ( 'NONE',  ( 1.000000000000000000, 0.000000000000000000, 0.000000000000000000 ) ) ;
#11882=EDGE_CURVE ( 'NONE', #25305, #30087, #1826, .T. ) ;
#11886=VERTEX_POINT ( 'NONE', #20613 ) ;
#11889=CARTESIAN_POINT ( 'NONE',  ( 10.69247012765650062, -13.31688477309528196, 19.28454053338348473 ) ) ;
#11892=CARTESIAN_POINT ( 'NONE',  ( 10.99809977392671279, -16.70505906359367643, 20.34789198813115618 ) ) ;
#11894=EDGE_LOOP ( 'NONE', ( #15548, #3984, #10098, #6953 ) ) ;
#11902=VERTEX_POINT ( 'NONE', #3787 ) ;
#11903=DIRECTION ( 'NONE',  ( 1.000000000000000000, 0.000000000000000000, 0.000000000000000000 ) ) ;
#11904=CARTESIAN_POINT ( 'NONE',  ( -14.92657760816261359, -8.264136099378399436, 20.19593175699879595 ) ) ;
#11905=EDGE_CURVE ( 'NONE', #16299, #19910, #30134, .T. ) ;
#11907=EDGE_CURVE ( 'NONE', #30397, #26027, #3311, .T. ) ;
#11910=CIRCLE ( 'NONE', #7931, 10.00000000000000000 ) ;
#11912=DIRECTION ( 'NONE',  ( 1.000000000000000000, 0.000000000000000000, 0.000000000000000000 ) ) ;
#11913=CARTESIAN_POINT ( 'NONE',  ( -5.549075634136967139, 16.11684027513961226, 5.652196082368482699 ) ) ;
#11919=VERTEX_POINT ( 'NONE', #27810 ) ;
#11921=DIRECTION ( 'NONE',  ( 1.000000000000000000, 0.000000000000000000, 0.000000000000000000 ) ) ;
#11922=EDGE_LOOP ( 'NONE', ( #4309, #14742 ) ) ;
#11924=DIRECTION ( 'NONE',  ( 1.000000000000000000, 0.000000000000000000, 0.000000000000000000 ) ) ;
#11928=ORIENTED_EDGE ( 'NONE', *, *, #16398, .T. ) ;
#11929=CARTESIAN_POINT ( 'NONE',  ( 0.05528831664089212811, -17.02727625121208632, 20.05479082170252525 ) ) ;
#11930=CARTESIAN_POINT ( 'NONE',  ( -7.747355498299751453, -15.21644541356980440, 6.233981582756856987 ) ) ;
#11931=CARTESIAN_POINT ( 'NONE',  ( -2.959227181723746547, 8.499586724479465616, 1.500000000000001332 ) ) ;
#11932=AXIS2_PLACEMENT_3D ( 'NONE', #10962, #11250, #9214 ) ;
#11933=CARTESIAN_POINT ( 'NONE',  ( 1.745046693156364404, -16.98705356654485854, 19.03762469184452755 ) ) ;
#11937=CARTESIAN_POINT ( 'NONE',  ( 14.20032907733019911, 14.10870362182395077, 19.47783254395485031 ) ) ;
#11938=CARTESIAN_POINT ( 'NONE',  ( 1.000000000000008438, 13.00000000000001421, 1.500000000000001332 ) ) ;
#11939=ORIENTED_EDGE ( 'NONE', *, *, #16224, .T. ) ;
#11944=LINE ( 'NONE', #9589, #16759 ) ;
#11945=CARTESIAN_POINT ( 'NONE',  ( -12.71614549213777678, 11.31496011770029853, 19.47784884541372818 ) ) ;
#11950=ORIENTED_EDGE ( 'NONE', *, *, #10742, .T. ) ;
#11957=CARTESIAN_POINT ( 'NONE',  ( 18.30570112562006102, -8.101025642224000123, 20.34789198813115263 ) ) ;
#11958=FACE_OUTER_BOUND ( 'NONE', #2796, .T. ) ;
#11959=ORIENTED_EDGE ( 'NONE', *, *, #30141, .T. ) ;
#11960=CARTESIAN_POINT ( 'NONE',  ( 4.870982490315499014, 16.31268916845846206, 18.80699882434806369 ) ) ;
#11961=CARTESIAN_POINT ( 'NONE',  ( 12.06031594364852033, 12.06435167025952282, 7.559636331181775581 ) ) ;
#11969=VERTEX_POINT ( 'NONE', #20321 ) ;
#11970=CARTESIAN_POINT ( 'NONE',  ( -15.49172192819003691, -7.063155179282995633, 6.018569869498933578 ) ) ;
#11972=DIRECTION ( 'NONE',  ( -0.9898214418809326842, -0.1423148382732852824, 0.000000000000000000 ) ) ;
#11973=VECTOR ( 'NONE', #15312, 1000.000000000000000 ) ;
#11974=DIRECTION ( 'NONE',  ( -0.000000000000000000, -0.000000000000000000, 1.000000000000000000 ) ) ;
#11975=CARTESIAN_POINT ( 'NONE',  ( -17.06520330450695155, 0.6550632133703635507, 19.14333282897057842 ) ) ;
#11976=DIRECTION ( 'NONE',  ( -0.8412535328311884220, -0.5406408174555862312, 0.000000000000000000 ) ) ;
#11977=ORIENTED_EDGE ( 'NONE', *, *, #12771, .F. ) ;
#11980=ORIENTED_EDGE ( 'NONE', *, *, #25034, .F. ) ;
#11981=AXIS2_PLACEMENT_3D ( 'NONE', #25641, #21085, #4418 ) ;
#11983=CARTESIAN_POINT ( 'NONE',  ( 4.335955696074039523, 19.52440042691176458, 19.61564845152807735 ) ) ;
#11986=ORIENTED_EDGE ( 'NONE', *, *, #15917, .F. ) ;
#11989=ORIENTED_EDGE ( 'NONE', *, *, #20437, .F. ) ;
#11990=CARTESIAN_POINT ( 'NONE',  ( 16.09309408545196618, -5.686824080536027282, 18.64703902303423178 ) ) ;
#11991=CARTESIAN_POINT ( 'NONE',  ( -15.97601187733367922, 12.03191775062556346, 19.21940439362674624 ) ) ;
#12000=CARTESIAN_POINT ( 'NONE',  ( -17.67829152986845642, -9.353438168054491797, 6.037995405461185960 ) ) ;
#12004=EDGE_CURVE ( 'NONE', #12022, #26711, #26880, .T. ) ;
#12008=CIRCLE ( 'NONE', #2548, 1.000000000000010436 ) ;
#12010=DIRECTION ( 'NONE',  ( 0.000000000000000000, 0.000000000000000000, 1.000000000000000000 ) ) ;
#12012=CARTESIAN_POINT ( 'NONE',  ( -2.555255504830907132, 9.131494062835638914, 1.500000000000001332 ) ) ;
#12017=CARTESIAN_POINT ( 'NONE',  ( 18.39103589699442054, -7.860502636612779703, 18.34869673959211767 ) ) ;
#12018=CARTESIAN_POINT ( 'NONE',  ( -3.912171961292012057, -8.637616862297827325, 21.50000000000000000 ) ) ;
#12020=EDGE_CURVE ( 'NONE', #26415, #22510, #10647, .T. ) ;
#12022=VERTEX_POINT ( 'NONE', #8317 ) ;
#12024=CARTESIAN_POINT ( 'NONE',  ( -18.04156136322730219, -8.631457789788591128, 18.34798005863226678 ) ) ;
#12028=ORIENTED_EDGE ( 'NONE', *, *, #9993, .F. ) ;
#12029=FACE_BOUND ( 'NONE', #12466, .T. ) ;
#12030=EDGE_CURVE ( 'NONE', #6265, #24299, #9527, .T. ) ;
#12037=ADVANCED_FACE ( 'NONE', ( #2045 ), #16396, .F. ) ;
#12038=CARTESIAN_POINT ( 'NONE',  ( 9.860909914091285700, -13.90333503830274253, 20.34789198813115263 ) ) ;
#12042=ORIENTED_EDGE ( 'NONE', *, *, #10466, .F. ) ;
#12043=EDGE_CURVE ( 'NONE', #27530, #14763, #30585, .T. ) ;
#12048=ORIENTED_EDGE ( 'NONE', *, *, #4963, .T. ) ;
#12049=CARTESIAN_POINT ( 'NONE',  ( 2.703030265324084080, -12.75514121382991384, 1.500000000000001332 ) ) ;
#12050=CARTESIAN_POINT ( 'NONE',  ( -19.62935297797563905, -3.832558109936532009, 1.500000000000001332 ) ) ;
#12051=CYLINDRICAL_SURFACE ( 'NONE', #7765, 9.482273699623480212 ) ;
#12054=VECTOR ( 'NONE', #17878, 1000.000000000000000 ) ;
#12061=CARTESIAN_POINT ( 'NONE',  ( -6.910239377218537093, 18.76835738875812964, 6.392525840300343987 ) ) ;
#12066=ORIENTED_EDGE ( 'NONE', *, *, #1417, .F. ) ;
#12068=CARTESIAN_POINT ( 'NONE',  ( -10.39781135303995008, -17.08517550777068905, 5.652912763329821288 ) ) ;
#12073=CARTESIAN_POINT ( 'NONE',  ( -0.1765357775187695322, -17.02148976770177669, 19.00652017443069752 ) ) ;
#12074=EDGE_CURVE ( 'NONE', #21154, #17232, #27957, .T. ) ;
#12076=CARTESIAN_POINT ( 'NONE',  ( -10.33762405876901447, -17.14187335405548751, 7.627891251804737927 ) ) ;
#12077=LINE ( 'NONE', #10042, #24300 ) ;
#12078=ORIENTED_EDGE ( 'NONE', *, *, #8281, .F. ) ;
#12079=CARTESIAN_POINT ( 'NONE',  ( 18.33793066653144521, -7.982499537706466697, 5.652196082369965069 ) ) ;
#12080=B_SPLINE_CURVE_WITH_KNOTS ( 'NONE', 3,
 ( #15516, #13039, #10683, #29713, #1643, #22845, #1495, #8359, #30025, #11003, #11306, #17875, #3674, #30327, #13189, #11156, #30174, #20503 ),
 .UNSPECIFIED., .F., .F.,
 ( 4, 2, 2, 2, 2, 2, 2, 2, 4 ),
 ( 0.000000000000000000, 0.0003967869494442890772, 0.0007935738988885781544, 0.001190360848332867177, 0.001587147797777156309, 0.001983934747221445440, 0.002380721696665734355, 0.002777508646110023703, 0.003174295595554312618 ),
 .UNSPECIFIED. ) ;
#12083=CARTESIAN_POINT ( 'NONE',  ( 11.92830948316210105, 12.20365889974008944, 20.13759033520874908 ) ) ;
#12086=ADVANCED_FACE ( 'NONE', ( #2200 ), #1937, .T. ) ;
#12088=CARTESIAN_POINT ( 'NONE',  ( 7.730328572437743517, -4.608906612435629491, 1.500000000000001332 ) ) ;
#12089=CARTESIAN_POINT ( 'NONE',  ( 10.47960520055065992, -7.757439966934453146, 1.500000000000001332 ) ) ;
#12091=CARTESIAN_POINT ( 'NONE',  ( -19.84344116185557283, 2.497567387674354489, 7.652108011868850035 ) ) ;
#12092=DIRECTION ( 'NONE',  ( 1.000000000000000000, 0.000000000000000000, 0.000000000000000000 ) ) ;
#12093=ADVANCED_FACE ( 'NONE', ( #14518, #2820, #12029 ), #17159, .T. ) ;
#12096=DIRECTION ( 'NONE',  ( -0.000000000000000000, -0.000000000000000000, 1.000000000000000000 ) ) ;
#12097=VERTEX_POINT ( 'NONE', #24011 ) ;
#12098=ORIENTED_EDGE ( 'NONE', *, *, #16475, .F. ) ;
#12100=CARTESIAN_POINT ( 'NONE',  ( -5.488535287689155773, 19.23255048776056952, 18.47110296274025387 ) ) ;
#12102=CARTESIAN_POINT ( 'NONE',  ( 18.58529988941437949, 7.388276390372287672, 24.50000000000000000 ) ) ;
#12105=CARTESIAN_POINT ( 'NONE',  ( 16.19468640091380607, -5.422205736210270466, 19.47952243369110548 ) ) ;
#12106=CARTESIAN_POINT ( 'NONE',  ( 4.817555027346760887, 16.32979927342788784, 7.272049892295485485 ) ) ;
#12109=CARTESIAN_POINT ( 'NONE',  ( 4.874170568648001023, 16.31160065975151241, 19.87181966307587544 ) ) ;
#12110=CARTESIAN_POINT ( 'NONE',  ( 14.21537200517654576, 14.09360477215025931, 6.892848776733236704 ) ) ;
#12114=EDGE_LOOP ( 'NONE', ( #3393, #22028, #8268, #11193 ) ) ;
#12122=CARTESIAN_POINT ( 'NONE',  ( 14.53509801925589784, 13.73847344395387537, 5.779535427900759359 ) ) ;
#12123=CARTESIAN_POINT ( 'NONE',  ( -0.2311899301088659875, -17.01971842090038223, 6.755862304746362845 ) ) ;
#12124=DIRECTION ( 'NONE',  ( -0.000000000000000000, -0.000000000000000000, 1.000000000000000000 ) ) ;
#12128=ORIENTED_EDGE ( 'NONE', *, *, #20630, .T. ) ;
#12130=VECTOR ( 'NONE', #8097, 1000.000000000000000 ) ;
#12132=ORIENTED_EDGE ( 'NONE', *, *, #21025, .F. ) ;
#12135=CARTESIAN_POINT ( 'NONE',  ( -15.97539537256529840, 12.03273630363204738, 6.788986777570705122 ) ) ;
#12139=B_SPLINE_CURVE_WITH_KNOTS ( 'NONE', 3,
 ( #10656, #3028, #20014, #10192, #17676, #27195, #22040, #15326, #19700, #5517, #15019, #3495, #13008, #20165, #29686, #14527, #14205, #9852 ),
 .UNSPECIFIED., .F., .F.,
 ( 4, 2, 2, 2, 2, 2, 2, 2, 4 ),
 ( 0.003174295595554290066, 0.003570702171545513722, 0.003967108747536737812, 0.004363515323527961468, 0.004759921899519185123, 0.005156328475510408779, 0.005552735051501632435, 0.005949141627492856091, 0.006345548203484079747 ),
 .UNSPECIFIED. ) ;
#12142=CARTESIAN_POINT ( 'NONE',  ( 16.18939002998177301, -5.436351910499660711, 19.14333282897057842 ) ) ;
#12143=CARTESIAN_POINT ( 'NONE',  ( 19.61674503250825197, 3.986191100139168775, 18.73743063545763121 ) ) ;
#12148=VERTEX_POINT ( 'NONE', #29019 ) ;
#12153=CARTESIAN_POINT ( 'NONE',  ( -13.02230393242516371, 10.97666050933785797, 20.19668224736330941 ) ) ;
#12154=CARTESIAN_POINT ( 'NONE',  ( -7.995704773938816956, -15.07639970738306268, 18.56793045041961321 ) ) ;
#12159=CARTESIAN_POINT ( 'NONE',  ( -19.84673203616235071, 2.611426761413843778, 18.35377592296120497 ) ) ;
#12167=DIRECTION ( 'NONE',  ( -0.5406408174555976665, 0.8412535328311810945, 0.000000000000000000 ) ) ;
#12169=CARTESIAN_POINT ( 'NONE',  ( -4.863253556059215832, 16.31819504766686180, 18.63641924841378028 ) ) ;
#12170=CARTESIAN_POINT ( 'NONE',  ( 11.75175153053879384, 12.38566219042179206, 7.158811349119584833 ) ) ;
#12178=ORIENTED_EDGE ( 'NONE', *, *, #11284, .F. ) ;
#12179=CARTESIAN_POINT ( 'NONE',  ( 12.71820101047899421, 11.32761398983758383, 7.500898271101006820 ) ) ;
#12181=CARTESIAN_POINT ( 'NONE',  ( 18.71162862491809875, -7.111980085401802931, 6.995624166085161910 ) ) ;
#12182=CARTESIAN_POINT ( 'NONE',  ( 16.58239702338339683, 4.066005520117116134, 19.85459532544247452 ) ) ;
#12185=CARTESIAN_POINT ( 'NONE',  ( 18.58529988941437949, 7.388276390372287672, 24.50000000000000000 ) ) ;
#12191=CARTESIAN_POINT ( 'NONE',  ( 6.187077094091595342, 11.47693674426096599, 1.500000000000001332 ) ) ;
#12204=EDGE_CURVE ( 'NONE', #30019, #17362, #14303, .T. ) ;
#12205=CARTESIAN_POINT ( 'NONE',  ( 5.352643706120463030, 7.827050521741900191, 21.50000000000000000 ) ) ;
#12206=ORIENTED_EDGE ( 'NONE', *, *, #30686, .T. ) ;
#12208=ORIENTED_EDGE ( 'NONE', *, *, #7707, .F. ) ;
#12211=ORIENTED_EDGE ( 'NONE', *, *, #28513, .F. ) ;
#12214=CARTESIAN_POINT ( 'NONE',  ( -10.29013980557132690, -17.15015428632897709, 7.626218077512938009 ) ) ;
#12215=ADVANCED_FACE ( 'NONE', ( #20435 ), #1258, .F. ) ;
#12216=ORIENTED_EDGE ( 'NONE', *, *, #18187, .F. ) ;
#12217=VERTEX_POINT ( 'NONE', #20278 ) ;
#12218=CARTESIAN_POINT ( 'NONE',  ( -0.6368756358441500787, -20.00777098345650984, 19.56050940960062690 ) ) ;
#12221=CARTESIAN_POINT ( 'NONE',  ( -9.692246323650991258, -17.51472466453636656, 6.341840715582230281 ) ) ;
#12223=EDGE_CURVE ( 'NONE', #13757, #20446, #26383, .T. ) ;
#12224=CARTESIAN_POINT ( 'NONE',  ( 1.279633210264036425, -19.97671948047979029, 18.92976555901915603 ) ) ;
#12230=CARTESIAN_POINT ( 'NONE',  ( 0.4831130459764284568, -19.99459506363783490, 20.34789198813115263 ) ) ;
#12231=DIRECTION ( 'NONE',  ( 1.000000000000000000, 0.000000000000000000, 0.000000000000000000 ) ) ;
#12232=VERTEX_POINT ( 'NONE', #5937 ) ;
#12236=CIRCLE ( 'NONE', #5807, 9.482273699623480212 ) ;
#12238=CARTESIAN_POINT ( 'NONE',  ( -18.20229063954116455, -8.330696590476666330, 18.39701043959520987 ) ) ;
#12245=CARTESIAN_POINT ( 'NONE',  ( -15.06643696584252368, 13.18059642443756907, 7.557577766377196582 ) ) ;
#12256=CARTESIAN_POINT ( 'NONE',  ( 6.127899591227621734, 19.05688428395638923, 19.87181966307587544 ) ) ;
#12263=DIRECTION ( 'NONE',  ( -0.000000000000000000, -0.000000000000000000, 1.000000000000000000 ) ) ;
#12265=B_SPLINE_CURVE_WITH_KNOTS ( 'NONE', 3,
 ( #23176, #13990, #1532, #25849, #6361, #27579, #16330, #18668, #4481, #30214, #23027, #11042, #25688, #3870, #23487, #20400 ),
 .UNSPECIFIED., .F., .F.,
 ( 4, 2, 2, 2, 2, 2, 2, 4 ),
 ( 0.4999999999999999445, 0.6249999999999995559, 0.6874999999999994449, 0.7187499999999995559, 0.7499999999999997780, 0.8124999999999995559, 0.8749999999999993339, 1.000000000000000000 ),
 .UNSPECIFIED. ) ;
#12266=EDGE_CURVE ( 'NONE', #4819, #13119, #24366, .T. ) ;
#12271=CARTESIAN_POINT ( 'NONE',  ( -18.45502384974594889, -7.754294478968726700, 6.974106381145714018 ) ) ;
#12273=CARTESIAN_POINT ( 'NONE',  ( 1.000000000000008438, 13.00000000000001421, 1.500000000000001332 ) ) ;
#12274=CARTESIAN_POINT ( 'NONE',  ( 0.1486850733125486546, -17.02875910996195685, 5.862424720655265098 ) ) ;
#12280=ORIENTED_EDGE ( 'NONE', *, *, #1377, .T. ) ;
#12284=ORIENTED_EDGE ( 'NONE', *, *, #24998, .T. ) ;
#12289=AXIS2_PLACEMENT_3D ( 'NONE', #2918, #2762, #2605 ) ;
#12290=ORIENTED_EDGE ( 'NONE', *, *, #14908, .T. ) ;
#12293=CARTESIAN_POINT ( 'NONE',  ( -8.835414383224247103, -14.56605378991199551, 7.595116371587256054 ) ) ;
#12295=CARTESIAN_POINT ( 'NONE',  ( 16.16412758434836405, -5.502972621964707933, 18.92976555901915603 ) ) ;
#12296=CARTESIAN_POINT ( 'NONE',  ( 19.58625041283695367, 4.133291823432034384, 19.69140814234746273 ) ) ;
#12298=DIRECTION ( 'NONE',  ( 0.000000000000000000, 0.000000000000000000, 1.000000000000000000 ) ) ;
#12305=CIRCLE ( 'NONE', #16795, 0.7499999999999988898 ) ;
#12308=CARTESIAN_POINT ( 'NONE',  ( -6.505190245242044256, 15.79074656234091201, 19.47783254395485031 ) ) ;
#12309=CARTESIAN_POINT ( 'NONE',  ( -15.13676175850366334, 13.09931225869579308, 20.29090034784956131 ) ) ;
#12312=CARTESIAN_POINT ( 'NONE',  ( 0.000000000000000000, 0.000000000000000000, 1.500000000000001332 ) ) ;
#12313=DIRECTION ( 'NONE',  ( -0.8412535328311884220, -0.5406408174555862312, 0.000000000000000000 ) ) ;
#12315=ADVANCED_FACE ( 'NONE', ( #28063 ), #27923, .F. ) ;
#12318=CARTESIAN_POINT ( 'NONE',  ( -15.40257881337302592, 12.78582346615752741, 7.652108011868850035 ) ) ;
#12320=DIRECTION ( 'NONE',  ( 1.000000000000000000, 0.000000000000000000, 0.000000000000000000 ) ) ;
#12323=ORIENTED_EDGE ( 'NONE', *, *, #1622, .T. ) ;
#12324=CARTESIAN_POINT ( 'NONE',  ( 8.884323311075775109, 1.438332125858202692, 1.500000000000001332 ) ) ;
#12327=CARTESIAN_POINT ( 'NONE',  ( -4.935065328765587012, 16.29835470421561539, 7.429667576816606278 ) ) ;
#12331=AXIS2_PLACEMENT_3D ( 'NONE', #16244, #15633, #4095 ) ;
#12337=CARTESIAN_POINT ( 'NONE',  ( -17.68050765791476309, -9.349252870402535720, 19.96797677718664588 ) ) ;
#12339=ORIENTED_EDGE ( 'NONE', *, *, #24020, .F. ) ;
#12340=CARTESIAN_POINT ( 'NONE',  ( 15.49551216414738875, 12.67315350590407697, 7.080843742048788414 ) ) ;
#12342=CIRCLE ( 'NONE', #15329, 9.482273699623480212 ) ;
#12347=ORIENTED_EDGE ( 'NONE', *, *, #11681, .F. ) ;
#12348=CARTESIAN_POINT ( 'NONE',  ( 4.866781629985560187, 19.41732998781225916, 5.749491821935610147 ) ) ;
#12355=CARTESIAN_POINT ( 'NONE',  ( 11.11118388262826784, -16.62953976291649028, 18.34798005863226678 ) ) ;
#12356=ORIENTED_EDGE ( 'NONE', *, *, #1794, .T. ) ;
#12359=DIRECTION ( 'NONE',  ( 1.000000000000000000, 0.000000000000000000, 0.000000000000000000 ) ) ;
#12361=CARTESIAN_POINT ( 'NONE',  ( -17.96415918337694961, -8.831719996762313230, 20.32367522806703874 ) ) ;
#12368=PLANE ( 'NONE',  #21426 ) ;
#12378=EDGE_LOOP ( 'NONE', ( #1087, #7184 ) ) ;
#12380=ORIENTED_EDGE ( 'NONE', *, *, #80, .F. ) ;
#12382=EDGE_LOOP ( 'NONE', ( #20283, #16351, #6839, #5736 ) ) ;
#12386=DIRECTION ( 'NONE',  ( 1.000000000000000000, 0.000000000000000000, 0.000000000000000000 ) ) ;
#12387=AXIS2_PLACEMENT_3D ( 'NONE', #70, #2720, #19554 ) ;
#12388=CARTESIAN_POINT ( 'NONE',  ( 4.176140024798157491, 16.52246432927137931, 20.34789198813115618 ) ) ;
#12389=DIRECTION ( 'NONE',  ( 1.000000000000000000, 0.000000000000000000, 0.000000000000000000 ) ) ;
#12390=AXIS2_PLACEMENT_3D ( 'NONE', #27878, #24912, #13684 ) ;
#12395=CARTESIAN_POINT ( 'NONE',  ( 12.25310179107605002, 11.85582831497230138, 18.35718225375110180 ) ) ;
#12400=CARTESIAN_POINT ( 'NONE',  ( -8.550548368345314287, -14.74545326172986570, 20.34789198813115263 ) ) ;
#12403=CARTESIAN_POINT ( 'NONE',  ( -5.549075634136965363, 16.11684027513961226, 18.34798005863078885 ) ) ;
#12405=DIRECTION ( 'NONE',  ( 0.000000000000000000, 0.000000000000000000, 1.000000000000000000 ) ) ;
#12407=DIRECTION ( 'NONE',  ( 0.000000000000000000, 0.000000000000000000, 1.000000000000000000 ) ) ;
#12409=ORIENTED_EDGE ( 'NONE', *, *, #20863, .F. ) ;
#12411=CARTESIAN_POINT ( 'NONE',  ( -7.852931496087791174, -15.15760027743181482, 7.269896094239230777 ) ) ;
#12413=DIRECTION ( 'NONE',  ( 0.000000000000000000, 0.000000000000000000, 1.000000000000000000 ) ) ;
#12417=CIRCLE ( 'NONE', #13429, 9.482273699623480212 ) ;
#12418=CARTESIAN_POINT ( 'NONE',  ( -0.7220001660363114526, -9.454746441592957851, 13.00000000000000178 ) ) ;
#12421=CARTESIAN_POINT ( 'NONE',  ( 5.517068924551619347, 19.24285362756905471, 18.36582235739946611 ) ) ;
#12424=CARTESIAN_POINT ( 'NONE',  ( -7.785146467922785085, -15.19543897951832889, 18.84329447212443753 ) ) ;
#12428=CARTESIAN_POINT ( 'NONE',  ( 12.35846533491530685, 11.73919094685904341, 20.34789198813115263 ) ) ;
#12430=DIRECTION ( 'NONE',  ( -0.000000000000000000, -0.000000000000000000, 1.000000000000000000 ) ) ;
#12434=DIRECTION ( 'NONE',  ( -0.000000000000000000, -0.000000000000000000, 1.000000000000000000 ) ) ;
#12435=DIRECTION ( 'NONE',  ( -0.000000000000000000, -0.000000000000000000, 1.000000000000000000 ) ) ;
#12436=EDGE_CURVE ( 'NONE', #1600, #2106, #20525, .T. ) ;
#12449=CARTESIAN_POINT ( 'NONE',  ( -2.523760598493569596, 1.621922452366830747, 24.50000000000000000 ) ) ;
#12459=CARTESIAN_POINT ( 'NONE',  ( 12.87427757126085837, 11.14157019477620914, 18.71435384576123440 ) ) ;
#12461=CARTESIAN_POINT ( 'NONE',  ( -11.37242378808260668, -16.47377160145866171, 6.755862304746362845 ) ) ;
#12463=DIRECTION ( 'NONE',  ( 0.000000000000000000, 0.000000000000000000, -1.000000000000000000 ) ) ;
#12464=CARTESIAN_POINT ( 'NONE',  ( 19.66622914841314440, 3.734651121118245154, 18.50655187082627862 ) ) ;
#12466=EDGE_LOOP ( 'NONE', ( #3481, #14392 ) ) ;
#12468=ORIENTED_EDGE ( 'NONE', *, *, #13038, .T. ) ;
#12471=EDGE_CURVE ( 'NONE', #1853, #27034, #5989, .T. ) ;
#12474=CARTESIAN_POINT ( 'NONE',  ( -6.842536740270960038, 18.81187820119070508, 19.79423548914561692 ) ) ;
#12475=CARTESIAN_POINT ( 'NONE',  ( -14.79144470604038020, 13.48820156989937225, 18.80699882434806369 ) ) ;
#12481=CARTESIAN_POINT ( 'NONE',  ( 10.26788185420488553, -17.18392197670719668, 6.530762810602277924 ) ) ;
#12483=CARTESIAN_POINT ( 'NONE',  ( 19.76377475971901632, 3.067715173639373294, 5.651480102388687143 ) ) ;
#12489=CARTESIAN_POINT ( 'NONE',  ( -15.16307827826492627, -7.786259562520722710, 5.652196082368482699 ) ) ;
#12492=CARTESIAN_POINT ( 'NONE',  ( 5.549407557472018304, 19.21507098571442995, 7.626647697317578078 ) ) ;
#12494=DIRECTION ( 'NONE',  ( 0.000000000000000000, 0.000000000000000000, 1.000000000000000000 ) ) ;
#12495=CYLINDRICAL_SURFACE ( 'NONE', #21159, 20.00000000000000000 ) ;
#12496=CARTESIAN_POINT ( 'NONE',  ( 16.77777292147014876, 2.975267875541940832, 5.670038381137163519 ) ) ;
#12500=EDGE_CURVE ( 'NONE', #25827, #26330, #27096, .T. ) ;
#12503=DIRECTION ( 'NONE',  ( 1.000000000000000000, 0.000000000000000000, 0.000000000000000000 ) ) ;
#12506=CYLINDRICAL_SURFACE ( 'NONE', #26761, 1.000000000000000888 ) ;
#12509=DIRECTION ( 'NONE',  ( -0.2817325568414293380, -0.9594929736144974797, 0.000000000000000000 ) ) ;
#12513=CARTESIAN_POINT ( 'NONE',  ( 0.000000000000000000, 0.000000000000000000, 21.50000000000000000 ) ) ;
#12515=CARTESIAN_POINT ( 'NONE',  ( 10.27753383451899261, -17.15735655630020773, 19.08232364404840808 ) ) ;
#12519=DIRECTION ( 'NONE',  ( -0.000000000000000000, -0.000000000000000000, 1.000000000000000000 ) ) ;
#12526=CARTESIAN_POINT ( 'NONE',  ( 16.81773250897607141, 2.696729702855183763, 5.774779864094944593 ) ) ;
#12528=ORIENTED_EDGE ( 'NONE', *, *, #7287, .F. ) ;
#12532=B_SPLINE_CURVE_WITH_KNOTS ( 'NONE', 3,
 ( #21423, #12388, #23917, #24064, #9884, #26104, #2715, #9432, #21256, #21889, #21573, #24215, #14567, #4734, #19551, #19401, #29067, #7711, #28919, #209 ),
 .UNSPECIFIED., .F., .F.,
 ( 4, 2, 2, 2, 2, 2, 2, 2, 2, 4 ),
 ( 0.000000000000000000, 0.06250000000000170697, 0.1250000000000034139, 0.1875000000000051070, 0.2187500000000052736, 0.2500000000000054401, 0.3125000000000041078, 0.3750000000000027200, 0.4375000000000013878, 0.5000000000000000000 ),
 .UNSPECIFIED. ) ;
#12536=VERTEX_POINT ( 'NONE', #22409 ) ;
#12538=ADVANCED_FACE ( 'NONE', ( #5879 ), #15382, .F. ) ;
#12542=ADVANCED_FACE ( 'NONE', ( #1206 ), #10708, .T. ) ;
#12544=VECTOR ( 'NONE', #18533, 1000.000000000000227 ) ;
#12546=LINE ( 'NONE', #10653, #3400 ) ;
#12551=CARTESIAN_POINT ( 'NONE',  ( 14.89737979318874928, 13.37085219355980747, 20.34789198813115263 ) ) ;
#12552=DIRECTION ( 'NONE',  ( -0.000000000000000000, -0.000000000000000000, -1.000000000000000000 ) ) ;
#12553=ORIENTED_EDGE ( 'NONE', *, *, #6125, .F. ) ;
#12556=CARTESIAN_POINT ( 'NONE',  ( -15.13023987665973458, -7.854877310202119212, 5.652605728828375753 ) ) ;
#12557=CARTESIAN_POINT ( 'NONE',  ( -9.169883732660077058, -9.268939115642981008, 24.50000000000000000 ) ) ;
#12563=CARTESIAN_POINT ( 'NONE',  ( -8.550548372801092256, -14.74545326687210611, 7.652108011868850923 ) ) ;
#12564=CARTESIAN_POINT ( 'NONE',  ( -14.99868389510897160, 13.25752457422374775, 7.500898271101006820 ) ) ;
#12566=AXIS2_PLACEMENT_3D ( 'NONE', #16882, #15247, #14384 ) ;
#12567=VERTEX_POINT ( 'NONE', #25673 ) ;
#12569=CARTESIAN_POINT ( 'NONE',  ( 15.67696945782692097, -6.669264855739880815, 18.39701043959520987 ) ) ;
#12572=VERTEX_POINT ( 'NONE', #2426 ) ;
#12574=DIRECTION ( 'NONE',  ( 0.000000000000000000, 0.000000000000000000, 1.000000000000000000 ) ) ;
#12578=ORIENTED_EDGE ( 'NONE', *, *, #29610, .F. ) ;
#12582=CARTESIAN_POINT ( 'NONE',  ( -19.69217677393683630, 3.495450461901489447, 19.47728749465737863 ) ) ;
#12587=CARTESIAN_POINT ( 'NONE',  ( 15.81416692036122917, -6.360574302898113430, 5.652196082368483587 ) ) ;
#12588=VECTOR ( 'NONE', #14430, 1000.000000000000000 ) ;
#12590=FACE_OUTER_BOUND ( 'NONE', #18427, .T. ) ;
#12595=FACE_OUTER_BOUND ( 'NONE', #18334, .T. ) ;
#12596=CYLINDRICAL_SURFACE ( 'NONE', #5117, 20.00000000000000355 ) ;
#12598=ORIENTED_EDGE ( 'NONE', *, *, #22737, .F. ) ;
#12604=CARTESIAN_POINT ( 'NONE',  ( 15.18428249823343990, 13.04421712177833648, 18.44501272782439827 ) ) ;
#12606=EDGE_CURVE ( 'NONE', #12720, #19956, #20969, .T. ) ;
#12609=CARTESIAN_POINT ( 'NONE',  ( -16.82187727961404278, 2.603938281378752162, 6.974106381145714018 ) ) ;
#12610=CARTESIAN_POINT ( 'NONE',  ( 16.60164139905474201, 3.971857776421114483, 19.97651184436794125 ) ) ;
#12620=B_SPLINE_SURFACE_WITH_KNOTS ( 'NONE', 3, 1, ( 
 ( #19004, #9793 ),
 ( #5112, #21016 ),
 ( #2300, #4796 ),
 ( #30539, #30683 ),
 ( #6992, #26167 ),
 ( #11825, #21326 ),
 ( #14302, #5431 ),
 ( #435, #577 ),
 ( #26639, #2941 ),
 ( #9952, #3231 ),
 ( #10415, #10094 ),
 ( #21947, #19760 ),
 ( #26805, #17584 ),
 ( #19931, #5266 ),
 ( #27253, #19458 ),
 ( #29595, #12753 ),
 ( #3085, #3392 ),
 ( #24443, #14773 ),
 ( #19609, #14934 ),
 ( #7764, #27102 ),
 ( #29289, #12459 ),
 ( #15075, #8227 ),
 ( #29129, #22257 ),
 ( #28975, #12920 ),
 ( #12604, #24292 ),
 ( #17272, #22097 ),
 ( #728, #5723 ),
 ( #895, #7608 ),
 ( #24591, #17728 ),
 ( #10245, #29445 ),
 ( #17116, #7933 ) ),
 .UNSPECIFIED., .F., .F., .F.,
 ( 4, 3, 3, 3, 3, 3, 3, 3, 3, 3, 4 ),
 ( 2, 2 ),
 ( 0.000000000000000000, 0.05425176834609614362, 0.1085332949128348518, 0.1623767749169379715, 0.2157504826133058717, 0.2688657508888169789, 0.3218907763505471364, 0.3749548578363334772, 0.4282048033836237666, 0.4818374082110496448, 0.4999999999131653494 ),
 ( 0.000000000000000000, 1.000000000000000000 ),
 .UNSPECIFIED. ) ;
#12621=CARTESIAN_POINT ( 'NONE',  ( -6.290842788517063688, 19.00387417064636608, 20.29915277494337644 ) ) ;
#12622=CARTESIAN_POINT ( 'NONE',  ( -14.70379955820389206, 13.58362208154139772, 19.56050940960062690 ) ) ;
#12624=CARTESIAN_POINT ( 'NONE',  ( 9.185733585337910512, -2.352830851074146246, 13.00000000000000178 ) ) ;
#12625=EDGE_CURVE ( 'NONE', #27915, #20124, #23324, .T. ) ;
#12627=CIRCLE ( 'NONE', #4134, 9.482273699623480212 ) ;
#12631=CIRCLE ( 'NONE', #30055, 9.482273699623480212 ) ;
#12632=CARTESIAN_POINT ( 'NONE',  ( -17.00515754968434479, 1.312003563659741134, 5.704143890883081269 ) ) ;
#12634=CARTESIAN_POINT ( 'NONE',  ( -3.662523238938586001, -12.47340865698848056, 24.50000000000000000 ) ) ;
#12639=DIRECTION ( 'NONE',  ( 0.000000000000000000, 0.000000000000000000, 1.000000000000000000 ) ) ;
#12641=DIRECTION ( 'NONE',  ( 1.000000000000000000, 0.000000000000000000, 0.000000000000000000 ) ) ;
#12642=DIRECTION ( 'NONE',  ( -0.000000000000000000, -0.000000000000000000, 1.000000000000000000 ) ) ;
#12643=EDGE_CURVE ( 'NONE', #4157, #3062, #16612, .T. ) ;
#12646=EDGE_CURVE ( 'NONE', #3764, #14781, #6954, .T. ) ;
#12648=CARTESIAN_POINT ( 'NONE',  ( -9.748913725731210178, -17.46314199939011047, 18.84486140012299060 ) ) ;
#12649=CYLINDRICAL_SURFACE ( 'NONE', #13232, 1.000000000000004441 ) ;
#12650=EDGE_CURVE ( 'NONE', #26027, #15172, #21120, .T. ) ;
#12651=CARTESIAN_POINT ( 'NONE',  ( 19.88727842228974652, 2.283828795636142495, 7.080843742048788414 ) ) ;
#12653=CARTESIAN_POINT ( 'NONE',  ( 15.42025756663164948, 12.76459690492384702, 7.272049892295485485 ) ) ;
#12654=VECTOR ( 'NONE', #27447, 1000.000000000000000 ) ;
#12655=VERTEX_POINT ( 'NONE', #4753 ) ;
#12656=CARTESIAN_POINT ( 'NONE',  ( 18.43859109590531276, -7.792859017390147969, 7.627891251804737927 ) ) ;
#12663=CARTESIAN_POINT ( 'NONE',  ( -12.54846374865995706, -9.550116103605041928, 1.500000000000001332 ) ) ;
#12668=CARTESIAN_POINT ( 'NONE',  ( 10.89102995336899582, -16.77499580993352879, 18.37250658438899009 ) ) ;
#12671=CARTESIAN_POINT ( 'NONE',  ( -15.97838715008244748, 12.05808207567199197, 19.14333282897057842 ) ) ;
#12675=AXIS2_PLACEMENT_3D ( 'NONE', #27294, #12952, #5924 ) ;
#12679=DIRECTION ( 'NONE',  ( 0.000000000000000000, 0.000000000000000000, -1.000000000000000000 ) ) ;
#12684=CARTESIAN_POINT ( 'NONE',  ( 16.76419345869466326, 3.064929150614125408, 7.652108011868850035 ) ) ;
#12685=CARTESIAN_POINT ( 'NONE',  ( 19.69872561633593477, 3.460482060625765133, 5.679672709359371297 ) ) ;
#12686=EDGE_LOOP ( 'NONE', ( #13571, #15038, #7121, #17770 ) ) ;
#12690=ORIENTED_EDGE ( 'NONE', *, *, #22911, .T. ) ;
#12691=ORIENTED_EDGE ( 'NONE', *, *, #18157, .T. ) ;
#12697=VECTOR ( 'NONE', #14470, 1000.000000000000227 ) ;
#12708=CARTESIAN_POINT ( 'NONE',  ( -17.82234029294485111, -9.114408740892772087, 7.500147780736496017 ) ) ;
#12709=FACE_OUTER_BOUND ( 'NONE', #5505, .T. ) ;
#12710=CARTESIAN_POINT ( 'NONE',  ( 11.92709382895865389, -16.07640909887372516, 6.892848776733236704 ) ) ;
#12716=AXIS2_PLACEMENT_3D ( 'NONE', #25378, #8548, #20838 ) ;
#12717=CARTESIAN_POINT ( 'NONE',  ( -5.485816626893757153, 19.23332246807784074, 20.22277707861862694 ) ) ;
#12718=CARTESIAN_POINT ( 'NONE',  ( -12.74837729798237618, 11.28012212083751287, 6.310736198168394928 ) ) ;
#12720=VERTEX_POINT ( 'NONE', #17075 ) ;
#12722=CARTESIAN_POINT ( 'NONE',  ( 18.30707599941031560, -8.097116190180058126, 18.35377592296120497 ) ) ;
#12724=ORIENTED_EDGE ( 'NONE', *, *, #25792, .F. ) ;
#12725=CARTESIAN_POINT ( 'NONE',  ( 5.818449564404028607, 19.15386117387415865, 18.49267272388512140 ) ) ;
#12727=CARTESIAN_POINT ( 'NONE',  ( -7.322557715923444732, 14.41080185948837311, 1.500000000000000000 ) ) ;
#12732=DIRECTION ( 'NONE',  ( 0.000000000000000000, 0.000000000000000000, 1.000000000000000000 ) ) ;
#12733=DIRECTION ( 'NONE',  ( 0.000000000000000000, 0.000000000000000000, -1.000000000000000000 ) ) ;
#12734=CARTESIAN_POINT ( 'NONE',  ( -19.69701826448871174, 3.468437286170584333, 19.08232364404839743 ) ) ;
#12736=CARTESIAN_POINT ( 'NONE',  ( -15.30652580117162209, -7.480423316612006879, 5.701226463332907279 ) ) ;
#12737=AXIS2_PLACEMENT_3D ( 'NONE', #18590, #8931, #2040 ) ;
#12738=CARTESIAN_POINT ( 'NONE',  ( 12.35846533491530685, 11.73919094685904341, 20.34789198813115263 ) ) ;
#12743=DIRECTION ( 'NONE',  ( 1.000000000000000000, 0.000000000000000000, 0.000000000000000000 ) ) ;
#12744=ORIENTED_EDGE ( 'NONE', *, *, #23256, .F. ) ;
#12746=CARTESIAN_POINT ( 'NONE',  ( -11.86767874445213167, -1.850092897552710225, 1.500000000000001332 ) ) ;
#12750=LINE ( 'NONE', #15071, #7161 ) ;
#12753=CARTESIAN_POINT ( 'NONE',  ( 13.00882613046785075, 10.97723423515712859, 19.22654678686458141 ) ) ;
#12756=CARTESIAN_POINT ( 'NONE',  ( -16.96496223448355067, 1.652369715233091396, 7.652108011868850035 ) ) ;
#12761=CARTESIAN_POINT ( 'NONE',  ( -4.953525029936337809, 16.29343450965543738, 18.54473042795395443 ) ) ;
#12764=AXIS2_PLACEMENT_3D ( 'NONE', #19916, #3373, #15203 ) ;
#12765=ORIENTED_EDGE ( 'NONE', *, *, #22329, .F. ) ;
#12768=CARTESIAN_POINT ( 'NONE',  ( 16.63005575832080041, 3.830191698062872074, 5.872146474157316831 ) ) ;
#12769=CARTESIAN_POINT ( 'NONE',  ( -14.93957691572895818, 13.32381478560234456, 20.12545155307891065 ) ) ;
#12770=CARTESIAN_POINT ( 'NONE',  ( 1.043163081472838760, -17.02278858106119586, 7.652108011868851811 ) ) ;
#12771=EDGE_CURVE ( 'NONE', #21044, #29096, #19717, .T. ) ;
#12772=CIRCLE ( 'NONE', #6771, 0.7499999999999988898 ) ;
#12776=ORIENTED_EDGE ( 'NONE', *, *, #23258, .T. ) ;
#12777=PRODUCT_DEFINITION ( 'UNKNOWN', '', #9906, #27005 ) ;
#12778=CARTESIAN_POINT ( 'NONE',  ( 10.26079415706018771, -17.18817258638080503, 6.755862304746362845 ) ) ;
#12779=AXIS2_PLACEMENT_3D ( 'NONE', #26730, #24532, #10043 ) ;
#12781=CIRCLE ( 'NONE', #26712, 9.482273699623480212 ) ;
#12784=ORIENTED_EDGE ( 'NONE', *, *, #30141, .F. ) ;
#12791=DIRECTION ( 'NONE',  ( 1.000000000000000000, 0.000000000000000000, -0.000000000000000000 ) ) ;
#12792=CIRCLE ( 'NONE', #20265, 0.7500000000000006661 ) ;
#12794=( GEOMETRIC_REPRESENTATION_CONTEXT ( 3 ) GLOBAL_UNCERTAINTY_ASSIGNED_CONTEXT ( ( #14519 ) ) GLOBAL_UNIT_ASSIGNED_CONTEXT ( ( #14066, #23125, #4564 ) ) REPRESENTATION_CONTEXT ( 'NONE', 'WORKASPACE' ) );
#12795=CARTESIAN_POINT ( 'NONE',  ( 5.419676874198345651, 19.25213680916389691, 5.651480102388686255 ) ) ;
#12796=VERTEX_POINT ( 'NONE', #10207 ) ;
#12800=CARTESIAN_POINT ( 'NONE',  ( 19.88570912806761370, 2.296683858978091575, 6.211014596808754007 ) ) ;
#12803=EDGE_CURVE ( 'NONE', #2701, #18086, #25885, .T. ) ;
#12804=LINE ( 'NONE', #17789, #25283 ) ;
#12805=VERTEX_POINT ( 'NONE', #17389 ) ;
#12811=CARTESIAN_POINT ( 'NONE',  ( 16.74250988114178185, 3.198928528055117848, 5.652196082368483587 ) ) ;
#12816=CARTESIAN_POINT ( 'NONE',  ( 10.42711161940499487, -17.06705191410861744, 19.96302680909625238 ) ) ;
#12819=EDGE_CURVE ( 'NONE', #21250, #20491, #19930, .T. ) ;
#12823=CARTESIAN_POINT ( 'NONE',  ( -13.47895127716181207, 10.44112259311556556, 18.35718225375110180 ) ) ;
#12826=VECTOR ( 'NONE', #23148, 1000.000000000000114 ) ;
#12829=EDGE_CURVE ( 'NONE', #25657, #26575, #1498, .T. ) ;
#12831=CARTESIAN_POINT ( 'NONE',  ( 12.53355205349238233, 11.54212474472216776, 7.626437579292366209 ) ) ;
#12833=AXIS2_PLACEMENT_3D ( 'NONE', #24782, #5759, #29321 ) ;
#12838=EDGE_CURVE ( 'NONE', #21094, #1001, #690, .T. ) ;
#12839=ORIENTED_EDGE ( 'NONE', *, *, #12004, .F. ) ;
#12842=AXIS2_PLACEMENT_3D ( 'NONE', #6634, #19102, #4595 ) ;
#12843=CARTESIAN_POINT ( 'NONE',  ( 3.196529495465388226, 8.413215745755008967, 1.500000000000001332 ) ) ;
#12845=ORIENTED_EDGE ( 'NONE', *, *, #19867, .T. ) ;
#12846=CIRCLE ( 'NONE', #10838, 1.000000000000007772 ) ;
#12852=ADVANCED_FACE ( 'NONE', ( #10372 ), #24702, .F. ) ;
#12855=AXIS2_PLACEMENT_3D ( 'NONE', #8202, #29264, #29720 ) ;
#12859=DIRECTION ( 'NONE',  ( 0.000000000000000000, 0.000000000000000000, 1.000000000000000000 ) ) ;
#12860=LINE ( 'NONE', #10355, #15739 ) ;
#12863=AXIS2_PLACEMENT_3D ( 'NONE', #24561, #7584, #7431 ) ;
#12864=VERTEX_POINT ( 'NONE', #27378 ) ;
#12867=AXIS2_PLACEMENT_3D ( 'NONE', #10116, #29148, #7783 ) ;
#12868=CARTESIAN_POINT ( 'NONE',  ( -9.356685943497542013, -14.22000274044911805, 19.66989035740801839 ) ) ;
#12871=CARTESIAN_POINT ( 'NONE',  ( 11.55802067824463109, -16.34381896053850269, 7.500147780736496017 ) ) ;
#12873=CARTESIAN_POINT ( 'NONE',  ( 19.62935297797556444, -3.832558109936519575, 1.500000000000001332 ) ) ;
#12874=VECTOR ( 'NONE', #7939, 1000.000000000000114 ) ;
#12875=ORIENTED_EDGE ( 'NONE', *, *, #1487, .T. ) ;
#12880=CARTESIAN_POINT ( 'NONE',  ( -0.2301049870084636018, -17.01973991014544296, 6.519181285484531685 ) ) ;
#12882=CARTESIAN_POINT ( 'NONE',  ( 0.000000000000000000, 0.000000000000000000, 1.500000000000001332 ) ) ;
#12883=DIRECTION ( 'NONE',  ( -0.000000000000000000, -0.000000000000000000, 1.000000000000000000 ) ) ;
#12884=CIRCLE ( 'NONE', #6398, 20.00000000000000000 ) ;
#12886=CARTESIAN_POINT ( 'NONE',  ( 5.984782097461517125, 19.10229623552459088, 18.63641924841378028 ) ) ;
#12888=VECTOR ( 'NONE', #6699, 1000.000000000000114 ) ;
#12900=CARTESIAN_POINT ( 'NONE',  ( -9.169883732660077058, -9.268939115642981008, 1.500000000000001332 ) ) ;
#12904=DIRECTION ( 'NONE',  ( 1.000000000000000000, 0.000000000000000000, 0.000000000000000000 ) ) ;
#12906=LINE ( 'NONE', #22547, #30812 ) ;
#12911=CARTESIAN_POINT ( 'NONE',  ( -4.390207617113899730, 7.856594496258241023, 21.50000000000000000 ) ) ;
#12920=CARTESIAN_POINT ( 'NONE',  ( 12.71123406193363081, 11.33589958720536650, 18.49267272388512140 ) ) ;
#12923=CARTESIAN_POINT ( 'NONE',  ( -16.84919502704011052, 2.444546520875935158, 7.272049892295485485 ) ) ;
#12924=AXIS2_PLACEMENT_3D ( 'NONE', #23580, #9250, #13784 ) ;
#12926=B_SPLINE_CURVE_WITH_KNOTS ( 'NONE', 3,
 ( #6017, #8975, #1502, #11316, #6480, #3990, #13807, #27692, #4133, #6321, #11010, #11470, #1648, #20511, #18491, #3685 ),
 .UNSPECIFIED., .F., .F.,
 ( 4, 2, 2, 2, 2, 2, 2, 4 ),
 ( 0.5000000000000000000, 0.6250000000000021094, 0.6875000000000026645, 0.7187500000000029976, 0.7500000000000033307, 0.8125000000000023315, 0.8750000000000013323, 1.000000000000000000 ),
 .UNSPECIFIED. ) ;
#12940=DIRECTION ( 'NONE',  ( 0.000000000000000000, 0.000000000000000000, 1.000000000000000000 ) ) ;
#12941=ORIENTED_EDGE ( 'NONE', *, *, #10742, .F. ) ;
#12942=CARTESIAN_POINT ( 'NONE',  ( 9.025811419443956041, -14.43167044742872207, 6.420335371522007506 ) ) ;
#12943=AXIS2_PLACEMENT_3D ( 'NONE', #25112, #10767, #7979 ) ;
#12947=CARTESIAN_POINT ( 'NONE',  ( 18.12802117124498835, -8.449244086891157579, 20.22277707861862339 ) ) ;
#12949=CARTESIAN_POINT ( 'NONE',  ( -5.010690217951878189, 19.38064900392119227, 6.530762810602277924 ) ) ;
#12952=DIRECTION ( 'NONE',  ( 0.000000000000000000, 0.000000000000000000, 1.000000000000000000 ) ) ;
#12956=CARTESIAN_POINT ( 'NONE',  ( 11.98626544954001005, 12.14249340222027840, 5.810767894563978686 ) ) ;
#12957=CARTESIAN_POINT ( 'NONE',  ( 16.84609478243855563, 2.477959627222518613, 7.359006845440219102 ) ) ;
#12959=LINE ( 'NONE', #1100, #8351 ) ;
#12964=ORIENTED_EDGE ( 'NONE', *, *, #17222, .T. ) ;
#12966=CARTESIAN_POINT ( 'NONE',  ( 5.089453839167154214, 19.35995229554825769, 7.627891251804737927 ) ) ;
#12969=CARTESIAN_POINT ( 'NONE',  ( 5.291489565152559749, 19.28730510418394672, 18.34798005863226678 ) ) ;
#12976=CARTESIAN_POINT ( 'NONE',  ( -15.80654879600848162, 12.28271411401623503, 20.06253562465620632 ) ) ;
#12977=DIRECTION ( 'NONE',  ( 0.7557495743542582689, -0.6548607339452849896, 0.000000000000000000 ) ) ;
#12978=CARTESIAN_POINT ( 'NONE',  ( -3.662523238938586001, -12.47340865698848056, 1.500000000000001332 ) ) ;
#12979=VERTEX_POINT ( 'NONE', #3511 ) ;
#12983=CARTESIAN_POINT ( 'NONE',  ( -14.69500743155267486, 13.56684717634543347, 19.08232364404840098 ) ) ;
#12987=CARTESIAN_POINT ( 'NONE',  ( 16.78337223357194574, 2.938206247955208905, 5.676815824193228721 ) ) ;
#12989=CYLINDRICAL_SURFACE ( 'NONE', #3623, 1.000000000000010436 ) ;
#12993=ORIENTED_EDGE ( 'NONE', *, *, #21531, .F. ) ;
#12997=CARTESIAN_POINT ( 'NONE',  ( -19.77413607932156481, 2.999736578675605170, 7.526993102356318133 ) ) ;
#13001=CARTESIAN_POINT ( 'NONE',  ( 0.3158150563615978457, -20.01532941283344158, 18.34777357837151968 ) ) ;
#13008=CARTESIAN_POINT ( 'NONE',  ( -11.19063532726251609, -16.57644352599300319, 6.033082186765053478 ) ) ;
#13009=DIRECTION ( 'NONE',  ( 1.000000000000000000, 0.000000000000000000, 0.000000000000000000 ) ) ;
#13010=CARTESIAN_POINT ( 'NONE',  ( 0.3541522971493289429, -20.01464067411589198, 5.652196082364321583 ) ) ;
#13014=EDGE_CURVE ( 'NONE', #984, #23438, #11291, .T. ) ;
#13016=CARTESIAN_POINT ( 'NONE',  ( -6.575147850411299899, 18.90724948634255753, 7.441806358946449151 ) ) ;
#13017=ADVANCED_FACE ( 'NONE', ( #18770 ), #15971, .F. ) ;
#13018=CARTESIAN_POINT ( 'NONE',  ( 10.57816699686867601, -13.40145493435145774, 6.131018562779544823 ) ) ;
#13022=DIRECTION ( 'NONE',  ( -0.000000000000000000, -0.000000000000000000, -1.000000000000000000 ) ) ;
#13027=CARTESIAN_POINT ( 'NONE',  ( -12.71685080539083934, 11.31419172277363749, 6.530762810602277924 ) ) ;
#13030=CARTESIAN_POINT ( 'NONE',  ( 0.000000000000000000, 0.000000000000000000, 1.500000000000001332 ) ) ;
#13032=CARTESIAN_POINT ( 'NONE',  ( -9.321015140911132590, -14.24452793913984650, 7.080843742048788414 ) ) ;
#13035=CARTESIAN_POINT ( 'NONE',  ( 4.654893560761752980, 16.38086414125080736, 18.55820869691756769 ) ) ;
#13036=EDGE_CURVE ( 'NONE', #15693, #12097, #18474, .T. ) ;
#13038=EDGE_CURVE ( 'NONE', #22613, #1600, #18408, .T. ) ;
#13039=CARTESIAN_POINT ( 'NONE',  ( 19.72123249184183180, 3.330269068327009752, 18.34869673959212122 ) ) ;
#13040=ORIENTED_EDGE ( 'NONE', *, *, #12829, .F. ) ;
#13041=CARTESIAN_POINT ( 'NONE',  ( 5.296161872597630271, 19.28602264385380849, 7.652108011868850035 ) ) ;
#13042=EDGE_CURVE ( 'NONE', #10258, #15172, #13423, .T. ) ;
#13045=CARTESIAN_POINT ( 'NONE',  ( 8.999114229549594057, -0.1262659238204522361, 21.50000000000000000 ) ) ;
#13046=CARTESIAN_POINT ( 'NONE',  ( -19.84404562991029763, 2.492760124447683800, 18.34798005863226678 ) ) ;
#13056=CARTESIAN_POINT ( 'NONE',  ( 11.82521593960875173, 5.400395169024529984, 1.500000000000001332 ) ) ;
#13058=CIRCLE ( 'NONE', #25982, 0.7500000000000006661 ) ;
#13064=CARTESIAN_POINT ( 'NONE',  ( 0.000000000000000000, 0.000000000000000000, 1.500000000000001332 ) ) ;
#13065=CARTESIAN_POINT ( 'NONE',  ( 1.964582201835905151, 2.267248723062786908, 24.50000000000000000 ) ) ;
#13069=ADVANCED_FACE ( 'NONE', ( #28130, #13646, #27978 ), #20934, .T. ) ;
#13072=DIRECTION ( 'NONE',  ( 1.000000000000000000, 0.000000000000000000, 0.000000000000000000 ) ) ;
#13073=ORIENTED_EDGE ( 'NONE', *, *, #30330, .T. ) ;
#13075=CARTESIAN_POINT ( 'NONE',  ( 16.02044690728354936, -5.868896442471950081, 20.19593175699879595 ) ) ;
#13077=CARTESIAN_POINT ( 'NONE',  ( -8.917851762035226670, -14.51287734179233446, 18.44501272782439827 ) ) ;
#13079=ORIENTED_EDGE ( 'NONE', *, *, #4571, .T. ) ;
#13085=CARTESIAN_POINT ( 'NONE',  ( -6.809999484610175458, 18.80496293131997732, 19.85730954408918336 ) ) ;
#13087=CARTESIAN_POINT ( 'NONE',  ( 19.70572240696341026, 3.522277800415036353, 7.603368798681074736 ) ) ;
#13088=CARTESIAN_POINT ( 'NONE',  ( -15.30875331599079736, 12.89789204219718854, 18.34969686940296185 ) ) ;
#13089=CARTESIAN_POINT ( 'NONE',  ( -8.423436389728852447, -14.82351904252668717, 20.33971507717571114 ) ) ;
#13090=CARTESIAN_POINT ( 'NONE',  ( -16.96496224101209194, 1.652369717150043549, 20.34789198813115263 ) ) ;
#13092=DIRECTION ( 'NONE',  ( 0.7557495743542582689, -0.6548607339452849896, 0.000000000000000000 ) ) ;
#13094=CARTESIAN_POINT ( 'NONE',  ( -13.83213539500865785, 7.758783772730382111, 24.50000000000000000 ) ) ;
#13095=CARTESIAN_POINT ( 'NONE',  ( 10.57816699686867068, -13.40145493435145063, 18.82680253904184298 ) ) ;
#13098=ORIENTED_EDGE ( 'NONE', *, *, #25359, .T. ) ;
#13102=AXIS2_PLACEMENT_3D ( 'NONE', #12911, #22247, #5420 ) ;
#13103=CYLINDRICAL_SURFACE ( 'NONE', #11870, 0.7499999999999997780 ) ;
#13104=VERTEX_POINT ( 'NONE', #4568 ) ;
#13105=FACE_OUTER_BOUND ( 'NONE', #27440, .T. ) ;
#13107=ADVANCED_FACE ( 'NONE', ( #11143, #6606, #13492 ), #30458, .T. ) ;
#13108=CARTESIAN_POINT ( 'NONE',  ( 5.524309650260771143, -7.706848733600969226, 1.500000000000001332 ) ) ;
#13111=CARTESIAN_POINT ( 'NONE',  ( 12.05308393316171944, 12.07205540120323128, 5.749491821935610147 ) ) ;
#13112=CARTESIAN_POINT ( 'NONE',  ( 19.85228648261877282, 2.570616772381430604, 5.862424720655265098 ) ) ;
#13114=CARTESIAN_POINT ( 'NONE',  ( 14.91976180470934388, 13.34593040386456408, 5.651989602109218858 ) ) ;
#13116=CARTESIAN_POINT ( 'NONE',  ( -13.97970881677390587, 9.806700574777895696, 19.02573955821369367 ) ) ;
#13119=VERTEX_POINT ( 'NONE', #21236 ) ;
#13121=CARTESIAN_POINT ( 'NONE',  ( 4.318335944327696296, 19.54627428603377126, 6.782048567692550378 ) ) ;
#13122=DIRECTION ( 'NONE',  ( -0.000000000000000000, -0.000000000000000000, 1.000000000000000000 ) ) ;
#13123=CARTESIAN_POINT ( 'NONE',  ( -7.869584159753960861, 10.39565510934976977, 1.500000000000001332 ) ) ;
#13127=ORIENTED_EDGE ( 'NONE', *, *, #28866, .T. ) ;
#13128=CARTESIAN_POINT ( 'NONE',  ( -16.81263688882341967, 2.656251026639211865, 19.33715507985239412 ) ) ;
#13129=CARTESIAN_POINT ( 'NONE',  ( 17.94887244118349301, -8.863227448567840838, 6.310736198168394928 ) ) ;
#13130=CARTESIAN_POINT ( 'NONE',  ( -13.88241978398541576, 9.934084310449183164, 18.73743063545763121 ) ) ;
#13135=CARTESIAN_POINT ( 'NONE',  ( 0.000000000000000000, 0.000000000000000000, 1.500000000000001332 ) ) ;
#13137=CARTESIAN_POINT ( 'NONE',  ( 12.99618331673367244, 10.99290767929104540, 6.385774490351133537 ) ) ;
#13140=LINE ( 'NONE', #5806, #15886 ) ;
#13142=CARTESIAN_POINT ( 'NONE',  ( 16.87927834490895052, 2.194149605794860847, 6.714907520933423690 ) ) ;
#13145=DIRECTION ( 'NONE',  ( -0.000000000000000000, -0.000000000000000000, 1.000000000000000000 ) ) ;
#13151=CARTESIAN_POINT ( 'NONE',  ( -5.687793815610304726, 6.974883619896852238, 21.50000000000000000 ) ) ;
#13157=CARTESIAN_POINT ( 'NONE',  ( 0.000000000000000000, 0.000000000000000000, 21.50000000000000000 ) ) ;
#13158=CARTESIAN_POINT ( 'NONE',  ( -8.499586724479453181, -2.959227181723774525, 21.50000000000000000 ) ) ;
#13159=CARTESIAN_POINT ( 'NONE',  ( -1.687027447297492211, -8.840471615930066918, 1.500000000000001332 ) ) ;
#13162=AXIS2_PLACEMENT_3D ( 'NONE', #20441, #18103, #6242 ) ;
#13163=CARTESIAN_POINT ( 'NONE',  ( -11.24586906513001772, -16.56046035145272199, 18.80699882434806369 ) ) ;
#13165=CARTESIAN_POINT ( 'NONE',  ( -5.544451647051929832, 16.11829164193972019, 7.652108011868850923 ) ) ;
#13166=CARTESIAN_POINT ( 'NONE',  ( 9.864935476092966837, -13.90063640548121171, 5.652196082364323360 ) ) ;
#13171=VERTEX_POINT ( 'NONE', #16425 ) ;
#13174=CARTESIAN_POINT ( 'NONE',  ( -12.78170796079387195, 11.24374406685325134, 6.211014596808754007 ) ) ;
#13176=EDGE_CURVE ( 'NONE', #863, #17560, #17245, .T. ) ;
#13179=CARTESIAN_POINT ( 'NONE',  ( 3.190007960661453534, 16.77295862815147842, 7.158811349119584833 ) ) ;
#13181=CARTESIAN_POINT ( 'NONE',  ( -10.90225941753887362, -16.78887681002774812, 7.557577766377196582 ) ) ;
#13184=EDGE_CURVE ( 'NONE', #27848, #28528, #30340, .T. ) ;
#13185=ORIENTED_EDGE ( 'NONE', *, *, #11681, .T. ) ;
#13189=CARTESIAN_POINT ( 'NONE',  ( 19.65639872822723078, 3.693339721720559687, 20.22386025856690139 ) ) ;
#13190=EDGE_LOOP ( 'NONE', ( #1069, #29762, #15650, #1430 ) ) ;
#13191=DIRECTION ( 'NONE',  ( -0.4154150130018972598, -0.9096319953545133341, 0.000000000000000000 ) ) ;
#13193=VECTOR ( 'NONE', #27383, 1000.000000000000000 ) ;
#13195=ORIENTED_EDGE ( 'NONE', *, *, #12829, .T. ) ;
#13201=CIRCLE ( 'NONE', #30614, 0.7500000000000006661 ) ;
#13206=EDGE_CURVE ( 'NONE', #2106, #24485, #10024, .T. ) ;
#13207=CARTESIAN_POINT ( 'NONE',  ( 9.340794358757445792, -14.23940931083286898, 7.453286057244485008 ) ) ;
#13216=ADVANCED_FACE ( 'NONE', ( #2543 ), #12368, .F. ) ;
#13218=CIRCLE ( 'NONE', #29144, 0.7500000000000002220 ) ;
#13225=CARTESIAN_POINT ( 'NONE',  ( -16.87560513830565867, 2.281487909151090232, 7.429667576816606278 ) ) ;
#13227=CARTESIAN_POINT ( 'NONE',  ( 19.63374410927882963, 3.902325345048615279, 20.06253562465620632 ) ) ;
#13228=CARTESIAN_POINT ( 'NONE',  ( -8.643687819870514488, -14.68753251638875490, 18.35377592296120497 ) ) ;
#13230=VERTEX_POINT ( 'NONE', #7381 ) ;
#13231=CYLINDRICAL_SURFACE ( 'NONE', #21303, 0.7500000000000006661 ) ;
#13232=AXIS2_PLACEMENT_3D ( 'NONE', #14815, #29012, #14660 ) ;
#13237=ADVANCED_FACE ( 'NONE', ( #26707 ), #9555, .F. ) ;
#13238=FACE_OUTER_BOUND ( 'NONE', #372, .T. ) ;
#13240=CARTESIAN_POINT ( 'NONE',  ( 19.57650873258265989, 4.179294809495486263, 6.447548852708279377 ) ) ;
#13241=CARTESIAN_POINT ( 'NONE',  ( -12.96684546537104588, 11.03909700805841965, 18.55820869691756769 ) ) ;
#13242=ADVANCED_FACE ( 'NONE', ( #5654 ), #28900, .F. ) ;
#13245=CARTESIAN_POINT ( 'NONE',  ( -17.06384985643509822, 0.6725948717545796596, 19.08844262864049313 ) ) ;
#13246=CARTESIAN_POINT ( 'NONE',  ( -8.774062814044063074, -14.60569725947857833, 7.626437579292365321 ) ) ;
#13249=EDGE_CURVE ( 'NONE', #4645, #19042, #13140, .T. ) ;
#13250=CARTESIAN_POINT ( 'NONE',  ( 10.65192122195201385, -13.34697535456211703, 19.03762469184452755 ) ) ;
#13257=CARTESIAN_POINT ( 'NONE',  ( -4.786560543001539436, 16.33923032321832736, 6.018569869498933578 ) ) ;
#13258=ORIENTED_EDGE ( 'NONE', *, *, #24444, .T. ) ;
#13259=FACE_BOUND ( 'NONE', #6351, .T. ) ;
#13263=ORIENTED_EDGE ( 'NONE', *, *, #28425, .T. ) ;
#13264=CARTESIAN_POINT ( 'NONE',  ( -2.094186647214681063, 9.248129367672087042, 13.00000000000000178 ) ) ;
#13269=CARTESIAN_POINT ( 'NONE',  ( 12.64536614603776066, 11.41255465792765555, 5.749228751562096562 ) ) ;
#13272=ORIENTED_EDGE ( 'NONE', *, *, #10346, .F. ) ;
#13275=CARTESIAN_POINT ( 'NONE',  ( 4.365174083970719821, 19.53587658871429156, 6.341840715582230281 ) ) ;
#13281=CARTESIAN_POINT ( 'NONE',  ( 10.66524827722686197, -16.94040236790928944, 18.49267272388512140 ) ) ;
#13282=CARTESIAN_POINT ( 'NONE',  ( 19.86411046155384952, 2.477959627222519057, 20.05479082170252525 ) ) ;
#13283=VERTEX_POINT ( 'NONE', #19842 ) ;
#13284=CARTESIAN_POINT ( 'NONE',  ( -16.84919502704010696, 2.444546520875934270, 19.96783386855779341 ) ) ;
#13285=CARTESIAN_POINT ( 'NONE',  ( 15.39534585122291332, -7.260971684546494664, 6.420335371522007506 ) ) ;
#13286=CARTESIAN_POINT ( 'NONE',  ( -13.47385700491362570, 10.44730466805193281, 20.33971507717571114 ) ) ;
#13288=CARTESIAN_POINT ( 'NONE',  ( 3.728348255937726563, 16.64288108867316396, 20.29915277494337644 ) ) ;
#13289=ORIENTED_EDGE ( 'NONE', *, *, #15251, .F. ) ;
#13294=FACE_OUTER_BOUND ( 'NONE', #5588, .T. ) ;
#13297=CARTESIAN_POINT ( 'NONE',  ( -7.706848733600990542, -5.524309650260742721, 1.500000000000001332 ) ) ;
#13298=CIRCLE ( 'NONE', #10794, 0.7500000000000015543 ) ;
#13301=VECTOR ( 'NONE', #11972, 1000.000000000000114 ) ;
#13302=AXIS2_PLACEMENT_3D ( 'NONE', #29082, #21737, #10054 ) ;
#13307=CARTESIAN_POINT ( 'NONE',  ( -19.71440049134193728, 3.368233808196386292, 6.144783687052523646 ) ) ;
#13309=B_SPLINE_CURVE_WITH_KNOTS ( 'NONE', 3,
 ( #12738, #19912, #29426, #3368, #20366, #3832, #17563, #1338, #24726, #10856, #22236, #8060, #15200, #25814, #15834, #9119, #20661, #4446, #11165, #11471 ),
 .UNSPECIFIED., .F., .F.,
 ( 4, 2, 2, 2, 2, 2, 2, 2, 2, 4 ),
 ( 0.000000000000000000, 0.06250000000000194289, 0.1250000000000038858, 0.1875000000000058287, 0.2187500000000059119, 0.2500000000000059952, 0.3125000000000044964, 0.3750000000000029976, 0.4375000000000014988, 0.5000000000000000000 ),
 .UNSPECIFIED. ) ;
#13310=CARTESIAN_POINT ( 'NONE',  ( -19.84404562991029763, 2.492760124447683800, 18.34798005863226678 ) ) ;
#13311=ORIENTED_EDGE ( 'NONE', *, *, #17165, .F. ) ;
#13320=CARTESIAN_POINT ( 'NONE',  ( 0.4984457374290394149, -20.01168570850557415, 7.643931100913408550 ) ) ;
#13321=CARTESIAN_POINT ( 'NONE',  ( -16.84831847205055411, 2.450595478048609444, 7.267659094423558841 ) ) ;
#13322=ORIENTED_EDGE ( 'NONE', *, *, #15478, .F. ) ;
#13324=CARTESIAN_POINT ( 'NONE',  ( -9.002647793593395065, -14.45788447640154040, 18.49267272388512140 ) ) ;
#13327=CARTESIAN_POINT ( 'NONE',  ( 10.13630142350640817, -13.71646693216191082, 7.603368798681074736 ) ) ;
#13336=LINE ( 'NONE', #20180, #6113 ) ;
#13337=ORIENTED_EDGE ( 'NONE', *, *, #8669, .T. ) ;
#13339=CIRCLE ( 'NONE', #19797, 9.482273699623480212 ) ;
#13341=CARTESIAN_POINT ( 'NONE',  ( -8.611567383417474630, -14.70762963579928773, 5.653912893140659257 ) ) ;
#13344=VECTOR ( 'NONE', #20767, 1000.000000000000000 ) ;
#13348=VERTEX_POINT ( 'NONE', #20308 ) ;
#13352=DIRECTION ( 'NONE',  ( -0.000000000000000000, -0.000000000000000000, 1.000000000000000000 ) ) ;
#13357=CARTESIAN_POINT ( 'NONE',  ( -3.196529495465446402, -8.413215745754985875, 1.500000000000001332 ) ) ;
#13358=ADVANCED_FACE ( 'NONE', ( #29837 ), #8154, .F. ) ;
#13361=CARTESIAN_POINT ( 'NONE',  ( -17.05621956093816749, 0.7704973847036212797, 7.158811349119585721 ) ) ;
#13371=EDGE_CURVE ( 'NONE', #6597, #26415, #2933, .T. ) ;
#13374=AXIS2_PLACEMENT_3D ( 'NONE', #18724, #28236, #6866 ) ;
#13375=CARTESIAN_POINT ( 'NONE',  ( -4.163336342344337027E-14, 1.387778780781445676E-14, 1.500000000000000000 ) ) ;
#13380=CIRCLE ( 'NONE', #22822, 10.00000000000000000 ) ;
#13384=CARTESIAN_POINT ( 'NONE',  ( -16.90598708042469056, 2.083096162940500484, 5.749228751562096562 ) ) ;
#13386=CARTESIAN_POINT ( 'NONE',  ( 15.40745978470623534, 12.75221478727798896, 6.033082186765058808 ) ) ;
#13391=VERTEX_POINT ( 'NONE', #13297 ) ;
#13393=DIRECTION ( 'NONE',  ( -0.000000000000000000, -0.000000000000000000, 1.000000000000000000 ) ) ;
#13394=CARTESIAN_POINT ( 'NONE',  ( -16.93131609043274821, 1.909234121842923626, 18.37259980046034613 ) ) ;
#13395=ORIENTED_EDGE ( 'NONE', *, *, #3494, .T. ) ;
#13396=CARTESIAN_POINT ( 'NONE',  ( -6.742350454026563078, 18.82948505227175318, 18.73377938172348678 ) ) ;
#13401=B_SPLINE_SURFACE_WITH_KNOTS ( 'NONE', 3, 1, ( 
 ( #20589, #9202 ),
 ( #30114, #13888 ),
 ( #29969, #2027 ),
 ( #25592, #8745 ),
 ( #4069, #25446 ),
 ( #13597, #22933 ),
 ( #11552, #3930 ),
 ( #18716, #8607 ),
 ( #18113, #15607 ),
 ( #28225, #25125 ),
 ( #4212, #23075 ),
 ( #20733, #27787 ),
 ( #3768, #6414 ),
 ( #27628, #1880 ),
 ( #23225, #1585 ),
 ( #30266, #8912 ),
 ( #11403, #6252 ),
 ( #15763, #18575 ),
 ( #20895, #18435 ),
 ( #27937, #6564 ),
 ( #16076, #30420 ),
 ( #9057, #4674 ),
 ( #6858, #21354 ),
 ( #11408, #4522 ),
 ( #14338, #16683 ),
 ( #9663, #14176 ),
 ( #24150, #26042 ),
 ( #21823, #14031 ),
 ( #11696, #23535 ),
 ( #12318, #464 ),
 ( #4983, #28695 ) ),
 .UNSPECIFIED., .F., .F., .F.,
 ( 4, 3, 3, 3, 3, 3, 3, 3, 3, 3, 4 ),
 ( 2, 2 ),
 ( 0.4999999998345682206, 0.5360336730431942698, 0.5907651151589017324, 0.6456034593241839481, 0.6998270958050443191, 0.7529536536315944995, 0.8052385063053264513, 0.8575343587103996246, 0.9106564858195047574, 0.9648414833209688624, 1.000000006602610014 ),
 ( 0.000000000000000000, 1.000000000000000000 ),
 .UNSPECIFIED. ) ;
#13402=CARTESIAN_POINT ( 'NONE',  ( -0.08122345276805190140, -17.02407875822364147, 7.176035686813569292 ) ) ;
#13403=AXIS2_PLACEMENT_3D ( 'NONE', #14832, #24653, #22618 ) ;
#13404=CIRCLE ( 'NONE', #3411, 9.482273699623480212 ) ;
#13405=AXIS2_PLACEMENT_3D ( 'NONE', #16470, #4922, #21448 ) ;
#13406=CARTESIAN_POINT ( 'NONE',  ( 19.74251403343738076, 3.198927889078825970, 5.652196082369965069 ) ) ;
#13409=CARTESIAN_POINT ( 'NONE',  ( -17.04337418722499820, 0.9225192032720760382, 18.64703902303423178 ) ) ;
#13411=ORIENTED_EDGE ( 'NONE', *, *, #6483, .T. ) ;
#13420=FACE_OUTER_BOUND ( 'NONE', #18166, .T. ) ;
#13421=CARTESIAN_POINT ( 'NONE',  ( -7.730328572437709767, 4.608906612435681005, 1.500000000000001332 ) ) ;
#13423=CIRCLE ( 'NONE', #7438, 0.7500000000000006661 ) ;
#13429=AXIS2_PLACEMENT_3D ( 'NONE', #15293, #3462, #10476 ) ;
#13430=CARTESIAN_POINT ( 'NONE',  ( -8.430595340551228389, 4.340342926365043930, 13.00000000000000178 ) ) ;
#13434=ORIENTED_EDGE ( 'NONE', *, *, #189, .T. ) ;
#13439=ADVANCED_FACE ( 'NONE', ( #20600 ), #6427, .F. ) ;
#13440=VERTEX_POINT ( 'NONE', #15942 ) ;
#13441=CARTESIAN_POINT ( 'NONE',  ( 9.163215745754998309, -3.196529495465417980, 1.500000000000001332 ) ) ;
#13442=CARTESIAN_POINT ( 'NONE',  ( 5.549407557472024521, 19.21507098571442285, 20.32243167357988867 ) ) ;
#13443=VERTEX_POINT ( 'NONE', #20905 ) ;
#13445=CYLINDRICAL_SURFACE ( 'NONE', #23761, 0.7500000000000006661 ) ;
#13446=CARTESIAN_POINT ( 'NONE',  ( 19.89210292178043460, 2.240810012149824892, 19.66989035740801839 ) ) ;
#13449=CARTESIAN_POINT ( 'NONE',  ( -12.72536390617885260, -2.839914339433650348, 1.500000000000001332 ) ) ;
#13452=CARTESIAN_POINT ( 'NONE',  ( 4.972463595808062742, 19.39063357279558275, 18.39992786714538298 ) ) ;
#13456=CARTESIAN_POINT ( 'NONE',  ( 10.08077896144684260, -13.75650449134903397, 7.652108011868851811 ) ) ;
#13457=CARTESIAN_POINT ( 'NONE',  ( 14.96781329949620165, 13.26582956964653448, 18.34726407865098707 ) ) ;
#13458=CARTESIAN_POINT ( 'NONE',  ( -4.997519263521717825, 19.38405562624022949, 19.33715507985239412 ) ) ;
#13461=VECTOR ( 'NONE', #5044, 1000.000000000000000 ) ;
#13463=DIRECTION ( 'NONE',  ( 0.000000000000000000, 0.000000000000000000, -1.000000000000000000 ) ) ;
#13470=DIRECTION ( 'NONE',  ( 0.000000000000000000, 0.000000000000000000, -1.000000000000000000 ) ) ;
#13472=ORIENTED_EDGE ( 'NONE', *, *, #30410, .F. ) ;
#13473=CARTESIAN_POINT ( 'NONE',  ( -19.69701826448871174, 3.468437286170584777, 6.386539667786103713 ) ) ;
#13476=CARTESIAN_POINT ( 'NONE',  ( -0.6570508600772840824, -19.98920419113417069, 6.518927109361846384 ) ) ;
#13478=CARTESIAN_POINT ( 'NONE',  ( 5.130938270761610021, -7.974144905643801629, 21.50000000000000000 ) ) ;
#13481=CARTESIAN_POINT ( 'NONE',  ( -5.694318326875605685, 16.07090250511087248, 18.35718225375110180 ) ) ;
#13483=CARTESIAN_POINT ( 'NONE',  ( 1.797484530300063721, -16.98352104300882814, 6.560937769032974209 ) ) ;
#13486=CARTESIAN_POINT ( 'NONE',  ( 0.000000000000000000, 0.000000000000000000, 1.500000000000001332 ) ) ;
#13488=CARTESIAN_POINT ( 'NONE',  ( -5.292460272911076125, 16.19569186419612805, 7.626437579292365321 ) ) ;
#13492=FACE_BOUND ( 'NONE', #18595, .T. ) ;
#13495=LINE ( 'NONE', #4119, #3186 ) ;
#13496=EDGE_LOOP ( 'NONE', ( #17952, #3344, #18418, #23114 ) ) ;
#13497=CIRCLE ( 'NONE', #26437, 20.00000000000000000 ) ;
#13500=DIRECTION ( 'NONE',  ( -0.000000000000000000, -0.000000000000000000, 1.000000000000000000 ) ) ;
#13509=CARTESIAN_POINT ( 'NONE',  ( -10.52279982399693559, -17.02885636288122129, 5.652196082364321583 ) ) ;
#13510=CARTESIAN_POINT ( 'NONE',  ( 4.390207617113956573, -7.856594496258208160, 1.500000000000001332 ) ) ;
#13511=CARTESIAN_POINT ( 'NONE',  ( 0.8597189258598725292, -17.02598424914432584, 18.34838970509067479 ) ) ;
#13517=CIRCLE ( 'NONE', #8034, 9.482273699623480212 ) ;
#13521=CARTESIAN_POINT ( 'NONE',  ( 4.622016212553096359, -12.19167610014704906, 1.500000000000001332 ) ) ;
#13526=ORIENTED_EDGE ( 'NONE', *, *, #266, .F. ) ;
#13527=DIRECTION ( 'NONE',  ( -0.000000000000000000, -0.000000000000000000, 1.000000000000000000 ) ) ;
#13532=DIRECTION ( 'NONE',  ( -0.2817325568414293380, -0.9594929736144974797, 0.000000000000000000 ) ) ;
#13533=CARTESIAN_POINT ( 'NONE',  ( 9.007774317138297349, -14.44244895400449558, 19.41069149716886955 ) ) ;
#13536=VERTEX_POINT ( 'NONE', #893 ) ;
#13537=CARTESIAN_POINT ( 'NONE',  ( -10.94076559809103699, -16.74260033555410843, 18.47110296274026098 ) ) ;
#13538=CYLINDRICAL_SURFACE ( 'NONE', #16266, 0.7500000000000015543 ) ;
#13543=LINE ( 'NONE', #28023, #4366 ) ;
#13544=EDGE_LOOP ( 'NONE', ( #24605, #19190 ) ) ;
#13548=DIRECTION ( 'NONE',  ( -0.000000000000000000, -0.000000000000000000, 1.000000000000000000 ) ) ;
#13550=AXIS2_PLACEMENT_3D ( 'NONE', #18224, #16034, #24931 ) ;
#13554=LINE ( 'NONE', #6214, #5568 ) ;
#13555=CARTESIAN_POINT ( 'NONE',  ( -17.05537006572907899, 0.7816414089123745468, 18.82680253904184298 ) ) ;
#13556=CARTESIAN_POINT ( 'NONE',  ( 19.62935297797556089, -3.832558109936519575, 24.50000000000000000 ) ) ;
#13558=CARTESIAN_POINT ( 'NONE',  ( 10.52132926683979974, -13.44281371605820041, 18.73743063545763121 ) ) ;
#13571=ORIENTED_EDGE ( 'NONE', *, *, #1417, .T. ) ;
#13572=EDGE_CURVE ( 'NONE', #30200, #6265, #9912, .T. ) ;
#13573=AXIS2_PLACEMENT_3D ( 'NONE', #925, #1240, #178 ) ;
#13577=CARTESIAN_POINT ( 'NONE',  ( -13.68208811019134785, -10.53240720452297374, 24.50000000000000000 ) ) ;
#13580=DIRECTION ( 'NONE',  ( -0.000000000000000000, -0.000000000000000000, 1.000000000000000000 ) ) ;
#13582=VERTEX_POINT ( 'NONE', #27564 ) ;
#13586=CARTESIAN_POINT ( 'NONE',  ( 3.728348255937731448, 16.64288108867316751, 7.603368798681074736 ) ) ;
#13589=VERTEX_POINT ( 'NONE', #3853 ) ;
#13594=VECTOR ( 'NONE', #24434, 1000.000000000000000 ) ;
#13596=CARTESIAN_POINT ( 'NONE',  ( 18.01689225005682005, -8.724154469992754457, 7.272049892295485485 ) ) ;
#13597=CARTESIAN_POINT ( 'NONE',  ( -15.64089046717303333, 12.49323067438738555, 5.749491821935610147 ) ) ;
#13598=CARTESIAN_POINT ( 'NONE',  ( 5.231931633751615074, 19.32210152104737233, 20.34789198813115263 ) ) ;
#13599=ORIENTED_EDGE ( 'NONE', *, *, #24461, .T. ) ;
#13601=DIRECTION ( 'NONE',  ( 0.9594929736144992560, 0.2817325568414232317, 0.000000000000000000 ) ) ;
#13602=ADVANCED_FACE ( 'NONE', ( #29593 ), #22559, .F. ) ;
#13605=CARTESIAN_POINT ( 'NONE',  ( -5.103338407348686268, 19.35644909001343805, 18.90679857307105749 ) ) ;
#13608=EDGE_CURVE ( 'NONE', #23147, #2256, #27714, .T. ) ;
#13612=ORIENTED_EDGE ( 'NONE', *, *, #12471, .T. ) ;
#13614=CARTESIAN_POINT ( 'NONE',  ( 1.342668813586973764, -19.95494644892924185, 6.392525840300336881 ) ) ;
#13615=CARTESIAN_POINT ( 'NONE',  ( 14.20168120032941594, 14.08243226175162555, 19.08830981656263504 ) ) ;
#13616=DIRECTION ( 'NONE',  ( 0.000000000000000000, 0.000000000000000000, 1.000000000000000000 ) ) ;
#13625=CARTESIAN_POINT ( 'NONE',  ( -19.87500762523393050, 2.235808837979145203, 20.32200205377525393 ) ) ;
#13627=CARTESIAN_POINT ( 'NONE',  ( -7.827050521741846012, 5.352643706120544742, 21.50000000000000000 ) ) ;
#13631=DIRECTION ( 'NONE',  ( -0.000000000000000000, -0.000000000000000000, 1.000000000000000000 ) ) ;
#13633=CARTESIAN_POINT ( 'NONE',  ( 1.512395753140456378, -17.00118538373299160, 5.951255046771932733 ) ) ;
#13634=ORIENTED_EDGE ( 'NONE', *, *, #30575, .T. ) ;
#13638=FACE_OUTER_BOUND ( 'NONE', #3315, .T. ) ;
#13640=DIRECTION ( 'NONE',  ( -0.000000000000000000, -0.000000000000000000, 1.000000000000000000 ) ) ;
#13641=AXIS2_PLACEMENT_3D ( 'NONE', #13710, #23196, #22594 ) ;
#13642=CARTESIAN_POINT ( 'NONE',  ( -14.87733195063809255, -8.360270151095061664, 18.56793045041961321 ) ) ;
#13646=FACE_BOUND ( 'NONE', #5407, .T. ) ;
#13650=ORIENTED_EDGE ( 'NONE', *, *, #2304, .F. ) ;
#13654=B_SPLINE_SURFACE_WITH_KNOTS ( 'NONE', 3, 1, ( 
 ( #4299, #25986 ),
 ( #11957, #30498 ),
 ( #23782, #11633 ),
 ( #4614, #30811 ),
 ( #18816, #21125 ),
 ( #26127, #18514 ),
 ( #2263, #30644 ),
 ( #7256, #18659 ),
 ( #9291, #90 ),
 ( #21289, #2114 ),
 ( #28634, #28335 ),
 ( #20836, #9000 ),
 ( #14262, #11784 ),
 ( #28014, #4471 ),
 ( #26286, #14114 ),
 ( #18974, #1819 ),
 ( #23621, #2434 ),
 ( #6646, #7112 ),
 ( #4758, #13978 ),
 ( #9607, #19116 ),
 ( #11342, #16163 ),
 ( #13829, #28164 ),
 ( #23331, #1971 ),
 ( #11493, #21601 ),
 ( #15041, #24405 ),
 ( #239, #12569 ),
 ( #542, #9750 ),
 ( #12722, #17234 ),
 ( #16932, #26920 ),
 ( #24554, #3199 ),
 ( #26759, #5390 ) ),
 .UNSPECIFIED., .F., .F., .F.,
 ( 4, 3, 3, 3, 3, 3, 3, 3, 3, 3, 4 ),
 ( 2, 2 ),
 ( 0.000000000000000000, 0.05425176834609614362, 0.1085332949128348518, 0.1623767749169379715, 0.2157504826133058717, 0.2688657508888169789, 0.3218907763505471364, 0.3749548578363334772, 0.4282048033836237666, 0.4818374082110496448, 0.4999999999131654604 ),
 ( 0.000000000000000000, 1.000000000000000000 ),
 .UNSPECIFIED. ) ;
#13658=FACE_OUTER_BOUND ( 'NONE', #16957, .T. ) ;
#13661=CARTESIAN_POINT ( 'NONE',  ( -10.39297074171569690, -17.10854403003571989, 5.661398277488802755 ) ) ;
#13662=DIRECTION ( 'NONE',  ( -0.000000000000000000, -0.000000000000000000, 1.000000000000000000 ) ) ;
#13663=FACE_OUTER_BOUND ( 'NONE', #27733, .T. ) ;
#13666=CARTESIAN_POINT ( 'NONE',  ( 16.58213327075030818, 4.067275193340576855, 6.147510495896841398 ) ) ;
#13670=DIRECTION ( 'NONE',  ( -0.000000000000000000, -0.000000000000000000, -1.000000000000000000 ) ) ;
#13672=CARTESIAN_POINT ( 'NONE',  ( 3.537840656726939592, 16.69140805415182527, 18.45571264222803975 ) ) ;
#13674=CARTESIAN_POINT ( 'NONE',  ( -18.41515300997269122, -7.848447721146241562, 19.87181966307587544 ) ) ;
#13684=DIRECTION ( 'NONE',  ( 1.000000000000000000, 0.000000000000000000, 0.000000000000000000 ) ) ;
#13687=CARTESIAN_POINT ( 'NONE',  ( -19.81665592078379490, 2.832673353242748604, 5.701226463332907279 ) ) ;
#13688=CARTESIAN_POINT ( 'NONE',  ( 15.52089561533224327, 12.61365839305099179, 6.913388067999413522 ) ) ;
#13701=FACE_OUTER_BOUND ( 'NONE', #24973, .T. ) ;
#13702=DIRECTION ( 'NONE',  ( 0.000000000000000000, 0.000000000000000000, 1.000000000000000000 ) ) ;
#13703=CARTESIAN_POINT ( 'NONE',  ( -19.88720069594608475, 2.282442057551329562, 20.32367522806703874 ) ) ;
#13705=VERTEX_POINT ( 'NONE', #1666 ) ;
#13706=CARTESIAN_POINT ( 'NONE',  ( -6.385759811051640256, 15.83451745216270901, 6.147510495896842286 ) ) ;
#13710=CARTESIAN_POINT ( 'NONE',  ( 8.999114229549594057, -0.1262659238204522361, 1.500000000000001332 ) ) ;
#13713=CARTESIAN_POINT ( 'NONE',  ( 10.16054539467770113, 13.96046037420044961, 1.500000000000000000 ) ) ;
#13723=EDGE_LOOP ( 'NONE', ( #24408, #24690 ) ) ;
#13726=DIRECTION ( 'NONE',  ( 1.000000000000000000, 0.000000000000000000, 0.000000000000000000 ) ) ;
#13727=AXIS2_PLACEMENT_3D ( 'NONE', #13135, #8301, #27332 ) ;
#13730=CARTESIAN_POINT ( 'NONE',  ( 19.85280965686022014, 2.565335765644451094, 20.12545155307891065 ) ) ;
#13732=EDGE_CURVE ( 'NONE', #21892, #14781, #25837, .T. ) ;
#13733=CARTESIAN_POINT ( 'NONE',  ( -16.87560513830565867, 2.281487909151088012, 20.12545155307891065 ) ) ;
#13736=CARTESIAN_POINT ( 'NONE',  ( 3.077027262763119442, 16.79827892558873614, 19.14333282897057842 ) ) ;
#13741=CARTESIAN_POINT ( 'NONE',  ( 14.87898868866547097, 13.36471831362575102, 18.34798005863227388 ) ) ;
#13745=EDGE_CURVE ( 'NONE', #5492, #2392, #25369, .T. ) ;
#13748=CARTESIAN_POINT ( 'NONE',  ( -19.94516883457951550, 1.701953382846943086, 6.041646659195333058 ) ) ;
#13750=LINE ( 'NONE', #16392, #8495 ) ;
#13755=DIRECTION ( 'NONE',  ( -0.9898214418809326842, 0.1423148382732851158, -0.000000000000000000 ) ) ;
#13757=VERTEX_POINT ( 'NONE', #28484 ) ;
#13758=CARTESIAN_POINT ( 'NONE',  ( -0.1522245795255685596, -19.99979613760742225, 5.775318986477954830 ) ) ;
#13760=EDGE_CURVE ( 'NONE', #15501, #26631, #9402, .T. ) ;
#13762=ADVANCED_FACE ( 'NONE', ( #16769 ), #13654, .T. ) ;
#13769=VERTEX_POINT ( 'NONE', #7735 ) ;
#13772=DIRECTION ( 'NONE',  ( 1.000000000000000000, 0.000000000000000000, 0.000000000000000000 ) ) ;
#13773=EDGE_LOOP ( 'NONE', ( #16021, #20438, #7433, #9855 ) ) ;
#13775=CARTESIAN_POINT ( 'NONE',  ( 0.000000000000000000, 0.000000000000000000, 1.500000000000001332 ) ) ;
#13776=CARTESIAN_POINT ( 'NONE',  ( -14.74412167020460274, -8.612351851578502249, 18.92976555901915603 ) ) ;
#13781=VECTOR ( 'NONE', #22029, 1000.000000000000000 ) ;
#13783=ORIENTED_EDGE ( 'NONE', *, *, #11336, .T. ) ;
#13784=DIRECTION ( 'NONE',  ( -1.000000000000000000, 0.000000000000000000, 0.000000000000000000 ) ) ;
#13786=DIRECTION ( 'NONE',  ( 0.9898214418809326842, 0.1423148382732852268, -0.000000000000000000 ) ) ;
#13788=CARTESIAN_POINT ( 'NONE',  ( -6.908049759614255159, 18.76916546752687509, 6.919864475265776527 ) ) ;
#13793=DIRECTION ( 'NONE',  ( -0.000000000000000000, -0.000000000000000000, 1.000000000000000000 ) ) ;
#13794=VERTEX_POINT ( 'NONE', #10377 ) ;
#13807=CARTESIAN_POINT ( 'NONE',  ( 11.68275852895869349, 12.45554129448069602, 19.08844262864050023 ) ) ;
#13812=CIRCLE ( 'NONE', #22282, 0.7500000000000006661 ) ;
#13813=CARTESIAN_POINT ( 'NONE',  ( -15.27573937290524242, -7.547610621728492397, 18.37259980046034258 ) ) ;
#13814=CARTESIAN_POINT ( 'NONE',  ( 0.000000000000000000, 0.000000000000000000, 1.500000000000001332 ) ) ;
#13815=CARTESIAN_POINT ( 'NONE',  ( 4.668110441710642711, -19.44758969394385062, 24.50000000000000000 ) ) ;
#13818=CARTESIAN_POINT ( 'NONE',  ( -15.26311659977723956, -7.574663188999289254, 20.32842677360128292 ) ) ;
#13820=AXIS2_PLACEMENT_3D ( 'NONE', #23100, #4692, #30286 ) ;
#13823=AXIS2_PLACEMENT_3D ( 'NONE', #27996, #15833, #30180 ) ;
#13827=VERTEX_POINT ( 'NONE', #14732 ) ;
#13829=CARTESIAN_POINT ( 'NONE',  ( 18.05613910678266976, -8.642405844459423392, 18.63641924841378028 ) ) ;
#13830=CARTESIAN_POINT ( 'NONE',  ( 4.119120293826441959, 16.53802619141620411, 5.653912893140659257 ) ) ;
#13831=AXIS2_PLACEMENT_3D ( 'NONE', #8664, #15515, #27218 ) ;
#13832=ADVANCED_FACE ( 'NONE', ( #21913 ), #8045, .F. ) ;
#13834=CARTESIAN_POINT ( 'NONE',  ( -16.81500952837178886, 2.642855143025227616, 6.530762810602277924 ) ) ;
#13835=AXIS2_PLACEMENT_3D ( 'NONE', #28386, #2636, #23988 ) ;
#13837=EDGE_CURVE ( 'NONE', #3697, #4518, #24639, .T. ) ;
#13838=VECTOR ( 'NONE', #5255, 1000.000000000000000 ) ;
#13841=ORIENTED_EDGE ( 'NONE', *, *, #29838, .F. ) ;
#13842=DIRECTION ( 'NONE',  ( 0.000000000000000000, 0.000000000000000000, 1.000000000000000000 ) ) ;
#13843=DIRECTION ( 'NONE',  ( 1.000000000000000000, 0.000000000000000000, 0.000000000000000000 ) ) ;
#13847=AXIS2_PLACEMENT_3D ( 'NONE', #20690, #20989, #30513 ) ;
#13849=DIRECTION ( 'NONE',  ( -0.9096319953545183301, -0.4154150130018863796, 0.000000000000000000 ) ) ;
#13854=CARTESIAN_POINT ( 'NONE',  ( -19.92072812706008023, 1.967956072006115331, 20.19593175699879595 ) ) ;
#13858=CARTESIAN_POINT ( 'NONE',  ( 11.81973518349029462, -16.15564139912475738, 19.89182036555910571 ) ) ;
#13863=CARTESIAN_POINT ( 'NONE',  ( 5.041560023644207966, 19.35451993181657926, 20.32200205377525393 ) ) ;
#13868=ORIENTED_EDGE ( 'NONE', *, *, #26976, .T. ) ;
#13869=CARTESIAN_POINT ( 'NONE',  ( -15.85201432996395710, 12.19518096057847600, 18.73377938172350810 ) ) ;
#13871=ORIENTED_EDGE ( 'NONE', *, *, #24998, .F. ) ;
#13877=AXIS2_PLACEMENT_3D ( 'NONE', #4328, #1844, #1995 ) ;
#13880=CARTESIAN_POINT ( 'NONE',  ( 0.7836604620899298990, -17.02735026737547841, 18.34798005863078885 ) ) ;
#13881=DIRECTION ( 'NONE',  ( -0.000000000000000000, -0.000000000000000000, 1.000000000000000000 ) ) ;
#13886=CARTESIAN_POINT ( 'NONE',  ( 10.83311381505435023, -16.83321666392360783, 7.595116371587256054 ) ) ;
#13887=CARTESIAN_POINT ( 'NONE',  ( 15.76815964721467367, -6.465453726329344342, 5.657991946698900598 ) ) ;
#13888=CARTESIAN_POINT ( 'NONE',  ( -13.43037651602832128, 10.49991632925268625, 5.652605728828375753 ) ) ;
#13889=CARTESIAN_POINT ( 'NONE',  ( 5.080682615984644990, 19.36225455879193902, 18.37415474056476938 ) ) ;
#13891=VERTEX_POINT ( 'NONE', #22836 ) ;
#13894=CARTESIAN_POINT ( 'NONE',  ( -5.557658336892892237, 19.23087281213773281, 18.44501272782439827 ) ) ;
#13899=CYLINDRICAL_SURFACE ( 'NONE', #5940, 20.00000000000000355 ) ;
#13901=CARTESIAN_POINT ( 'NONE',  ( 0.8583496426666205048, -19.98194197654538584, 7.528076282304595246 ) ) ;
#13902=CIRCLE ( 'NONE', #8451, 9.482273699623480212 ) ;
#13904=CARTESIAN_POINT ( 'NONE',  ( 19.76423196911361302, 3.064691114365034608, 20.34789198813115263 ) ) ;
#13905=ORIENTED_EDGE ( 'NONE', *, *, #16398, .F. ) ;
#13916=ADVANCED_FACE ( 'NONE', ( #1486 ), #18168, .F. ) ;
#13920=CARTESIAN_POINT ( 'NONE',  ( -19.84403786039536755, 2.492757843112275662, 5.652196082369963293 ) ) ;
#13922=CARTESIAN_POINT ( 'NONE',  ( 15.38884489568259362, -7.274072546997685684, 6.782064869129509788 ) ) ;
#13926=ORIENTED_EDGE ( 'NONE', *, *, #16050, .T. ) ;
#13929=ADVANCED_FACE ( 'NONE', ( #3815 ), #1018, .F. ) ;
#13931=ORIENTED_EDGE ( 'NONE', *, *, #20391, .T. ) ;
#13932=DIRECTION ( 'NONE',  ( 0.000000000000000000, 0.000000000000000000, 1.000000000000000000 ) ) ;
#13941=CARTESIAN_POINT ( 'NONE',  ( -20.00000000000004263, 1.387778780781445676E-14, 24.50000000000000000 ) ) ;
#13942=EDGE_CURVE ( 'NONE', #18940, #24218, #26130, .T. ) ;
#13948=EDGE_CURVE ( 'NONE', #19294, #1929, #3351, .T. ) ;
#13949=LINE ( 'NONE', #30782, #26459 ) ;
#13953=CARTESIAN_POINT ( 'NONE',  ( 1.316598178790388207, -17.01073877869967532, 20.19593175699879595 ) ) ;
#13955=EDGE_CURVE ( 'NONE', #26398, #1188, #6148, .T. ) ;
#13959=ORIENTED_EDGE ( 'NONE', *, *, #3618, .T. ) ;
#13960=CARTESIAN_POINT ( 'NONE',  ( 0.000000000000000000, 0.000000000000000000, 21.50000000000000000 ) ) ;
#13961=CARTESIAN_POINT ( 'NONE',  ( -15.57728904105048606, -6.860944617588176087, 19.21496526180053621 ) ) ;
#13962=FACE_OUTER_BOUND ( 'NONE', #29801, .T. ) ;
#13963=DIRECTION ( 'NONE',  ( 1.000000000000000000, 0.000000000000000000, 0.000000000000000000 ) ) ;
#13966=CARTESIAN_POINT ( 'NONE',  ( -15.57976790534002909, -6.855017190910953850, 19.33715507985239412 ) ) ;
#13969=EDGE_LOOP ( 'NONE', ( #10889, #4919 ) ) ;
#13973=EDGE_CURVE ( 'NONE', #23230, #4543, #1942, .T. ) ;
#13976=VERTEX_POINT ( 'NONE', #9107 ) ;
#13978=CARTESIAN_POINT ( 'NONE',  ( 15.43168774359948436, -7.187270164670358064, 18.90679857307105749 ) ) ;
#13980=CARTESIAN_POINT ( 'NONE',  ( 6.184030279945250008, 19.03884152227148263, 7.080843742048788414 ) ) ;
#13982=CARTESIAN_POINT ( 'NONE',  ( 0.1262659238204208167, 8.999114229549594057, 21.50000000000000000 ) ) ;
#13984=CARTESIAN_POINT ( 'NONE',  ( 12.13430697852917994, 11.98518526348621371, 7.603368798681074736 ) ) ;
#13985=CARTESIAN_POINT ( 'NONE',  ( 0.000000000000000000, 0.000000000000000000, 1.500000000000001332 ) ) ;
#13987=ORIENTED_EDGE ( 'NONE', *, *, #3106, .F. ) ;
#13990=CARTESIAN_POINT ( 'NONE',  ( -15.04923167492114366, -8.024232118407711667, 5.653604225791662330 ) ) ;
#13992=CARTESIAN_POINT ( 'NONE',  ( -15.01515151829604910, 13.21212483861245168, 5.775318986477952166 ) ) ;
#13994=CARTESIAN_POINT ( 'NONE',  ( 16.83255095305771931, 2.584307790367077029, 18.54473042795394022 ) ) ;
#13997=CARTESIAN_POINT ( 'NONE',  ( -5.687793815610304726, 6.974883619896852238, 1.500000000000001332 ) ) ;
#13999=CYLINDRICAL_SURFACE ( 'NONE', #25944, 0.7499999999999988898 ) ;
#14004=CARTESIAN_POINT ( 'NONE',  ( 10.69227409735889722, -13.31703061742498306, 19.36813350477385143 ) ) ;
#14014=DIRECTION ( 'NONE',  ( 0.000000000000000000, 0.000000000000000000, 1.000000000000000000 ) ) ;
#14015=CARTESIAN_POINT ( 'NONE',  ( 0.000000000000000000, 0.000000000000000000, 21.50000000000000000 ) ) ;
#14022=DIRECTION ( 'NONE',  ( -1.000000000000000000, 0.000000000000000000, 0.000000000000000000 ) ) ;
#14025=CARTESIAN_POINT ( 'NONE',  ( -14.79998981349582721, -8.507912210612349924, 18.73314399819311404 ) ) ;
#14026=DIRECTION ( 'NONE',  ( 1.000000000000000000, 0.000000000000000000, 0.000000000000000000 ) ) ;
#14028=EDGE_LOOP ( 'NONE', ( #4938, #15585, #6303, #22663 ) ) ;
#14031=CARTESIAN_POINT ( 'NONE',  ( -13.51981801095249658, 10.39108251695558138, 7.627891251804737927 ) ) ;
#14032=LINE ( 'NONE', #9664, #26778 ) ;
#14033=ORIENTED_EDGE ( 'NONE', *, *, #26906, .F. ) ;
#14041=ORIENTED_EDGE ( 'NONE', *, *, #30549, .F. ) ;
#14042=CARTESIAN_POINT ( 'NONE',  ( -17.05413688332568967, 0.7966627085705102473, 7.196036389296800451 ) ) ;
#14043=CARTESIAN_POINT ( 'NONE',  ( 6.187077094091595342, 11.47693674426096599, 1.500000000000001332 ) ) ;
#14048=CARTESIAN_POINT ( 'NONE',  ( 15.98815986143407208, -5.948957736846856470, 5.749491821935610147 ) ) ;
#14050=ORIENTED_EDGE ( 'NONE', *, *, #30356, .T. ) ;
#14056=CYLINDRICAL_SURFACE ( 'NONE', #884, 10.00000000000000000 ) ;
#14064=CARTESIAN_POINT ( 'NONE',  ( -14.75084321123810938, -8.599826344683139112, 19.79423548914561692 ) ) ;
#14066=( LENGTH_UNIT ( ) NAMED_UNIT ( * ) SI_UNIT ( .MILLI., .METRE. ) );
#14069=CARTESIAN_POINT ( 'NONE',  ( -12.86767874445213877, -1.850092897552710225, 1.500000000000001332 ) ) ;
#14071=CIRCLE ( 'NONE', #28097, 9.482273699623480212 ) ;
#14074=CARTESIAN_POINT ( 'NONE',  ( -4.622016212553093695, -12.19167610014704906, 24.50000000000000000 ) ) ;
#14076=ORIENTED_EDGE ( 'NONE', *, *, #3520, .F. ) ;
#14080=ORIENTED_EDGE ( 'NONE', *, *, #26331, .T. ) ;
#14084=CARTESIAN_POINT ( 'NONE',  ( 0.1277494853664046803, -20.01772078232906438, 18.36582235739946611 ) ) ;
#14085=CARTESIAN_POINT ( 'NONE',  ( -8.550548368345317840, -14.74545326172987103, 7.652108011868850035 ) ) ;
#14086=DIRECTION ( 'NONE',  ( -0.000000000000000000, -0.000000000000000000, 1.000000000000000000 ) ) ;
#14087=CARTESIAN_POINT ( 'NONE',  ( 0.9279538312821433710, -17.02439129904410464, 20.33971507717571114 ) ) ;
#14090=AXIS2_PLACEMENT_3D ( 'NONE', #20166, #26898, #5518 ) ;
#14091=CARTESIAN_POINT ( 'NONE',  ( 2.703030265324084080, -12.75514121382991384, 1.500000000000001332 ) ) ;
#14092=CARTESIAN_POINT ( 'NONE',  ( 11.70346162051516359, 12.43461153239107730, 19.69140814234746273 ) ) ;
#14095=AXIS2_PLACEMENT_3D ( 'NONE', #6104, #8753, #27175 ) ;
#14096=CARTESIAN_POINT ( 'NONE',  ( -15.57738559309032489, -6.860713375568480821, 19.41069149716888020 ) ) ;
#14097=DIRECTION ( 'NONE',  ( 0.9096319953545183301, 0.4154150130018865461, 0.000000000000000000 ) ) ;
#14099=CARTESIAN_POINT ( 'NONE',  ( 4.049916833591939103, 16.55712665779026693, 20.34789198813115263 ) ) ;
#14101=AXIS2_PLACEMENT_3D ( 'NONE', #16128, #23287, #1931 ) ;
#14102=ADVANCED_FACE ( 'NONE', ( #30318, #8964 ), #18480, .T. ) ;
#14113=AXIS2_PLACEMENT_3D ( 'NONE', #9439, #9729, #21262 ) ;
#14114=CARTESIAN_POINT ( 'NONE',  ( 15.38325456941028868, -7.285321374151285667, 19.33715507985239412 ) ) ;
#14115=EDGE_CURVE ( 'NONE', #21119, #17125, #11455, .T. ) ;
#14116=CARTESIAN_POINT ( 'NONE',  ( 4.964892671625814380, 16.28226395658652237, 6.310736198168394928 ) ) ;
#14121=CARTESIAN_POINT ( 'NONE',  ( 11.70346162051517780, 12.43461153239108441, 6.995624166085161910 ) ) ;
#14122=CARTESIAN_POINT ( 'NONE',  ( -4.622016212553093695, -12.19167610014704906, 1.500000000000001332 ) ) ;
#14125=DIRECTION ( 'NONE',  ( -0.000000000000000000, -0.000000000000000000, 1.000000000000000000 ) ) ;
#14127=CARTESIAN_POINT ( 'NONE',  ( -7.028330626922778990, 10.93629592680536788, 24.50000000000000000 ) ) ;
#14129=CARTESIAN_POINT ( 'NONE',  ( -18.46504858183722675, -7.730374101464832393, 6.420335371522007506 ) ) ;
#14132=DIRECTION ( 'NONE',  ( 1.000000000000000000, 0.000000000000000000, 0.000000000000000000 ) ) ;
#14133=EDGE_CURVE ( 'NONE', #18371, #29096, #24139, .T. ) ;
#14135=B_SPLINE_SURFACE_WITH_KNOTS ( 'NONE', 3, 1, ( 
 ( #24626, #19794 ),
 ( #8114, #17621 ),
 ( #21667, #7494 ),
 ( #15254, #24786 ),
 ( #5142, #304 ),
 ( #28863, #16992 ),
 ( #24156, #12327 ),
 ( #9987, #25097 ),
 ( #10751, #22903 ),
 ( #1405, #1245 ),
 ( #20564, #20262 ),
 ( #15580, #29787 ),
 ( #8263, #18406 ),
 ( #15902, #8429 ),
 ( #15420, #16045 ),
 ( #12949, #11063 ),
 ( #17939, #27911 ),
 ( #27448, #25415 ),
 ( #1552, #25249 ),
 ( #11210, #6069 ),
 ( #10918, #13257 ),
 ( #20112, #22595 ),
 ( #3740, #1695 ),
 ( #22746, #20421 ),
 ( #29942, #6536 ),
 ( #30237, #24942 ),
 ( #8579, #18085 ),
 ( #27602, #6224 ),
 ( #20707, #15731 ),
 ( #25561, #30086 ),
 ( #22442, #8882 ) ),
 .UNSPECIFIED., .F., .F., .F.,
 ( 4, 3, 3, 3, 3, 3, 3, 3, 3, 3, 4 ),
 ( 2, 2 ),
 ( 0.000000000000000000, 0.05425176834609633791, 0.1085332949128352958, 0.1623767749169382768, 0.2157504826133063158, 0.2688657508888171455, 0.3218907763505476360, 0.3749548578363336993, 0.4282048033836242107, 0.4818374082110501444, 0.4999999999131656825 ),
 ( 0.000000000000000000, 1.000000000000000000 ),
 .UNSPECIFIED. ) ;
#14141=DIRECTION ( 'NONE',  ( 1.000000000000000000, 0.000000000000000000, 0.000000000000000000 ) ) ;
#14143=ORIENTED_EDGE ( 'NONE', *, *, #27858, .F. ) ;
#14145=CARTESIAN_POINT ( 'NONE',  ( 10.22519205257000507, -13.65449557370668465, 20.25542030744407640 ) ) ;
#14146=CARTESIAN_POINT ( 'NONE',  ( -4.622016212553093695, -12.19167610014704906, 1.500000000000001332 ) ) ;
#14148=ORIENTED_EDGE ( 'NONE', *, *, #9470, .T. ) ;
#14151=EDGE_CURVE ( 'NONE', #2092, #2473, #13218, .T. ) ;
#14156=CARTESIAN_POINT ( 'NONE',  ( 16.13887868878509479, -5.569097860077073747, 19.89182036555910571 ) ) ;
#14157=CARTESIAN_POINT ( 'NONE',  ( 19.57650873258266344, 4.179294809495488039, 19.14333282897057842 ) ) ;
#14158=DIRECTION ( 'NONE',  ( -0.000000000000000000, -0.000000000000000000, 1.000000000000000000 ) ) ;
#14164=ORIENTED_EDGE ( 'NONE', *, *, #30202, .F. ) ;
#14168=CARTESIAN_POINT ( 'NONE',  ( 0.7788148816922458861, -17.02744011591804707, 20.34789198813115263 ) ) ;
#14169=CARTESIAN_POINT ( 'NONE',  ( 0.3493067888074735117, -20.01473451864462305, 7.652108011868850035 ) ) ;
#14170=CARTESIAN_POINT ( 'NONE',  ( -14.58213539500865785, 7.758783772730382111, 1.500000000000000000 ) ) ;
#14172=DIRECTION ( 'NONE',  ( 1.000000000000000000, 0.000000000000000000, 0.000000000000000000 ) ) ;
#14174=CARTESIAN_POINT ( 'NONE',  ( 10.92346103252092604, -16.77505673787611329, 7.632642797338977658 ) ) ;
#14176=CARTESIAN_POINT ( 'NONE',  ( -13.65791587866001855, 10.22062306005669363, 7.559636331181775581 ) ) ;
#14177=LINE ( 'NONE', #2800, #4851 ) ;
#14179=ORIENTED_EDGE ( 'NONE', *, *, #19079, .F. ) ;
#14182=FACE_OUTER_BOUND ( 'NONE', #6989, .T. ) ;
#14185=CARTESIAN_POINT ( 'NONE',  ( 12.35522425158189108, 11.74279415389956505, 5.652196082368482699 ) ) ;
#14190=CARTESIAN_POINT ( 'NONE',  ( -19.95113275051131652, 1.631914050426796159, 6.131018562779544823 ) ) ;
#14195=ORIENTED_EDGE ( 'NONE', *, *, #10591, .T. ) ;
#14197=CARTESIAN_POINT ( 'NONE',  ( 18.52707432543149579, -7.580618987226253935, 5.749491821935610147 ) ) ;
#14199=CARTESIAN_POINT ( 'NONE',  ( -2.959227181723746547, 8.499586724479465616, 1.500000000000001332 ) ) ;
#14203=CARTESIAN_POINT ( 'NONE',  ( 10.58819075803338450, -13.39403179698972934, 18.84329447212443753 ) ) ;
#14205=CARTESIAN_POINT ( 'NONE',  ( -10.62409560796092833, -16.94539057243558489, 5.651480102388687143 ) ) ;
#14214=CARTESIAN_POINT ( 'NONE',  ( -17.99620775894062419, -8.766556869501986426, 20.33971507717571114 ) ) ;
#14216=CARTESIAN_POINT ( 'NONE',  ( 4.172444469722463189, 16.52351170763985877, 5.651492010659114662 ) ) ;
#14217=CYLINDRICAL_SURFACE ( 'NONE', #22564, 9.482273699623480212 ) ;
#14225=CIRCLE ( 'NONE', #10754, 0.7500000000000002220 ) ;
#14226=ORIENTED_EDGE ( 'NONE', *, *, #11106, .T. ) ;
#14227=DIRECTION ( 'NONE',  ( 0.000000000000000000, 0.000000000000000000, 1.000000000000000000 ) ) ;
#14230=ORIENTED_EDGE ( 'NONE', *, *, #4837, .F. ) ;
#14232=VERTEX_POINT ( 'NONE', #17040 ) ;
#14234=CARTESIAN_POINT ( 'NONE',  ( 0.3346962451677067962, -17.03061174119336840, 20.25336174263950184 ) ) ;
#14235=DIRECTION ( 'NONE',  ( 1.000000000000000000, 0.000000000000000000, 0.000000000000000000 ) ) ;
#14236=CARTESIAN_POINT ( 'NONE',  ( 1.265447379378154436, -19.97763032565216790, 19.79423548914561692 ) ) ;
#14238=CARTESIAN_POINT ( 'NONE',  ( 18.57699708025013052, -7.409721753143990952, 5.853797745100183469 ) ) ;
#14241=CARTESIAN_POINT ( 'NONE',  ( 14.30907656312162679, 13.99861481489062598, 19.89182036555910571 ) ) ;
#14242=VERTEX_POINT ( 'NONE', #26566 ) ;
#14243=CIRCLE ( 'NONE', #14319, 0.7500000000000024425 ) ;
#14244=VECTOR ( 'NONE', #29374, 1000.000000000000227 ) ;
#14246=CARTESIAN_POINT ( 'NONE',  ( -17.59781475975453446, -9.540531696329381361, 6.560937769032974209 ) ) ;
#14247=CARTESIAN_POINT ( 'NONE',  ( 12.24063095261064404, 4.490763173670002217, 1.500000000000001332 ) ) ;
#14248=CARTESIAN_POINT ( 'NONE',  ( -19.90071050938331609, 1.994113959836041783, 7.528076282304594358 ) ) ;
#14250=CARTESIAN_POINT ( 'NONE',  ( -15.34842816977634428, -7.387654668753816267, 18.44501272782439827 ) ) ;
#14252=CIRCLE ( 'NONE', #27705, 0.7500000000000006661 ) ;
#14259=CARTESIAN_POINT ( 'NONE',  ( 11.83518757993566695, -16.12237520560631765, 18.84486140012300481 ) ) ;
#14260=ORIENTED_EDGE ( 'NONE', *, *, #4183, .T. ) ;
#14262=CARTESIAN_POINT ( 'NONE',  ( 17.93514094173302453, -8.890850898656898593, 19.56050940960062690 ) ) ;
#14264=CARTESIAN_POINT ( 'NONE',  ( 4.159666964149448809, 16.52698801271858287, 7.652108011868850035 ) ) ;
#14267=ORIENTED_EDGE ( 'NONE', *, *, #68, .F. ) ;
#14268=CARTESIAN_POINT ( 'NONE',  ( 4.917955972067796111, 16.29747060413736648, 18.90679857307105749 ) ) ;
#14269=LINE ( 'NONE', #9462, #778 ) ;
#14271=DIRECTION ( 'NONE',  ( -0.000000000000000000, -0.000000000000000000, 1.000000000000000000 ) ) ;
#14273=ORIENTED_EDGE ( 'NONE', *, *, #21531, .T. ) ;
#14276=DIRECTION ( 'NONE',  ( 0.000000000000000000, 0.000000000000000000, 1.000000000000000000 ) ) ;
#14280=CARTESIAN_POINT ( 'NONE',  ( -15.16517292768934411, -7.781889190071454188, 7.652108011868850035 ) ) ;
#14283=CARTESIAN_POINT ( 'NONE',  ( -0.6606983433884106027, -20.00701505202155417, 6.755862304746362845 ) ) ;
#14284=CIRCLE ( 'NONE', #3845, 1.000000000000004441 ) ;
#14287=ADVANCED_FACE ( 'NONE', ( #17984 ), #12989, .F. ) ;
#14289=CARTESIAN_POINT ( 'NONE',  ( -16.97424920726489006, 1.578583718960127280, 20.34789198813115263 ) ) ;
#14292=CARTESIAN_POINT ( 'NONE',  ( 10.64246886845954521, -13.35396698543973137, 19.69140814234746273 ) ) ;
#14294=ORIENTED_EDGE ( 'NONE', *, *, #25998, .T. ) ;
#14295=ORIENTED_EDGE ( 'NONE', *, *, #9142, .F. ) ;
#14301=AXIS2_PLACEMENT_3D ( 'NONE', #26868, #12519, #10160 ) ;
#14302=CARTESIAN_POINT ( 'NONE',  ( 15.31432103507273546, 12.89133701742166949, 20.12545155307891065 ) ) ;
#14303=B_SPLINE_CURVE_WITH_KNOTS ( 'NONE', 3,
 ( #1102, #17634, #22454, #6081, #11076, #13116, #27307, #10934, #6238, #17953, #10613, #27462, #22609, #29337, #15744, #25265 ),
 .UNSPECIFIED., .F., .F.,
 ( 4, 2, 2, 2, 2, 2, 2, 4 ),
 ( 0.5000000000000000000, 0.6250000000000017764, 0.6875000000000025535, 0.7187500000000028866, 0.7500000000000033307, 0.8125000000000022204, 0.8750000000000013323, 1.000000000000000000 ),
 .UNSPECIFIED. ) ;
#14304=EDGE_CURVE ( 'NONE', #30200, #19542, #17062, .T. ) ;
#14305=CARTESIAN_POINT ( 'NONE',  ( -8.550548368345317840, -14.74545326172986925, 7.652108011868850035 ) ) ;
#14308=EDGE_CURVE ( 'NONE', #466, #3526, #7624, .T. ) ;
#14309=CARTESIAN_POINT ( 'NONE',  ( 18.56338958360293390, -7.490577753534553018, 18.50655187082627862 ) ) ;
#14310=CARTESIAN_POINT ( 'NONE',  ( 16.58472157312808193, 4.055073576757204812, 18.82680253904184298 ) ) ;
#14315=CIRCLE ( 'NONE', #13847, 0.7499999999999997780 ) ;
#14316=CARTESIAN_POINT ( 'NONE',  ( 15.38611090871061293, -7.279566334535328309, 19.21496526180054332 ) ) ;
#14317=ORIENTED_EDGE ( 'NONE', *, *, #4787, .F. ) ;
#14319=AXIS2_PLACEMENT_3D ( 'NONE', #19697, #5826, #24854 ) ;
#14328=AXIS2_PLACEMENT_3D ( 'NONE', #5413, #9774, #19291 ) ;
#14329=CARTESIAN_POINT ( 'NONE',  ( 1.365674945463512424, -19.97097327164667391, 6.672349528511551497 ) ) ;
#14331=CARTESIAN_POINT ( 'NONE',  ( -14.70620249426369242, -8.682611668020191686, 19.21769074125272425 ) ) ;
#14337=VECTOR ( 'NONE', #13191, 1000.000000000000114 ) ;
#14338=CARTESIAN_POINT ( 'NONE',  ( -15.69442553397265883, 12.42550873695621938, 7.500147780736496017 ) ) ;
#14342=VECTOR ( 'NONE', #9086, 1000.000000000000000 ) ;
#14346=FACE_OUTER_BOUND ( 'NONE', #9070, .T. ) ;
#14352=VERTEX_POINT ( 'NONE', #10642 ) ;
#14354=AXIS2_PLACEMENT_3D ( 'NONE', #7275, #257, #28957 ) ;
#14357=CARTESIAN_POINT ( 'NONE',  ( -17.81964242321468461, -9.081580984160163794, 20.22386025856690139 ) ) ;
#14361=CARTESIAN_POINT ( 'NONE',  ( 15.45595318746689095, 12.72131790141721375, 6.111214848085761986 ) ) ;
#14366=AXIS2_PLACEMENT_3D ( 'NONE', #7809, #24337, #12503 ) ;
#14368=ORIENTED_EDGE ( 'NONE', *, *, #11276, .F. ) ;
#14372=CARTESIAN_POINT ( 'NONE',  ( 10.52561254568492011, -13.43997246243151267, 19.96568007040468729 ) ) ;
#14383=EDGE_LOOP ( 'NONE', ( #10919, #30106 ) ) ;
#14384=DIRECTION ( 'NONE',  ( -1.000000000000000000, 0.000000000000000000, 0.000000000000000000 ) ) ;
#14387=EDGE_CURVE ( 'NONE', #15666, #4693, #23202, .T. ) ;
#14388=DIRECTION ( 'NONE',  ( 1.000000000000000000, 0.000000000000000000, 0.000000000000000000 ) ) ;
#14390=CARTESIAN_POINT ( 'NONE',  ( -5.738360882150000286, -7.548823014270624299, 13.00000000000000178 ) ) ;
#14392=ORIENTED_EDGE ( 'NONE', *, *, #3093, .F. ) ;
#14396=EDGE_LOOP ( 'NONE', ( #7217, #16049, #15687, #21885 ) ) ;
#14402=DIRECTION ( 'NONE',  ( 1.000000000000000000, 0.000000000000000000, 0.000000000000000000 ) ) ;
#14404=ORIENTED_EDGE ( 'NONE', *, *, #45, .F. ) ;
#14406=ORIENTED_EDGE ( 'NONE', *, *, #19646, .T. ) ;
#14412=CARTESIAN_POINT ( 'NONE',  ( 0.2396382576306451684, -20.01636569787184783, 18.35377592296120497 ) ) ;
#14414=DIRECTION ( 'NONE',  ( 1.000000000000000000, 0.000000000000000000, 0.000000000000000000 ) ) ;
#14415=AXIS2_PLACEMENT_3D ( 'NONE', #29403, #20179, #6000 ) ;
#14416=CARTESIAN_POINT ( 'NONE',  ( 1.000541756189970544, -17.02230863066393241, 20.32367522806703874 ) ) ;
#14419=PLANE ( 'NONE',  #26316 ) ;
#14420=CARTESIAN_POINT ( 'NONE',  ( 14.40720023010962336, 13.89764844773314678, 20.06253562465620632 ) ) ;
#14423=AXIS2_PLACEMENT_3D ( 'NONE', #18454, #9383, #28410 ) ;
#14424=CARTESIAN_POINT ( 'NONE',  ( -2.094186647214681063, 9.248129367672087042, 21.50000000000000000 ) ) ;
#14425=CARTESIAN_POINT ( 'NONE',  ( -14.70315170625143075, -8.688231105434647716, 6.672349528511551497 ) ) ;
#14426=CARTESIAN_POINT ( 'NONE',  ( -6.493275194760118829, 15.79517802630852152, 6.447548852708279377 ) ) ;
#14427=CARTESIAN_POINT ( 'NONE',  ( -19.86062922652984142, 2.360743482685565997, 5.652912763329822177 ) ) ;
#14430=DIRECTION ( 'NONE',  ( -0.000000000000000000, -0.000000000000000000, 1.000000000000000000 ) ) ;
#14435=CARTESIAN_POINT ( 'NONE',  ( -15.35487586320816078, 12.84287697592353084, 7.652108011868850035 ) ) ;
#14440=DIRECTION ( 'NONE',  ( 0.4154150130018859910, 0.9096319953545186632, 0.000000000000000000 ) ) ;
#14441=CARTESIAN_POINT ( 'NONE',  ( 5.627515464934154110, 19.21053377385552707, 7.595116371587256054 ) ) ;
#14442=ORIENTED_EDGE ( 'NONE', *, *, #20194, .T. ) ;
#14443=CARTESIAN_POINT ( 'NONE',  ( 6.275630943545793983, 19.00876817605120195, 19.33715507985239412 ) ) ;
#14444=DIRECTION ( 'NONE',  ( 0.000000000000000000, 0.000000000000000000, -1.000000000000000000 ) ) ;
#14446=DIRECTION ( 'NONE',  ( -0.9096319953545185522, 0.4154150130018859355, 0.000000000000000000 ) ) ;
#14448=VERTEX_POINT ( 'NONE', #8470 ) ;
#14454=DIRECTION ( 'NONE',  ( 0.000000000000000000, 0.000000000000000000, -1.000000000000000000 ) ) ;
#14455=LINE ( 'NONE', #21621, #22751 ) ;
#14456=CARTESIAN_POINT ( 'NONE',  ( 0.7836603915001320031, -17.02734626464551226, 5.652196082367002994 ) ) ;
#14461=ORIENTED_EDGE ( 'NONE', *, *, #18735, .T. ) ;
#14462=DIRECTION ( 'NONE',  ( -0.000000000000000000, -0.000000000000000000, 1.000000000000000000 ) ) ;
#14465=VERTEX_POINT ( 'NONE', #17974 ) ;
#14466=CARTESIAN_POINT ( 'NONE',  ( 5.169584817211992700, 19.32078214751397738, 20.34789198813115618 ) ) ;
#14468=( NAMED_UNIT ( * ) SI_UNIT ( $, .STERADIAN. ) SOLID_ANGLE_UNIT ( ) );
#14470=DIRECTION ( 'NONE',  ( 0.5406408174555974444, 0.8412535328311813165, 0.000000000000000000 ) ) ;
#14473=CARTESIAN_POINT ( 'NONE',  ( 18.63200854944940232, -7.318485330915432741, 18.64703902303423178 ) ) ;
#14474=CARTESIAN_POINT ( 'NONE',  ( 16.71770988170261063, 3.349230485916621980, 18.35718225375110180 ) ) ;
#14476=DIRECTION ( 'NONE',  ( -1.000000000000000000, 0.000000000000000000, 0.000000000000000000 ) ) ;
#14479=ORIENTED_EDGE ( 'NONE', *, *, #26181, .T. ) ;
#14482=DIRECTION ( 'NONE',  ( 0.000000000000000000, 0.000000000000000000, -1.000000000000000000 ) ) ;
#14483=DIRECTION ( 'NONE',  ( -0.9898214418809326842, -0.1423148382732852824, 0.000000000000000000 ) ) ;
#14484=DIRECTION ( 'NONE',  ( -0.000000000000000000, -0.000000000000000000, -1.000000000000000000 ) ) ;
#14489=EDGE_CURVE ( 'NONE', #4417, #26711, #6864, .T. ) ;
#14491=CARTESIAN_POINT ( 'NONE',  ( -19.71314312682348913, 3.479754436677866547, 19.11611934778430921 ) ) ;
#14492=CARTESIAN_POINT ( 'NONE',  ( 18.32239734440382151, -8.062462575157594458, 5.653912893140659257 ) ) ;
#14495=DIRECTION ( 'NONE',  ( 0.000000000000000000, 0.000000000000000000, -1.000000000000000000 ) ) ;
#14504=CARTESIAN_POINT ( 'NONE',  ( -5.475907499891252250, 16.13963752243574490, 18.34969686940295830 ) ) ;
#14507=CARTESIAN_POINT ( 'NONE',  ( -5.001173922442003317, 19.36461358832317359, 6.518927109361842831 ) ) ;
#14509=VERTEX_POINT ( 'NONE', #23540 ) ;
#14512=CARTESIAN_POINT ( 'NONE',  ( -17.98703099176682230, -8.745510052321845862, 20.34789198813115618 ) ) ;
#14516=CARTESIAN_POINT ( 'NONE',  ( 12.94832566568966037, 11.05145698499350004, 6.211014596808754007 ) ) ;
#14518=FACE_OUTER_BOUND ( 'NONE', #23127, .T. ) ;
#14519=UNCERTAINTY_MEASURE_WITH_UNIT (LENGTH_MEASURE( 1.000000000000000082E-05 ), #14066, 'distance_accuracy_value', 'NONE');
#14524=CARTESIAN_POINT ( 'NONE',  ( -5.130938270761550513, 7.974144905643841597, 1.500000000000001332 ) ) ;
#14526=CARTESIAN_POINT ( 'NONE',  ( -18.40581374043506457, -7.824871006739531509, 6.144783687052511212 ) ) ;
#14527=CARTESIAN_POINT ( 'NONE',  ( -10.73477556097085461, -16.87541441043898516, 5.676722608126685721 ) ) ;
#14529=EDGE_CURVE ( 'NONE', #23663, #17274, #29070, .T. ) ;
#14531=ADVANCED_FACE ( 'NONE', ( #14182 ), #4989, .F. ) ;
#14537=VERTEX_POINT ( 'NONE', #18884 ) ;
#14539=CARTESIAN_POINT ( 'NONE',  ( -17.67332396526446914, -9.400239829055450969, 19.89182036555910571 ) ) ;
#14540=DIRECTION ( 'NONE',  ( -0.000000000000000000, -0.000000000000000000, 1.000000000000000000 ) ) ;
#14546=EDGE_CURVE ( 'NONE', #3669, #21410, #4679, .T. ) ;
#14547=DIRECTION ( 'NONE',  ( 0.000000000000000000, 0.000000000000000000, 1.000000000000000000 ) ) ;
#14553=ORIENTED_EDGE ( 'NONE', *, *, #5364, .F. ) ;
#14555=FACE_OUTER_BOUND ( 'NONE', #9498, .T. ) ;
#14561=VERTEX_POINT ( 'NONE', #2804 ) ;
#14562=CARTESIAN_POINT ( 'NONE',  ( 0.01267125088587655463, -20.01782649599895336, 20.29090034784956131 ) ) ;
#14565=CARTESIAN_POINT ( 'NONE',  ( -9.785592877189483119, -17.46290528139147469, 7.196036389296800451 ) ) ;
#14566=EDGE_CURVE ( 'NONE', #540, #26699, #22441, .T. ) ;
#14567=CARTESIAN_POINT ( 'NONE',  ( 4.989870534563210391, 16.27408959345712347, 19.08155846658118904 ) ) ;
#14571=CARTESIAN_POINT ( 'NONE',  ( 0.8583496426666220591, -19.98194197654537874, 20.22386025856689429 ) ) ;
#14575=CARTESIAN_POINT ( 'NONE',  ( -14.77047757180930176, -8.563270617688839792, 6.131018562779544823 ) ) ;
#14576=APPLICATION_CONTEXT ( 'automotive_design' ) ;
#14577=DIRECTION ( 'NONE',  ( 0.6548607339452855447, 0.7557495743542579358, 0.000000000000000000 ) ) ;
#14582=CARTESIAN_POINT ( 'NONE',  ( -15.25992540518562279, -7.581593484474005606, 18.36582235739946611 ) ) ;
#14587=CARTESIAN_POINT ( 'NONE',  ( -5.723804255145591213, 19.16384832744316213, 18.37250658438899009 ) ) ;
#14588=CARTESIAN_POINT ( 'NONE',  ( -13.09005700315871579, 10.89973235955167929, 7.557577766377196582 ) ) ;
#14591=CARTESIAN_POINT ( 'NONE',  ( 16.01701959592644897, -5.879758784403577465, 20.24143955528809258 ) ) ;
#14592=DIRECTION ( 'NONE',  ( 0.000000000000000000, 0.000000000000000000, -1.000000000000000000 ) ) ;
#14593=ORIENTED_EDGE ( 'NONE', *, *, #17979, .F. ) ;
#14594=CARTESIAN_POINT ( 'NONE',  ( 4.744089322959553101, 16.35312844164164048, 20.05479082170252525 ) ) ;
#14595=CARTESIAN_POINT ( 'NONE',  ( 14.74830145734718734, 13.53506178006322713, 7.627891251804737927 ) ) ;
#14599=FACE_OUTER_BOUND ( 'NONE', #21521, .T. ) ;
#14601=EDGE_CURVE ( 'NONE', #14763, #7727, #14804, .T. ) ;
#14602=AXIS2_PLACEMENT_3D ( 'NONE', #22974, #13022, #1313 ) ;
#14606=FACE_OUTER_BOUND ( 'NONE', #11083, .T. ) ;
#14609=CARTESIAN_POINT ( 'NONE',  ( 14.88222593340885958, 13.36111339922579155, 7.652108011868850035 ) ) ;
#14616=CARTESIAN_POINT ( 'NONE',  ( -4.163336342344337027E-14, 1.387778780781445676E-14, 24.50000000000000000 ) ) ;
#14618=FACE_OUTER_BOUND ( 'NONE', #26828, .T. ) ;
#14619=VERTEX_POINT ( 'NONE', #24783 ) ;
#14621=VECTOR ( 'NONE', #7493, 1000.000000000000000 ) ;
#14624=AXIS2_PLACEMENT_3D ( 'NONE', #15773, #17658, #24667 ) ;
#14626=ORIENTED_EDGE ( 'NONE', *, *, #28513, .T. ) ;
#14630=DIRECTION ( 'NONE',  ( 0.9594929736144951482, -0.2817325568414371095, 0.000000000000000000 ) ) ;
#14631=CARTESIAN_POINT ( 'NONE',  ( 16.66634534075877028, 3.639270104310703857, 18.44527579819791185 ) ) ;
#14637=AXIS2_PLACEMENT_3D ( 'NONE', #20723, #15751, #25271 ) ;
#14639=CARTESIAN_POINT ( 'NONE',  ( -6.495433978329089086, 18.93455902173412397, 18.50655187082627862 ) ) ;
#14640=CARTESIAN_POINT ( 'NONE',  ( -17.81964242321468816, -9.081580984160151360, 7.528076282304601463 ) ) ;
#14641=CARTESIAN_POINT ( 'NONE',  ( -8.353478261420260509, -14.86569112999328368, 18.37415474056476938 ) ) ;
#14645=ORIENTED_EDGE ( 'NONE', *, *, #25056, .F. ) ;
#14646=CARTESIAN_POINT ( 'NONE',  ( 9.195964344571802229, -14.32884674914071965, 6.018569869498933578 ) ) ;
#14648=CARTESIAN_POINT ( 'NONE',  ( 2.352830851074111163, 9.185733585337919394, 1.500000000000001332 ) ) ;
#14653=FACE_OUTER_BOUND ( 'NONE', #25572, .T. ) ;
#14654=PLANE ( 'NONE',  #17611 ) ;
#14656=CARTESIAN_POINT ( 'NONE',  ( 2.810445847081854964, 9.056208293496318618, 13.00000000000000178 ) ) ;
#14657=EDGE_LOOP ( 'NONE', ( #10970, #5288 ) ) ;
#14660=DIRECTION ( 'NONE',  ( 1.000000000000000000, 0.000000000000000000, 0.000000000000000000 ) ) ;
#14663=CARTESIAN_POINT ( 'NONE',  ( 15.53792925084563059, 12.62098510012954478, 6.864725433338323413 ) ) ;
#14666=DIRECTION ( 'NONE',  ( -1.000000000000000000, 0.000000000000000000, 0.000000000000000000 ) ) ;
#14667=CARTESIAN_POINT ( 'NONE',  ( 16.74328841314636662, 3.194145055459935545, 20.34789198813115263 ) ) ;
#14673=CARTESIAN_POINT ( 'NONE',  ( -18.37726663805288041, -7.892083924814681239, 7.267242832833947119 ) ) ;
#14675=CARTESIAN_POINT ( 'NONE',  ( 10.74273727477993567, -16.89139546617318999, 20.25336174263950184 ) ) ;
#14678=LINE ( 'NONE', #5326, #24254 ) ;
#14679=EDGE_CURVE ( 'NONE', #681, #8511, #929, .T. ) ;
#14684=CARTESIAN_POINT ( 'NONE',  ( -15.06839649859470853, -7.981447355247936137, 20.32367522806703874 ) ) ;
#14685=CARTESIAN_POINT ( 'NONE',  ( 15.43499236066653779, -3.229500095980124996, 24.50000000000000000 ) ) ;
#14686=CARTESIAN_POINT ( 'NONE',  ( -14.81308450742032434, 13.43805957489523095, 19.96302680909624527 ) ) ;
#14687=CARTESIAN_POINT ( 'NONE',  ( 4.533306948338779563, 16.41820958405255837, 5.774779864094946369 ) ) ;
#14691=CARTESIAN_POINT ( 'NONE',  ( 19.69983030747900443, 3.454193845114027273, 7.626218077512941562 ) ) ;
#14694=ORIENTED_EDGE ( 'NONE', *, *, #8648, .F. ) ;
#14695=DIRECTION ( 'NONE',  ( 1.000000000000000000, 0.000000000000000000, 0.000000000000000000 ) ) ;
#14696=CARTESIAN_POINT ( 'NONE',  ( 4.668110441710642711, -19.44758969394385062, 24.50000000000000000 ) ) ;
#14705=CARTESIAN_POINT ( 'NONE',  ( -0.5567245496722531550, -20.01015347392404209, 18.90679857307105749 ) ) ;
#14707=EDGE_CURVE ( 'NONE', #27782, #18935, #19521, .T. ) ;
#14708=CYLINDRICAL_SURFACE ( 'NONE', #7013, 20.00000000000000000 ) ;
#14715=CARTESIAN_POINT ( 'NONE',  ( 11.69519594420020248, 12.44297266173654748, 19.03762469184452755 ) ) ;
#14716=CARTESIAN_POINT ( 'NONE',  ( 6.587096388939653657, -18.88412458026098406, 24.50000000000000000 ) ) ;
#14717=EDGE_CURVE ( 'NONE', #5725, #28626, #2169, .T. ) ;
#14720=CARTESIAN_POINT ( 'NONE',  ( -17.77309463542032830, -9.210542792609436091, 5.872146474157316831 ) ) ;
#14721=CARTESIAN_POINT ( 'NONE',  ( -6.922783288613180375, 18.78247243576999992, 6.447548852708279377 ) ) ;
#14722=ADVANCED_FACE ( 'NONE', ( #13420 ), #15900, .F. ) ;
#14725=VECTOR ( 'NONE', #3587, 1000.000000000000000 ) ;
#14726=ORIENTED_EDGE ( 'NONE', *, *, #9932, .T. ) ;
#14728=CARTESIAN_POINT ( 'NONE',  ( -5.849168665050582305, 19.12602664087013693, 18.34726407865098707 ) ) ;
#14732=CARTESIAN_POINT ( 'NONE',  ( 19.91398265452213678, -1.852915226174634444, 24.50000000000000000 ) ) ;
#14735=EDGE_CURVE ( 'NONE', #18935, #15666, #4184, .T. ) ;
#14738=DIRECTION ( 'NONE',  ( 1.000000000000000000, 0.000000000000000000, 0.000000000000000000 ) ) ;
#14739=CARTESIAN_POINT ( 'NONE',  ( -8.097046320276927389, -15.01856385377392478, 18.45571264222804686 ) ) ;
#14740=EDGE_CURVE ( 'NONE', #16110, #14537, #28558, .T. ) ;
#14742=ORIENTED_EDGE ( 'NONE', *, *, #6192, .F. ) ;
#14748=CARTESIAN_POINT ( 'NONE',  ( -10.51513057463694523, -17.01270198993485394, 20.34789198813115263 ) ) ;
#14753=AXIS2_PLACEMENT_3D ( 'NONE', #7445, #16949, #17256 ) ;
#14755=CARTESIAN_POINT ( 'NONE',  ( -10.51100353655187369, -17.01524272303503693, 18.34798005863227388 ) ) ;
#14760=CARTESIAN_POINT ( 'NONE',  ( -5.796781398520591821, 16.03935303270742807, 7.652108011868850035 ) ) ;
#14761=CARTESIAN_POINT ( 'NONE',  ( 4.695984468547711899, 19.44110619659980088, 7.454606537396347932 ) ) ;
#14763=VERTEX_POINT ( 'NONE', #30085 ) ;
#14770=EDGE_LOOP ( 'NONE', ( #49, #18684, #25405, #1687 ) ) ;
#14771=EDGE_CURVE ( 'NONE', #25239, #15430, #6534, .T. ) ;
#14773=CARTESIAN_POINT ( 'NONE',  ( 12.97958999564962035, 11.01328844340110713, 19.00652017443069752 ) ) ;
#14774=CARTESIAN_POINT ( 'NONE',  ( -10.80882669148404673, -16.84912922860908679, 5.701226463332907279 ) ) ;
#14776=CARTESIAN_POINT ( 'NONE',  ( 18.52707432543149579, -7.580618987226257488, 18.44527579819791185 ) ) ;
#14778=CARTESIAN_POINT ( 'NONE',  ( 16.70510464924393901, 3.421819763545495441, 18.37415474056476938 ) ) ;
#14781=VERTEX_POINT ( 'NONE', #15730 ) ;
#14783=ORIENTED_EDGE ( 'NONE', *, *, #4804, .F. ) ;
#14789=CARTESIAN_POINT ( 'NONE',  ( -6.855891330591547650, 18.80700764124136626, 18.92976555901915603 ) ) ;
#14790=CARTESIAN_POINT ( 'NONE',  ( -12.71124774491287646, 11.32026698792773978, 19.45164628100866722 ) ) ;
#14791=CARTESIAN_POINT ( 'NONE',  ( -9.692246323650998363, -17.51472466453637367, 19.03762469184452755 ) ) ;
#14796=CARTESIAN_POINT ( 'NONE',  ( 9.496768069075223195, -14.14083042221133724, 5.749228751562096562 ) ) ;
#14804=LINE ( 'NONE', #21828, #18126 ) ;
#14807=CARTESIAN_POINT ( 'NONE',  ( -15.42380629409197645, -7.219239307320219901, 7.453286057244485008 ) ) ;
#14809=ADVANCED_FACE ( 'NONE', ( #6385 ), #25248, .F. ) ;
#14810=DIRECTION ( 'NONE',  ( 1.000000000000000000, 0.000000000000000000, 0.000000000000000000 ) ) ;
#14812=CARTESIAN_POINT ( 'NONE',  ( 5.889883548616666964, 19.11329876149442697, 7.454139397117727661 ) ) ;
#14815=CARTESIAN_POINT ( 'NONE',  ( 9.824744466605370263, -8.513189541288715745, 1.500000000000001332 ) ) ;
#14818=CARTESIAN_POINT ( 'NONE',  ( 9.185733585337914064, -2.352830851074140472, 1.500000000000001332 ) ) ;
#14821=CARTESIAN_POINT ( 'NONE',  ( 16.16412758434837471, -5.502972621964714151, 6.233981582756856987 ) ) ;
#14827=DIRECTION ( 'NONE',  ( 1.000000000000000000, 0.000000000000000000, 0.000000000000000000 ) ) ;
#14829=DIRECTION ( 'NONE',  ( 1.000000000000000000, 0.000000000000000000, 0.000000000000000000 ) ) ;
#14832=CARTESIAN_POINT ( 'NONE',  ( 0.000000000000000000, 0.000000000000000000, 21.50000000000000000 ) ) ;
#14833=CARTESIAN_POINT ( 'NONE',  ( 9.007065134480612301, -14.44288896217592111, 19.45164628100866722 ) ) ;
#14835=EDGE_LOOP ( 'NONE', ( #8952, #3237 ) ) ;
#14843=CARTESIAN_POINT ( 'NONE',  ( -15.17592917621934845, 13.02713289664471397, 18.37250658438899009 ) ) ;
#14845=AXIS2_PLACEMENT_3D ( 'NONE', #4775, #12435, #21463 ) ;
#14847=VECTOR ( 'NONE', #6216, 1000.000000000000000 ) ;
#14850=EDGE_CURVE ( 'NONE', #11240, #9760, #22581, .T. ) ;
#14851=CARTESIAN_POINT ( 'NONE',  ( 19.65528207207770350, 3.699272045506078577, 5.779535427900762024 ) ) ;
#14858=ORIENTED_EDGE ( 'NONE', *, *, #18875, .F. ) ;
#14859=FACE_OUTER_BOUND ( 'NONE', #25975, .T. ) ;
#14861=ORIENTED_EDGE ( 'NONE', *, *, #30346, .F. ) ;
#14873=CYLINDRICAL_SURFACE ( 'NONE', #30033, 9.482273699623480212 ) ;
#14874=CARTESIAN_POINT ( 'NONE',  ( 0.9949940796826640677, -19.99317329078836991, 5.872146474157316831 ) ) ;
#14879=DIRECTION ( 'NONE',  ( 1.000000000000000000, 0.000000000000000000, 0.000000000000000000 ) ) ;
#14880=CARTESIAN_POINT ( 'NONE',  ( -6.934698339095104025, 18.77804097180239395, 6.782048567692550378 ) ) ;
#14881=CARTESIAN_POINT ( 'NONE',  ( 10.64246886845954698, -13.35396698543974203, 6.995624166085161910 ) ) ;
#14886=ORIENTED_EDGE ( 'NONE', *, *, #11905, .F. ) ;
#14891=EDGE_CURVE ( 'NONE', #315, #14448, #21329, .T. ) ;
#14893=ORIENTED_EDGE ( 'NONE', *, *, #5099, .F. ) ;
#14900=LINE ( 'NONE', #7894, #16770 ) ;
#14901=CARTESIAN_POINT ( 'NONE',  ( 0.000000000000000000, 0.000000000000000000, 1.500000000000001332 ) ) ;
#14906=EDGE_LOOP ( 'NONE', ( #7828, #17695, #19335, #15929 ) ) ;
#14907=LINE ( 'NONE', #13041, #14337 ) ;
#14908=EDGE_CURVE ( 'NONE', #10764, #28271, #9084, .T. ) ;
#14911=CYLINDRICAL_SURFACE ( 'NONE', #9338, 0.7500000000000006661 ) ;
#14912=CARTESIAN_POINT ( 'NONE',  ( -19.84344116185556217, 2.497567387674351824, 20.34789198813115263 ) ) ;
#14915=CARTESIAN_POINT ( 'NONE',  ( -14.44122519041009234, -13.83658248990211348, 1.500000000000001332 ) ) ;
#14918=DIRECTION ( 'NONE',  ( -0.000000000000000000, -0.000000000000000000, 1.000000000000000000 ) ) ;
#14921=ORIENTED_EDGE ( 'NONE', *, *, #22526, .F. ) ;
#14926=CARTESIAN_POINT ( 'NONE',  ( -5.524309650260710747, 7.706848733601013635, 13.00000000000000178 ) ) ;
#14927=ORIENTED_EDGE ( 'NONE', *, *, #9078, .F. ) ;
#14928=ORIENTED_EDGE ( 'NONE', *, *, #28663, .F. ) ;
#14931=EDGE_CURVE ( 'NONE', #27751, #1760, #271, .T. ) ;
#14933=VECTOR ( 'NONE', #13527, 1000.000000000000000 ) ;
#14934=CARTESIAN_POINT ( 'NONE',  ( 12.94832566568965504, 11.05145698499349649, 18.90679857307105749 ) ) ;
#14935=CARTESIAN_POINT ( 'NONE',  ( -9.351023488831160080, -14.22394595406099782, 6.310736198168394928 ) ) ;
#14938=DIRECTION ( 'NONE',  ( -0.000000000000000000, -0.000000000000000000, 1.000000000000000000 ) ) ;
#14939=CARTESIAN_POINT ( 'NONE',  ( 16.71904594334103322, 3.341332093703275330, 20.33971507717571114 ) ) ;
#14941=ORIENTED_EDGE ( 'NONE', *, *, #19646, .F. ) ;
#14948=CARTESIAN_POINT ( 'NONE',  ( -6.145639756558241018, 15.91995507688107026, 20.13759033520874908 ) ) ;
#14949=CARTESIAN_POINT ( 'NONE',  ( -14.88094288956370370, 13.38957456607570506, 20.05479082170252525 ) ) ;
#14950=EDGE_CURVE ( 'NONE', #26251, #25239, #28824, .T. ) ;
#14954=DIRECTION ( 'NONE',  ( 0.1423148382732746797, -0.9898214418809342385, 0.000000000000000000 ) ) ;
#14956=CARTESIAN_POINT ( 'NONE',  ( 9.801156115998400864, -13.94312737849039685, 5.653912893140659257 ) ) ;
#14958=CARTESIAN_POINT ( 'NONE',  ( 19.85594780280178639, 2.397944088302079724, 6.033082186765058808 ) ) ;
#14961=CARTESIAN_POINT ( 'NONE',  ( 17.92197892105641799, -8.877232523309841028, 19.08232364404838677 ) ) ;
#14963=CARTESIAN_POINT ( 'NONE',  ( 18.71865409427299909, -7.043577866502360507, 19.21940439362676400 ) ) ;
#14964=CARTESIAN_POINT ( 'NONE',  ( 11.67912593705722735, 12.45929511321702776, 6.917457548096559883 ) ) ;
#14967=CARTESIAN_POINT ( 'NONE',  ( 5.545588074468602358, 19.21617731956022368, 5.676722608126683944 ) ) ;
#14968=ORIENTED_EDGE ( 'NONE', *, *, #16829, .F. ) ;
#14969=CARTESIAN_POINT ( 'NONE',  ( -9.978083804712666094, -17.33339668284229873, 18.54958172136247896 ) ) ;
#14971=CARTESIAN_POINT ( 'NONE',  ( 16.80805182381675422, 2.764250834391624334, 5.749228751562096562 ) ) ;
#14975=CARTESIAN_POINT ( 'NONE',  ( 16.18635831298873740, -5.444400941729625742, 6.892848776733236704 ) ) ;
#14987=CARTESIAN_POINT ( 'NONE',  ( 10.44014025173321514, -17.07989312292649586, 19.96783386855779341 ) ) ;
#14988=CARTESIAN_POINT ( 'NONE',  ( 10.36341371996391736, -17.10561997787537081, 19.85261563089511938 ) ) ;
#14991=CARTESIAN_POINT ( 'NONE',  ( -15.56646378676712672, 12.58598989586694827, 20.29915277494337644 ) ) ;
#14992=DIRECTION ( 'NONE',  ( -0.4154150130018972598, -0.9096319953545133341, 0.000000000000000000 ) ) ;
#14993=ORIENTED_EDGE ( 'NONE', *, *, #17202, .F. ) ;
#14996=CARTESIAN_POINT ( 'NONE',  ( 0.000000000000000000, 0.000000000000000000, 21.50000000000000000 ) ) ;
#15000=CARTESIAN_POINT ( 'NONE',  ( 16.87360174012151504, 2.245128340637304376, 6.973843882838226094 ) ) ;
#15002=ORIENTED_EDGE ( 'NONE', *, *, #24020, .T. ) ;
#15008=EDGE_LOOP ( 'NONE', ( #14260, #7991, #27535, #16714 ) ) ;
#15009=CARTESIAN_POINT ( 'NONE',  ( -9.635826629942096488, -17.52571954072710980, 6.523620417364432100 ) ) ;
#15011=ORIENTED_EDGE ( 'NONE', *, *, #3856, .F. ) ;
#15014=CIRCLE ( 'NONE', #2057, 1.000000000000004441 ) ;
#15019=CARTESIAN_POINT ( 'NONE',  ( -11.33743862782229250, -16.47619710613050614, 6.386539667786095720 ) ) ;
#15023=ORIENTED_EDGE ( 'NONE', *, *, #24989, .T. ) ;
#15025=CARTESIAN_POINT ( 'NONE',  ( -9.389232999038368277, -14.19758896559616623, 19.22654678686458141 ) ) ;
#15026=CARTESIAN_POINT ( 'NONE',  ( -17.62838677698389134, -9.483948870226234007, 6.995624166085161910 ) ) ;
#15027=CARTESIAN_POINT ( 'NONE',  ( -6.307863225249116468, 15.86248630188382869, 6.041646659195333058 ) ) ;
#15028=CARTESIAN_POINT ( 'NONE',  ( 10.14446381905445271, -13.71082019663805163, 5.704143890883081269 ) ) ;
#15030=CARTESIAN_POINT ( 'NONE',  ( -19.84404562991029763, 2.492760124447683800, 18.34798005863226678 ) ) ;
#15032=VERTEX_POINT ( 'NONE', #10412 ) ;
#15034=CARTESIAN_POINT ( 'NONE',  ( -5.001173922442007758, 19.36461358832318425, 19.21471108562413832 ) ) ;
#15037=VECTOR ( 'NONE', #18760, 1000.000000000000000 ) ;
#15038=ORIENTED_EDGE ( 'NONE', *, *, #9638, .T. ) ;
#15039=PRODUCT_CONTEXT ( 'NONE', #29700, 'mechanical' ) ;
#15040=B_SPLINE_CURVE_WITH_KNOTS ( 'NONE', 3,
 ( #8538, #15683, #21976, #7787, #13207, #18193, #3842, #6026, #11019, #605, #22696, #19486, #1348, #6332, #15847, #28998, #7635, #16001, #25825, #16608 ),
 .UNSPECIFIED., .F., .F.,
 ( 4, 2, 2, 2, 2, 2, 2, 2, 2, 4 ),
 ( 0.000000000000000000, 0.06249999999999993755, 0.1249999999999998751, 0.1874999999999998057, 0.2187499999999996669, 0.2499999999999994726, 0.3124999999999996114, 0.3749999999999996114, 0.4374999999999996669, 0.4999999999999997224 ),
 .UNSPECIFIED. ) ;
#15041=CARTESIAN_POINT ( 'NONE',  ( 18.17321615974886129, -8.393345561651576858, 18.44501272782439827 ) ) ;
#15044=CARTESIAN_POINT ( 'NONE',  ( 5.372849316406060005, 19.28330981562107027, 18.34969686940295830 ) ) ;
#15049=CARTESIAN_POINT ( 'NONE',  ( 11.61739189738757183, -16.28020533589259955, 7.454606537396342603 ) ) ;
#15050=CARTESIAN_POINT ( 'NONE',  ( 0.000000000000000000, 0.000000000000000000, 1.500000000000001332 ) ) ;
#15051=CARTESIAN_POINT ( 'NONE',  ( 3.668292057956000551, -8.743977807160085547, 21.50000000000000000 ) ) ;
#15052=CARTESIAN_POINT ( 'NONE',  ( -19.72672318758257148, 3.296256974645891180, 19.96302680909625238 ) ) ;
#15056=CARTESIAN_POINT ( 'NONE',  ( 16.19468640091380962, -5.422205736210276683, 6.783738457429056901 ) ) ;
#15064=ORIENTED_EDGE ( 'NONE', *, *, #24863, .T. ) ;
#15065=CARTESIAN_POINT ( 'NONE',  ( 11.64054540341803978, 16.26338533980433709, 1.500000000000001332 ) ) ;
#15066=CARTESIAN_POINT ( 'NONE',  ( 5.035381156335487773, 19.35612728853643105, 5.679672709359370408 ) ) ;
#15068=VERTEX_POINT ( 'NONE', #24585 ) ;
#15071=CARTESIAN_POINT ( 'NONE',  ( -2.703030265324078307, -12.75514121382991384, 1.500000000000001332 ) ) ;
#15072=DIRECTION ( 'NONE',  ( 1.000000000000000000, 0.000000000000000000, 0.000000000000000000 ) ) ;
#15075=CARTESIAN_POINT ( 'NONE',  ( 15.36220013476732404, 12.83425670785759110, 18.63641924841378028 ) ) ;
#15077=VECTOR ( 'NONE', #5376, 1000.000000000000000 ) ;
#15082=FACE_OUTER_BOUND ( 'NONE', #14906, .T. ) ;
#15083=EDGE_CURVE ( 'NONE', #9540, #30466, #12750, .T. ) ;
#15086=CARTESIAN_POINT ( 'NONE',  ( -16.89625272878630469, 2.150609578401780020, 18.47056384035244037 ) ) ;
#15089=FACE_OUTER_BOUND ( 'NONE', #13190, .T. ) ;
#15092=B_SPLINE_SURFACE_WITH_KNOTS ( 'NONE', 3, 1, ( 
 ( #7468, #4965 ),
 ( #26643, #26172 ),
 ( #28980, #14474 ),
 ( #7615, #14778 ),
 ( #23976, #24296 ),
 ( #11832, #14631 ),
 ( #12464, #2623 ),
 ( #21951, #10102 ),
 ( #5119, #19311 ),
 ( #12143, #6996 ),
 ( #30847, #14310 ),
 ( #26025, #16508 ),
 ( #24130, #21644 ),
 ( #14157, #126 ),
 ( #4654, #279 ),
 ( #2782, #23661 ),
 ( #9798, #21332 ),
 ( #9492, #19008 ),
 ( #12296, #28523 ),
 ( #7154, #16665 ),
 ( #4798, #23826 ),
 ( #2475, #12610 ),
 ( #13227, #3713 ),
 ( #22260, #7936 ),
 ( #27258, #22714 ),
 ( #17591, #22566 ),
 ( #8231, #900 ),
 ( #3396, #1368 ),
 ( #6041, #14939 ),
 ( #24596, #3235 ),
 ( #22419, #19613 ) ),
 .UNSPECIFIED., .F., .F., .F.,
 ( 4, 3, 3, 3, 3, 3, 3, 3, 3, 3, 4 ),
 ( 2, 2 ),
 ( 0.4999999998345686647, 0.5360336730431939367, 0.5907651151589012883, 0.6456034593241830599, 0.6998270958050434309, 0.7529536536315937223, 0.8052385063053260073, 0.8575343587103997356, 0.9106564858195042023, 0.9648414833209685293, 1.000000006602610236 ),
 ( 0.000000000000000000, 1.000000000000000000 ),
 .UNSPECIFIED. ) ;
#15093=CARTESIAN_POINT ( 'NONE',  ( 16.58777033243661592, 4.040313317649105507, 7.196036389296800451 ) ) ;
#15099=DIRECTION ( 'NONE',  ( -0.000000000000000000, -0.000000000000000000, -1.000000000000000000 ) ) ;
#15104=CARTESIAN_POINT ( 'NONE',  ( 11.05488513857797450, -16.68841100269527544, 5.653912893140659257 ) ) ;
#15106=DIRECTION ( 'NONE',  ( 1.000000000000000000, 0.000000000000000000, 0.000000000000000000 ) ) ;
#15113=FACE_OUTER_BOUND ( 'NONE', #11636, .T. ) ;
#15121=CARTESIAN_POINT ( 'NONE',  ( 16.87408724266514426, 2.240810012149825781, 6.974106381145714018 ) ) ;
#15122=ORIENTED_EDGE ( 'NONE', *, *, #6690, .T. ) ;
#15125=EDGE_CURVE ( 'NONE', #20277, #29673, #1207, .T. ) ;
#15131=ORIENTED_EDGE ( 'NONE', *, *, #25619, .F. ) ;
#15132=FACE_OUTER_BOUND ( 'NONE', #20615, .T. ) ;
#15139=ORIENTED_EDGE ( 'NONE', *, *, #28881, .F. ) ;
#15141=CARTESIAN_POINT ( 'NONE',  ( -15.90168156411150058, 12.15925017959999899, 18.82680253904184298 ) ) ;
#15146=CYLINDRICAL_SURFACE ( 'NONE', #13727, 9.482273699623480212 ) ;
#15147=CARTESIAN_POINT ( 'NONE',  ( -14.94050307174418712, 13.29624634855318988, 18.54479204710283824 ) ) ;
#15151=ADVANCED_FACE ( 'NONE', ( #3700 ), #6188, .T. ) ;
#15156=DIRECTION ( 'NONE',  ( -0.8412535328311884220, -0.5406408174555862312, 0.000000000000000000 ) ) ;
#15160=DIRECTION ( 'NONE',  ( -1.000000000000000000, 0.000000000000000000, 0.000000000000000000 ) ) ;
#15163=CIRCLE ( 'NONE', #25649, 20.00000000000000000 ) ;
#15164=CARTESIAN_POINT ( 'NONE',  ( -5.971396161871752817, 19.08775596758251680, 20.34789198813115263 ) ) ;
#15168=LINE ( 'NONE', #5828, #19346 ) ;
#15172=VERTEX_POINT ( 'NONE', #27709 ) ;
#15173=CARTESIAN_POINT ( 'NONE',  ( -11.37242378808260845, -16.47377160145866171, 19.45164628100866722 ) ) ;
#15175=CARTESIAN_POINT ( 'NONE',  ( -5.296822449995555182, 16.19439135686734588, 5.676815824193228721 ) ) ;
#15176=CARTESIAN_POINT ( 'NONE',  ( 11.63559590357233198, -16.28893981701509119, 7.441806358946449151 ) ) ;
#15187=CARTESIAN_POINT ( 'NONE',  ( 3.540451764263689682, 16.69076635161362887, 7.545655578832110244 ) ) ;
#15197=ORIENTED_EDGE ( 'NONE', *, *, #28127, .F. ) ;
#15198=CARTESIAN_POINT ( 'NONE',  ( 9.749114229549594057, -0.1262659238204522361, 21.50000000000000000 ) ) ;
#15200=CARTESIAN_POINT ( 'NONE',  ( 12.99618331672382610, 10.99290767930309443, 19.08155846658118904 ) ) ;
#15201=CARTESIAN_POINT ( 'NONE',  ( 16.14824862691416740, -5.544579173763282576, 7.158811349119585721 ) ) ;
#15203=DIRECTION ( 'NONE',  ( 1.000000000000000000, 0.000000000000000000, 0.000000000000000000 ) ) ;
#15205=DIRECTION ( 'NONE',  ( 1.000000000000000000, 0.000000000000000000, 0.000000000000000000 ) ) ;
#15209=CARTESIAN_POINT ( 'NONE',  ( 6.437683520590175235, -6.962021646281549181, 13.00000000000000178 ) ) ;
#15210=EDGE_LOOP ( 'NONE', ( #13073, #9978, #27432, #9680 ) ) ;
#15211=VERTEX_POINT ( 'NONE', #27247 ) ;
#15220=VERTEX_POINT ( 'NONE', #6340 ) ;
#15223=CARTESIAN_POINT ( 'NONE',  ( 17.90987090234841261, -8.901490003858826938, 6.518927109361837502 ) ) ;
#15233=DIRECTION ( 'NONE',  ( 0.6548607339452782172, -0.7557495743542642641, 0.000000000000000000 ) ) ;
#15235=CARTESIAN_POINT ( 'NONE',  ( 19.73572331631237375, 3.349230485916621092, 5.661398277488801867 ) ) ;
#15237=CARTESIAN_POINT ( 'NONE',  ( -10.24254388992509135, -17.19919274694469991, 20.29915277494337644 ) ) ;
#15240=DIRECTION ( 'NONE',  ( 0.000000000000000000, 0.000000000000000000, 1.000000000000000000 ) ) ;
#15241=CARTESIAN_POINT ( 'NONE',  ( -4.163336342344337027E-14, 1.387778780781445676E-14, 24.50000000000000000 ) ) ;
#15243=CARTESIAN_POINT ( 'NONE',  ( 9.263624429760993095, -14.28705663139043480, 5.940635272151477686 ) ) ;
#15246=EDGE_CURVE ( 'NONE', #3146, #6567, #26197, .T. ) ;
#15247=DIRECTION ( 'NONE',  ( 0.000000000000000000, 0.000000000000000000, -1.000000000000000000 ) ) ;
#15248=ORIENTED_EDGE ( 'NONE', *, *, #14931, .F. ) ;
#15251=EDGE_CURVE ( 'NONE', #4887, #27397, #27322, .T. ) ;
#15252=DIRECTION ( 'NONE',  ( -0.000000000000000000, -0.000000000000000000, 1.000000000000000000 ) ) ;
#15254=CARTESIAN_POINT ( 'NONE',  ( -5.651831417317677797, 19.20339396603468884, 7.595116371587256054 ) ) ;
#15257=AXIS2_PLACEMENT_3D ( 'NONE', #30187, #13670, #16454 ) ;
#15263=CARTESIAN_POINT ( 'NONE',  ( -10.08096377525215104, -17.27393813307046599, 20.22386025856688718 ) ) ;
#15266=CARTESIAN_POINT ( 'NONE',  ( 19.85280965686022014, 2.565335765644449761, 7.429667576816606278 ) ) ;
#15267=ORIENTED_EDGE ( 'NONE', *, *, #4804, .T. ) ;
#15270=ORIENTED_EDGE ( 'NONE', *, *, #29419, .T. ) ;
#15274=CARTESIAN_POINT ( 'NONE',  ( 9.169883732660084164, -9.268939115642975679, 24.50000000000000000 ) ) ;
#15276=EDGE_CURVE ( 'NONE', #29972, #13769, #24095, .T. ) ;
#15278=EDGE_CURVE ( 'NONE', #12217, #2701, #3043, .T. ) ;
#15291=CARTESIAN_POINT ( 'NONE',  ( -15.84987138805250773, 12.22653209092615612, 19.97651184436794125 ) ) ;
#15293=CARTESIAN_POINT ( 'NONE',  ( 0.000000000000000000, 0.000000000000000000, 1.500000000000001332 ) ) ;
#15295=AXIS2_PLACEMENT_3D ( 'NONE', #8206, #7909, #19911 ) ;
#15299=EDGE_CURVE ( 'NONE', #7775, #5590, #9653, .T. ) ;
#15302=CYLINDRICAL_SURFACE ( 'NONE', #6166, 9.482273699623480212 ) ;
#15305=CARTESIAN_POINT ( 'NONE',  ( 16.76361099852355352, 3.068725842366666345, 5.651492010659115550 ) ) ;
#15306=ORIENTED_EDGE ( 'NONE', *, *, #5383, .F. ) ;
#15310=AXIS2_PLACEMENT_3D ( 'NONE', #15530, #20665, #30188 ) ;
#15312=DIRECTION ( 'NONE',  ( -0.000000000000000000, -0.000000000000000000, 1.000000000000000000 ) ) ;
#15316=DIRECTION ( 'NONE',  ( 1.000000000000000000, 0.000000000000000000, 0.000000000000000000 ) ) ;
#15317=CIRCLE ( 'NONE', #3900, 9.482273699623480212 ) ;
#15318=CARTESIAN_POINT ( 'NONE',  ( -19.94274101607340910, 1.513210029880959651, 19.61564845152806313 ) ) ;
#15326=CARTESIAN_POINT ( 'NONE',  ( -11.33851205691660624, -16.47545820588255339, 6.913388067999417963 ) ) ;
#15327=DIRECTION ( 'NONE',  ( -0.000000000000000000, -0.000000000000000000, 1.000000000000000000 ) ) ;
#15328=DIRECTION ( 'NONE',  ( 0.000000000000000000, 0.000000000000000000, -1.000000000000000000 ) ) ;
#15329=AXIS2_PLACEMENT_3D ( 'NONE', #22067, #10070, #5696 ) ;
#15330=ORIENTED_EDGE ( 'NONE', *, *, #28842, .T. ) ;
#15332=AXIS2_PLACEMENT_3D ( 'NONE', #19033, #4680, #12167 ) ;
#15333=ADVANCED_FACE ( 'NONE', ( #25492 ), #21237, .F. ) ;
#15334=VECTOR ( 'NONE', #11579, 1000.000000000000000 ) ;
#15335=CARTESIAN_POINT ( 'NONE',  ( -10.90225941753887362, -16.78887681002774812, 20.25336174263950184 ) ) ;
#15338=CARTESIAN_POINT ( 'NONE',  ( 10.50949999207124641, -13.45141484214875227, 7.280727868105637768 ) ) ;
#15341=CIRCLE ( 'NONE', #1901, 0.7500000000000006661 ) ;
#15347=CYLINDRICAL_SURFACE ( 'NONE', #14415, 0.7500000000000006661 ) ;
#15348=CARTESIAN_POINT ( 'NONE',  ( -0.2028048457436513186, -17.02068360090467536, 6.385774490351131760 ) ) ;
#15351=VECTOR ( 'NONE', #18851, 1000.000000000000000 ) ;
#15353=LINE ( 'NONE', #24883, #30222 ) ;
#15355=CIRCLE ( 'NONE', #14354, 1.000000000000007772 ) ;
#15356=VECTOR ( 'NONE', #11976, 1000.000000000000000 ) ;
#15360=LINE ( 'NONE', #17411, #19332 ) ;
#15366=CARTESIAN_POINT ( 'NONE',  ( 16.19239463133262191, -5.428304825921630439, 6.521906765011495466 ) ) ;
#15370=DIRECTION ( 'NONE',  ( 0.000000000000000000, 0.000000000000000000, 1.000000000000000000 ) ) ;
#15372=CARTESIAN_POINT ( 'NONE',  ( 16.91972452348793610, -3.442972353390052920, -0.6213203435596476032 ) ) ;
#15379=EDGE_LOOP ( 'NONE', ( #17152, #5200 ) ) ;
#15382=CYLINDRICAL_SURFACE ( 'NONE', #3501, 9.482273699623480212 ) ;
#15384=CARTESIAN_POINT ( 'NONE',  ( 5.130938270761610021, -7.974144905643803405, 1.500000000000001332 ) ) ;
#15387=DIRECTION ( 'NONE',  ( -0.6548607339452852116, 0.7557495743542581579, 0.000000000000000000 ) ) ;
#15390=VERTEX_POINT ( 'NONE', #11913 ) ;
#15391=CARTESIAN_POINT ( 'NONE',  ( -16.93532286002824705, 1.879651667671731641, 7.632642797338977658 ) ) ;
#15392=CARTESIAN_POINT ( 'NONE',  ( 18.22972622987024138, -8.227512309863353579, 7.626647697317575414 ) ) ;
#15393=CARTESIAN_POINT ( 'NONE',  ( -10.58794734610131805, -16.98849370068515086, 18.34969686940295830 ) ) ;
#15395=ORIENTED_EDGE ( 'NONE', *, *, #13176, .T. ) ;
#15403=CARTESIAN_POINT ( 'NONE',  ( 16.61573067466907716, 3.902325345048613947, 7.366751648393900176 ) ) ;
#15404=CARTESIAN_POINT ( 'NONE',  ( -14.94322542805485377, 13.31996107294430942, 18.55820869691756769 ) ) ;
#15406=CARTESIAN_POINT ( 'NONE',  ( -8.006961111548649868, -15.06991809617584366, 20.13759033520874908 ) ) ;
#15407=CARTESIAN_POINT ( 'NONE',  ( -17.05006382470648418, 0.8465830297331881082, 19.96568007040467663 ) ) ;
#15408=CARTESIAN_POINT ( 'NONE',  ( -17.01654212181476566, 1.203597991882925378, 18.44527579819791185 ) ) ;
#15410=ORIENTED_EDGE ( 'NONE', *, *, #20633, .T. ) ;
#15416=EDGE_LOOP ( 'NONE', ( #19705, #21657, #4826, #26246 ) ) ;
#15420=CARTESIAN_POINT ( 'NONE',  ( -4.997519263521718713, 19.38405562624022593, 6.641371103590088865 ) ) ;
#15424=CARTESIAN_POINT ( 'NONE',  ( 12.37236664230077743, -12.04390635323149716, 24.50000000000000000 ) ) ;
#15426=LINE ( 'NONE', #26998, #14725 ) ;
#15428=FACE_OUTER_BOUND ( 'NONE', #29301, .T. ) ;
#15429=CARTESIAN_POINT ( 'NONE',  ( 16.86202325244927636, 2.345734461008499583, 6.111214848085761986 ) ) ;
#15430=VERTEX_POINT ( 'NONE', #23283 ) ;
#15431=FACE_OUTER_BOUND ( 'NONE', #9997, .T. ) ;
#15435=B_SPLINE_CURVE_WITH_KNOTS ( 'NONE', 3,
 ( #27173, #24664, #12831, #971, #8150, #20458, #1887, #23233, #25452, #27636, #11411, #27944, #13137, #8611, #15614, #6259, #15772, #24977, #29831, #6421 ),
 .UNSPECIFIED., .F., .F.,
 ( 4, 2, 2, 2, 2, 2, 2, 2, 2, 4 ),
 ( 0.000000000000000000, 0.06249999999999958367, 0.1249999999999991673, 0.1874999999999987510, 0.2187499999999988065, 0.2499999999999988898, 0.3124999999999990563, 0.3749999999999991673, 0.4374999999999992784, 0.4999999999999994449 ),
 .UNSPECIFIED. ) ;
#15440=CARTESIAN_POINT ( 'NONE',  ( 3.111445993792399278, 16.79059500618347656, 6.341840715582230281 ) ) ;
#15441=EDGE_CURVE ( 'NONE', #9025, #4691, #1924, .T. ) ;
#15445=CARTESIAN_POINT ( 'NONE',  ( 9.864935476506834888, -13.90063640520463650, 18.34798005862930736 ) ) ;
#15447=CARTESIAN_POINT ( 'NONE',  ( 19.82764810689592849, 2.754998275627143389, 20.25336174263950184 ) ) ;
#15450=CARTESIAN_POINT ( 'NONE',  ( -19.71348387055304485, 3.477795851889710299, 19.56050940960062690 ) ) ;
#15451=CARTESIAN_POINT ( 'NONE',  ( 15.51152286861890239, -7.023094163498096343, 7.359006845440219102 ) ) ;
#15453=CARTESIAN_POINT ( 'NONE',  ( -13.83017030316320728, 10.00185174541443978, 20.06253562465620632 ) ) ;
#15456=DIRECTION ( 'NONE',  ( 1.000000000000000000, 0.000000000000000000, 0.000000000000000000 ) ) ;
#15459=CARTESIAN_POINT ( 'NONE',  ( -5.651831417317678685, 19.20339396603469240, 20.29090034784956131 ) ) ;
#15463=DIRECTION ( 'NONE',  ( 1.000000000000000000, 0.000000000000000000, 0.000000000000000000 ) ) ;
#15468=ORIENTED_EDGE ( 'NONE', *, *, #20992, .F. ) ;
#15473=DIRECTION ( 'NONE',  ( 0.000000000000000000, 0.000000000000000000, -1.000000000000000000 ) ) ;
#15475=CARTESIAN_POINT ( 'NONE',  ( -19.93487782419341769, 1.613472484145540120, 18.84486140012300126 ) ) ;
#15478=EDGE_CURVE ( 'NONE', #23438, #9760, #22112, .T. ) ;
#15480=EDGE_CURVE ( 'NONE', #14242, #22916, #20625, .T. ) ;
#15486=DIRECTION ( 'NONE',  ( 1.000000000000000000, 0.000000000000000000, 0.000000000000000000 ) ) ;
#15489=CARTESIAN_POINT ( 'NONE',  ( -16.81926493917405807, 2.618766740933698323, 6.910395520694541105 ) ) ;
#15490=VERTEX_POINT ( 'NONE', #19636 ) ;
#15492=CARTESIAN_POINT ( 'NONE',  ( -9.400432693290859731, -14.18986588558385264, 19.33715507985239412 ) ) ;
#15493=CARTESIAN_POINT ( 'NONE',  ( -17.70591931088122806, -9.338465149306657054, 7.280727868105637768 ) ) ;
#15494=ADVANCED_FACE ( 'NONE', ( #28587 ), #17308, .T. ) ;
#15495=CARTESIAN_POINT ( 'NONE',  ( -6.393592071792283171, 18.96945647184856654, 7.559636331181775581 ) ) ;
#15498=CIRCLE ( 'NONE', #6042, 0.7499999999999997780 ) ;
#15501=VERTEX_POINT ( 'NONE', #10604 ) ;
#15504=CARTESIAN_POINT ( 'NONE',  ( -13.35701160122519404, 10.58771215013900502, 5.651989602109218858 ) ) ;
#15510=CARTESIAN_POINT ( 'NONE',  ( -9.085694127122231123, -14.40282604532832167, 7.429667576816606278 ) ) ;
#15511=ADVANCED_FACE ( 'NONE', ( #26669 ), #20115, .F. ) ;
#15513=AXIS2_PLACEMENT_3D ( 'NONE', #19535, #19680, #2693 ) ;
#15515=DIRECTION ( 'NONE',  ( 0.000000000000000000, 0.000000000000000000, -1.000000000000000000 ) ) ;
#15516=CARTESIAN_POINT ( 'NONE',  ( 19.74251403343738076, 3.198927889078825970, 18.34798005863226678 ) ) ;
#15517=EDGE_LOOP ( 'NONE', ( #24552, #22470, #14783, #30422 ) ) ;
#15518=DIRECTION ( 'NONE',  ( -0.000000000000000000, -0.000000000000000000, 1.000000000000000000 ) ) ;
#15522=FACE_OUTER_BOUND ( 'NONE', #13723, .T. ) ;
#15525=DIRECTION ( 'NONE',  ( 0.000000000000000000, 0.000000000000000000, 1.000000000000000000 ) ) ;
#15527=B_SPLINE_CURVE_WITH_KNOTS ( 'NONE', 3,
 ( #29566, #8199, #5858, #10685, #7903, #7743, #3527, #26773, #29715, #22531, #8361, #17877, #26930, #15049, #20654, #27990, #30176, #25346 ),
 .UNSPECIFIED., .F., .F.,
 ( 4, 2, 2, 2, 2, 2, 2, 2, 4 ),
 ( 0.000000000000000000, 0.0003967869494442896193, 0.0007935738988885792386, 0.001190360848332868912, 0.001587147797777158477, 0.001983934747221448042, 0.002380721696665737824, 0.002777508646110027173, 0.003174295595554316955 ),
 .UNSPECIFIED. ) ;
#15530=CARTESIAN_POINT ( 'NONE',  ( 12.72536390617885438, -2.839914339433650348, 1.500000000000001332 ) ) ;
#15533=ORIENTED_EDGE ( 'NONE', *, *, #11907, .T. ) ;
#15537=DIRECTION ( 'NONE',  ( 1.000000000000000000, 0.000000000000000000, 0.000000000000000000 ) ) ;
#15538=ORIENTED_EDGE ( 'NONE', *, *, #9965, .F. ) ;
#15540=DIRECTION ( 'NONE',  ( 0.000000000000000000, 0.000000000000000000, 1.000000000000000000 ) ) ;
#15543=ORIENTED_EDGE ( 'NONE', *, *, #11839, .T. ) ;
#15545=CARTESIAN_POINT ( 'NONE',  ( -6.315055774950723233, 15.86014940731417866, 18.73314399819311760 ) ) ;
#15546=CARTESIAN_POINT ( 'NONE',  ( 9.013259606647444855, -14.43917691232923417, 19.47784884541372818 ) ) ;
#15548=ORIENTED_EDGE ( 'NONE', *, *, #11644, .F. ) ;
#15549=ORIENTED_EDGE ( 'NONE', *, *, #6192, .T. ) ;
#15555=LINE ( 'NONE', #20231, #4882 ) ;
#15559=CARTESIAN_POINT ( 'NONE',  ( -16.81857544482621236, 2.623036418782660473, 19.08155846658118904 ) ) ;
#15562=FACE_OUTER_BOUND ( 'NONE', #5566, .T. ) ;
#15563=CARTESIAN_POINT ( 'NONE',  ( 16.73033351903584887, 3.274018421667482137, 5.652605728828373977 ) ) ;
#15565=CARTESIAN_POINT ( 'NONE',  ( -7.692543755867210287, -15.24678548464671124, 19.58863275299554019 ) ) ;
#15567=LINE ( 'NONE', #8250, #23456 ) ;
#15569=EDGE_LOOP ( 'NONE', ( #12216, #19669, #27989, #19683 ) ) ;
#15574=ORIENTED_EDGE ( 'NONE', *, *, #25043, .T. ) ;
#15579=AXIS2_PLACEMENT_3D ( 'NONE', #25051, #22861, #15537 ) ;
#15580=CARTESIAN_POINT ( 'NONE',  ( -5.048943207435892866, 19.37072948160042074, 6.974106381145714018 ) ) ;
#15585=ORIENTED_EDGE ( 'NONE', *, *, #23501, .T. ) ;
#15587=CARTESIAN_POINT ( 'NONE',  ( 12.25310179107605890, 11.85582831497230671, 5.661398277488801867 ) ) ;
#15588=CARTESIAN_POINT ( 'NONE',  ( 16.87674189766845956, 2.217009531549524848, 6.864725433338323413 ) ) ;
#15590=CARTESIAN_POINT ( 'NONE',  ( 15.04472583903953975, 13.20536594261729491, 5.670038381137163519 ) ) ;
#15592=CARTESIAN_POINT ( 'NONE',  ( 0.000000000000000000, 0.000000000000000000, 1.500000000000001332 ) ) ;
#15593=ORIENTED_EDGE ( 'NONE', *, *, #7287, .T. ) ;
#15602=CARTESIAN_POINT ( 'NONE',  ( 9.054000795813630376, -14.41483084819681260, 19.00652017443069752 ) ) ;
#15606=CARTESIAN_POINT ( 'NONE',  ( 15.63429980755321935, -6.761683097800861297, 5.749228751562096562 ) ) ;
#15607=CARTESIAN_POINT ( 'NONE',  ( -13.83904721019127848, 9.990416291640219271, 5.951255046771932733 ) ) ;
#15608=CARTESIAN_POINT ( 'NONE',  ( 3.111445993792395281, 16.79059500618346945, 19.03762469184452755 ) ) ;
#15612=CARTESIAN_POINT ( 'NONE',  ( 10.29773160334160131, -13.60426929931266038, 5.759928666072751113 ) ) ;
#15613=B_SPLINE_SURFACE_WITH_KNOTS ( 'NONE', 3, 1, ( 
 ( #15890, #17758 ),
 ( #8569, #15719 ),
 ( #6215, #29932 ),
 ( #27591, #18395 ),
 ( #27276, #25237 ),
 ( #5909, #15408 ),
 ( #10738, #3884 ),
 ( #20248, #29774 ),
 ( #8415, #13409 ),
 ( #22893, #1541 ),
 ( #11051, #13555 ),
 ( #23035, #1685 ),
 ( #11201, #18534 ),
 ( #26312, #11975 ),
 ( #28039, #21468 ),
 ( #18679, #6667 ),
 ( #7285, #25699 ),
 ( #21002, #20859 ),
 ( #16183, #28186 ),
 ( #30832, #2287 ),
 ( #109, #4327 ),
 ( #9629, #7137 ),
 ( #6817, #16493 ),
 ( #9478, #23643 ),
 ( #13854, #11658 ),
 ( #23497, #2141 ),
 ( #25859, #21312 ),
 ( #13703, #23355 ),
 ( #4491, #2457 ),
 ( #11809, #14289 ),
 ( #1994, #28359 ) ),
 .UNSPECIFIED., .F., .F., .F.,
 ( 4, 3, 3, 3, 3, 3, 3, 3, 3, 3, 4 ),
 ( 2, 2 ),
 ( 0.4999999998345687757, 0.5360336730431939367, 0.5907651151589012883, 0.6456034593241830599, 0.6998270958050434309, 0.7529536536315937223, 0.8052385063053260073, 0.8575343587103997356, 0.9106564858195042023, 0.9648414833209685293, 1.000000006602610014 ),
 ( 0.000000000000000000, 1.000000000000000000 ),
 .UNSPECIFIED. ) ;
#15614=CARTESIAN_POINT ( 'NONE',  ( 12.88304655974325108, 11.13107787108148550, 6.031926333436654630 ) ) ;
#15617=EDGE_CURVE ( 'NONE', #7784, #28377, #28605, .T. ) ;
#15618=CARTESIAN_POINT ( 'NONE',  ( -0.1262659238204836554, -8.999114229549588728, 1.500000000000001332 ) ) ;
#15622=CIRCLE ( 'NONE', #29077, 0.7499999999999988898 ) ;
#15623=ORIENTED_EDGE ( 'NONE', *, *, #19319, .T. ) ;
#15628=EDGE_LOOP ( 'NONE', ( #2987, #2143, #23505, #4055 ) ) ;
#15629=CARTESIAN_POINT ( 'NONE',  ( -8.072557715923444732, 14.41080185948837311, 1.500000000000000000 ) ) ;
#15631=CARTESIAN_POINT ( 'NONE',  ( -19.84344116185556217, 2.497567387674351824, 20.34789198813115263 ) ) ;
#15633=DIRECTION ( 'NONE',  ( 0.000000000000000000, 0.000000000000000000, 1.000000000000000000 ) ) ;
#15635=DIRECTION ( 'NONE',  ( 0.000000000000000000, 0.000000000000000000, 1.000000000000000000 ) ) ;
#15641=CARTESIAN_POINT ( 'NONE',  ( 1.139261986572422281, -19.98520933375988662, 7.280727868105637768 ) ) ;
#15642=CARTESIAN_POINT ( 'NONE',  ( -0.1262659238204836554, -8.999114229549588728, 1.500000000000001332 ) ) ;
#15644=CARTESIAN_POINT ( 'NONE',  ( -11.32740345151500172, -16.50481001894685917, 19.00652017443069752 ) ) ;
#15645=CARTESIAN_POINT ( 'NONE',  ( -14.73262409220166269, -8.633676228711859579, 6.995624166085161910 ) ) ;
#15647=CARTESIAN_POINT ( 'NONE',  ( -14.71031647956046129, -8.675071222119056458, 19.14333282897057842 ) ) ;
#15650=ORIENTED_EDGE ( 'NONE', *, *, #25197, .F. ) ;
#15651=ORIENTED_EDGE ( 'NONE', *, *, #6937, .T. ) ;
#15655=CARTESIAN_POINT ( 'NONE',  ( -15.28428954155913644, 12.92682542062230944, 5.657991946698900598 ) ) ;
#15660=CARTESIAN_POINT ( 'NONE',  ( -10.89423172471906476, -16.79374140667819759, 5.749228751562096562 ) ) ;
#15662=ORIENTED_EDGE ( 'NONE', *, *, #20999, .T. ) ;
#15666=VERTEX_POINT ( 'NONE', #6072 ) ;
#15668=CYLINDRICAL_SURFACE ( 'NONE', #20340, 9.482273699623480212 ) ;
#15671=CARTESIAN_POINT ( 'NONE',  ( -16.46198811862381817, -1.356593340923033075, 24.50000000000000000 ) ) ;
#15672=VERTEX_POINT ( 'NONE', #30398 ) ;
#15673=CARTESIAN_POINT ( 'NONE',  ( 9.169883732660084164, -9.268939115642975679, 24.50000000000000000 ) ) ;
#15677=DIRECTION ( 'NONE',  ( 0.5406408174555976665, -0.8412535328311810945, -0.000000000000000000 ) ) ;
#15678=CARTESIAN_POINT ( 'NONE',  ( -19.91398265452221850, -1.852915226174651986, 24.50000000000000000 ) ) ;
#15680=AXIS2_PLACEMENT_3D ( 'NONE', #26451, #5081, #14592 ) ;
#15682=CARTESIAN_POINT ( 'NONE',  ( -7.974144905643822945, -5.130938270761581599, 1.500000000000001332 ) ) ;
#15683=CARTESIAN_POINT ( 'NONE',  ( 9.752055262503102284, -13.97602916338938250, 7.652108011868852699 ) ) ;
#15686=VERTEX_POINT ( 'NONE', #13713 ) ;
#15687=ORIENTED_EDGE ( 'NONE', *, *, #19872, .F. ) ;
#15693=VERTEX_POINT ( 'NONE', #22750 ) ;
#15698=ORIENTED_EDGE ( 'NONE', *, *, #21608, .T. ) ;
#15700=CARTESIAN_POINT ( 'NONE',  ( -19.77235582619724141, 3.126546698941333080, 5.862424720655265098 ) ) ;
#15702=CARTESIAN_POINT ( 'NONE',  ( -8.738547258790619665, -14.62818084867463142, 18.36582235739946611 ) ) ;
#15708=EDGE_CURVE ( 'NONE', #4843, #16773, #6208, .T. ) ;
#15714=CARTESIAN_POINT ( 'NONE',  ( 19.57334175050933212, 4.193940174973930013, 6.672349528511551497 ) ) ;
#15717=CARTESIAN_POINT ( 'NONE',  ( -9.983339604393954403, -17.35078046477760694, 20.13759033520874908 ) ) ;
#15719=CARTESIAN_POINT ( 'NONE',  ( -16.97503503882429854, 1.572081968053589351, 18.34838970509067479 ) ) ;
#15723=EDGE_CURVE ( 'NONE', #4543, #23230, #29132, .T. ) ;
#15724=CARTESIAN_POINT ( 'NONE',  ( 11.94785300146925699, -16.06093515404948846, 19.25672174529527325 ) ) ;
#15728=AXIS2_PLACEMENT_3D ( 'NONE', #14901, #5240, #14738 ) ;
#15730=CARTESIAN_POINT ( 'NONE',  ( 11.64054540341803978, 16.26338533980433709, 24.50000000000000000 ) ) ;
#15731=CARTESIAN_POINT ( 'NONE',  ( -5.475907499891255803, 16.13963752243575200, 5.653912893140659257 ) ) ;
#15735=CARTESIAN_POINT ( 'NONE',  ( -12.71180423606275767, 11.31964500333552692, 6.714907520933424578 ) ) ;
#15739=VECTOR ( 'NONE', #29388, 1000.000000000000000 ) ;
#15744=CARTESIAN_POINT ( 'NONE',  ( -13.54809176563293427, 10.35918576916548695, 20.34789198813115618 ) ) ;
#15746=ORIENTED_EDGE ( 'NONE', *, *, #27865, .T. ) ;
#15747=ORIENTED_EDGE ( 'NONE', *, *, #1783, .T. ) ;
#15749=CARTESIAN_POINT ( 'NONE',  ( 3.352743984114611830, 16.73528478182341672, 7.366751648393900176 ) ) ;
#15751=DIRECTION ( 'NONE',  ( 0.000000000000000000, 0.000000000000000000, 1.000000000000000000 ) ) ;
#15754=AXIS2_PLACEMENT_3D ( 'NONE', #22912, #1561, #20569 ) ;
#15756=CARTESIAN_POINT ( 'NONE',  ( 10.34995923732865108, -17.13460031806512873, 18.90679857307105749 ) ) ;
#15758=ORIENTED_EDGE ( 'NONE', *, *, #8843, .F. ) ;
#15759=FACE_OUTER_BOUND ( 'NONE', #20142, .T. ) ;
#15761=CARTESIAN_POINT ( 'NONE',  ( 15.38325456941029579, -7.285321374151288332, 6.641371103590088865 ) ) ;
#15763=CARTESIAN_POINT ( 'NONE',  ( -15.97321056478110179, 12.06495093120146045, 6.892848776733236704 ) ) ;
#15764=CARTESIAN_POINT ( 'NONE',  ( 3.978203543573291867, 16.57681993851655022, 20.34789198813115263 ) ) ;
#15765=ORIENTED_EDGE ( 'NONE', *, *, #19086, .F. ) ;
#15768=LINE ( 'NONE', #28085, #26236 ) ;
#15769=CIRCLE ( 'NONE', #6307, 20.00000000000000000 ) ;
#15770=CARTESIAN_POINT ( 'NONE',  ( 10.67036453487905767, -13.33339184396348287, 6.917457548096560771 ) ) ;
#15771=CARTESIAN_POINT ( 'NONE',  ( 15.45572804192158500, 12.69342571624615168, 18.84056766331480404 ) ) ;
#15772=CARTESIAN_POINT ( 'NONE',  ( 12.69001473637765365, 11.36098604101993637, 5.774779864094941040 ) ) ;
#15773=CARTESIAN_POINT ( 'NONE',  ( 0.000000000000000000, 0.000000000000000000, 1.500000000000001332 ) ) ;
#15775=AXIS2_PLACEMENT_3D ( 'NONE', #2712, #22035, #10187 ) ;
#15779=CIRCLE ( 'NONE', #25752, 9.482273699623480212 ) ;
#15780=DIRECTION ( 'NONE',  ( 0.000000000000000000, 0.000000000000000000, 1.000000000000000000 ) ) ;
#15783=ORIENTED_EDGE ( 'NONE', *, *, #8480, .T. ) ;
#15786=DIRECTION ( 'NONE',  ( 0.000000000000000000, 0.000000000000000000, -1.000000000000000000 ) ) ;
#15787=ORIENTED_EDGE ( 'NONE', *, *, #21146, .F. ) ;
#15790=DIRECTION ( 'NONE',  ( -0.000000000000000000, -0.000000000000000000, 1.000000000000000000 ) ) ;
#15792=VECTOR ( 'NONE', #30143, 1000.000000000000227 ) ;
#15793=LINE ( 'NONE', #17843, #13344 ) ;
#15796=CARTESIAN_POINT ( 'NONE',  ( 1.733314906354231910, -16.98782497260186375, 6.995624166085161910 ) ) ;
#15797=CARTESIAN_POINT ( 'NONE',  ( -16.81857544482355493, 2.623036418797992209, 6.385774490351135313 ) ) ;
#15800=CARTESIAN_POINT ( 'NONE',  ( 6.778663211761466911, -6.630478080506930105, 1.500000000000001332 ) ) ;
#15802=CARTESIAN_POINT ( 'NONE',  ( -4.769904382622641492, 16.34378370247567247, 7.267659094423558841 ) ) ;
#15803=CARTESIAN_POINT ( 'NONE',  ( -18.02600256144196678, -8.705149951716494527, 18.34838970509067479 ) ) ;
#15804=AXIS2_PLACEMENT_3D ( 'NONE', #18056, #4160, #11349 ) ;
#15817=CARTESIAN_POINT ( 'NONE',  ( 3.068634486547840101, 16.80010772488981985, 6.521906765011495466 ) ) ;
#15821=AXIS2_PLACEMENT_3D ( 'NONE', #1748, #15955, #1904 ) ;
#15824=CARTESIAN_POINT ( 'NONE',  ( -8.099370871304801156, -15.01721251058671491, 20.24143955528809258 ) ) ;
#15825=CARTESIAN_POINT ( 'NONE',  ( -10.00000000000004263, 1.387778780781445676E-14, 21.50000000000000000 ) ) ;
#15829=B_SPLINE_CURVE_WITH_KNOTS ( 'NONE', 3,
 ( #7740, #5086, #14739, #16938, #12424, #21919, #26455, #29099, #7900, #3205, #8050, #17242, #17407, #15824, #22843, #1325 ),
 .UNSPECIFIED., .F., .F.,
 ( 4, 2, 2, 2, 2, 2, 2, 4 ),
 ( 0.5000000000000000000, 0.6250000000000015543, 0.6875000000000021094, 0.7187500000000023315, 0.7500000000000025535, 0.8125000000000014433, 0.8750000000000003331, 1.000000000000000000 ),
 .UNSPECIFIED. ) ;
#15833=DIRECTION ( 'NONE',  ( 0.000000000000000000, 0.000000000000000000, 1.000000000000000000 ) ) ;
#15834=CARTESIAN_POINT ( 'NONE',  ( 12.88304655979403712, 11.13107787102070745, 18.72771030977187223 ) ) ;
#15840=CARTESIAN_POINT ( 'NONE',  ( -15.42263072602161422, -7.221902784682912468, 18.54473042795394733 ) ) ;
#15844=EDGE_CURVE ( 'NONE', #15686, #17832, #2471, .T. ) ;
#15847=CARTESIAN_POINT ( 'NONE',  ( 9.184330860425914622, -14.33603326861445382, 6.031926333436654630 ) ) ;
#15848=CARTESIAN_POINT ( 'NONE',  ( -9.395348974764861083, -14.19336984580852956, 19.41069149716887665 ) ) ;
#15855=CARTESIAN_POINT ( 'NONE',  ( 12.24063095261064404, 4.490763173670002217, 1.500000000000001332 ) ) ;
#15865=CARTESIAN_POINT ( 'NONE',  ( -16.87659098782771849, 2.276273425076629664, 5.862424720655265098 ) ) ;
#15869=DIRECTION ( 'NONE',  ( 1.000000000000000000, 0.000000000000000000, 0.000000000000000000 ) ) ;
#15881=LINE ( 'NONE', #18068, #23042 ) ;
#15882=B_SPLINE_SURFACE_WITH_KNOTS ( 'NONE', 3, 1, ( 
 ( #25734, #4672 ),
 ( #143, #23992 ),
 ( #14174, #2178 ),
 ( #13886, #21658 ),
 ( #18573, #2325 ),
 ( #23388, #21351 ),
 ( #28079, #9507 ),
 ( #16681, #11550 ),
 ( #19025, #29470 ),
 ( #29151, #7633 ),
 ( #5135, #16982 ),
 ( #26504, #8104 ),
 ( #22279, #748 ),
 ( #12778, #2797 ),
 ( #3417, #24774 ),
 ( #12481, #28996 ),
 ( #17460, #12942 ),
 ( #17295, #922 ),
 ( #29314, #21973 ),
 ( #24467, #22435 ),
 ( #27129, #14646 ),
 ( #5752, #15243 ),
 ( #26829, #5289 ),
 ( #24148, #26982 ),
 ( #21820, #14796 ),
 ( #5608, #26659 ),
 ( #5453, #7487 ),
 ( #602, #10438 ),
 ( #15104, #14956 ),
 ( #19952, #461 ),
 ( #19483, #24619 ) ),
 .UNSPECIFIED., .F., .F., .F.,
 ( 4, 3, 3, 3, 3, 3, 3, 3, 3, 3, 4 ),
 ( 2, 2 ),
 ( 0.000000000000000000, 0.05425176834609633791, 0.1085332949128352958, 0.1623767749169382768, 0.2157504826133063158, 0.2688657508888171455, 0.3218907763505476360, 0.3749548578363336993, 0.4282048033836242107, 0.4818374082110501444, 0.4999999999131655715 ),
 ( 0.000000000000000000, 1.000000000000000000 ),
 .UNSPECIFIED. ) ;
#15883=CARTESIAN_POINT ( 'NONE',  ( 16.74328840634222715, 3.194145055459935101, 7.652108011868850035 ) ) ;
#15886=VECTOR ( 'NONE', #24836, 1000.000000000000000 ) ;
#15888=CARTESIAN_POINT ( 'NONE',  ( -7.726154291500652249, -15.22816856119838391, 19.69140814234746273 ) ) ;
#15889=DIRECTION ( 'NONE',  ( -0.000000000000000000, -0.000000000000000000, -1.000000000000000000 ) ) ;
#15890=CARTESIAN_POINT ( 'NONE',  ( -19.86132161767506688, 2.497832813224996951, 18.34798005862662507 ) ) ;
#15891=CARTESIAN_POINT ( 'NONE',  ( 0.4269445148198162121, -2.969464325642846347, 24.50000000000000000 ) ) ;
#15895=AXIS2_PLACEMENT_3D ( 'NONE', #725, #17268, #16959 ) ;
#15900=CYLINDRICAL_SURFACE ( 'NONE', #18613, 0.7500000000000006661 ) ;
#15901=ADVANCED_FACE ( 'NONE', ( #2155 ), #12620, .T. ) ;
#15902=CARTESIAN_POINT ( 'NONE',  ( -5.002692087210952820, 19.38273059899790596, 6.755862304746362845 ) ) ;
#15907=DIRECTION ( 'NONE',  ( 1.000000000000000000, 0.000000000000000000, 0.000000000000000000 ) ) ;
#15912=VERTEX_POINT ( 'NONE', #17439 ) ;
#15916=DIRECTION ( 'NONE',  ( 1.000000000000000000, 0.000000000000000000, 0.000000000000000000 ) ) ;
#15917=EDGE_CURVE ( 'NONE', #28288, #3771, #5582, .T. ) ;
#15918=EDGE_CURVE ( 'NONE', #17265, #10035, #22414, .T. ) ;
#15922=CARTESIAN_POINT ( 'NONE',  ( 4.982076346116051546, 19.38816267120398606, 7.603368798681074736 ) ) ;
#15927=CARTESIAN_POINT ( 'NONE',  ( 9.331524088667743300, -14.24511854140749811, 18.55820869691756769 ) ) ;
#15928=DIRECTION ( 'NONE',  ( 1.000000000000000000, 0.000000000000000000, 0.000000000000000000 ) ) ;
#15929=ORIENTED_EDGE ( 'NONE', *, *, #10320, .T. ) ;
#15931=CARTESIAN_POINT ( 'NONE',  ( 15.67520293387196517, -6.672517015027196408, 7.595116371587256054 ) ) ;
#15932=CARTESIAN_POINT ( 'NONE',  ( -13.59008529392185238, 10.30512752726515302, 20.29915277494337644 ) ) ;
#15933=CARTESIAN_POINT ( 'NONE',  ( 3.160432912108479098, 16.77963207014077796, 19.79423548914561692 ) ) ;
#15938=CARTESIAN_POINT ( 'NONE',  ( -4.718303904200451093, 16.35736724179925972, 19.87181966307587544 ) ) ;
#15942=CARTESIAN_POINT ( 'NONE',  ( 6.587096388939653657, -18.88412458026098406, 24.50000000000000000 ) ) ;
#15946=CARTESIAN_POINT ( 'NONE',  ( 1.164358918501127604, -19.96629823696783035, 6.037995405461183296 ) ) ;
#15948=CYLINDRICAL_SURFACE ( 'NONE', #2502, 9.482273699623480212 ) ;
#15952=DIRECTION ( 'NONE',  ( 0.000000000000000000, 0.000000000000000000, -1.000000000000000000 ) ) ;
#15953=CARTESIAN_POINT ( 'NONE',  ( -19.86062922652984852, 2.360743482685567773, 18.34869673959212122 ) ) ;
#15955=DIRECTION ( 'NONE',  ( 0.000000000000000000, 0.000000000000000000, -1.000000000000000000 ) ) ;
#15964=LINE ( 'NONE', #25779, #29237 ) ;
#15966=CYLINDRICAL_SURFACE ( 'NONE', #588, 0.7500000000000006661 ) ;
#15967=CARTESIAN_POINT ( 'NONE',  ( 11.39002951368468253, -16.46174851469273293, 7.603368798681074736 ) ) ;
#15971=CYLINDRICAL_SURFACE ( 'NONE', #2448, 0.7500000000000015543 ) ;
#15974=CARTESIAN_POINT ( 'NONE',  ( -12.54846374865995706, -9.550116103605043705, -0.6213203435596476032 ) ) ;
#15976=AXIS2_PLACEMENT_3D ( 'NONE', #21333, #14158, #19010 ) ;
#15977=CARTESIAN_POINT ( 'NONE',  ( -13.71169828473024488, 10.15410312375059476, 7.545655578832112909 ) ) ;
#15980=ORIENTED_EDGE ( 'NONE', *, *, #22155, .T. ) ;
#15988=DIRECTION ( 'NONE',  ( -0.000000000000000000, -0.000000000000000000, 1.000000000000000000 ) ) ;
#15993=AXIS2_PLACEMENT_3D ( 'NONE', #825, #17205, #21888 ) ;
#15995=AXIS2_PLACEMENT_3D ( 'NONE', #30076, #1391, #3729 ) ;
#15996=LINE ( 'NONE', #6632, #7353 ) ;
#16001=CARTESIAN_POINT ( 'NONE',  ( 9.644751206715360681, -14.04611738690515566, 5.676815824193228721 ) ) ;
#16004=EDGE_LOOP ( 'NONE', ( #7490, #23443, #2177, #9382 ) ) ;
#16005=CARTESIAN_POINT ( 'NONE',  ( -4.340342926365016396, -8.430595340551244377, 13.00000000000000178 ) ) ;
#16007=DIRECTION ( 'NONE',  ( 1.000000000000000000, 0.000000000000000000, 0.000000000000000000 ) ) ;
#16014=CARTESIAN_POINT ( 'NONE',  ( -10.51100883930070040, -17.01524884273342764, 18.34798005863226678 ) ) ;
#16016=CARTESIAN_POINT ( 'NONE',  ( -10.52280129341197323, -17.02885805942690567, 18.34798005862930381 ) ) ;
#16017=EDGE_CURVE ( 'NONE', #13348, #12864, #4934, .T. ) ;
#16018=DIRECTION ( 'NONE',  ( 0.000000000000000000, 0.000000000000000000, -1.000000000000000000 ) ) ;
#16019=VERTEX_POINT ( 'NONE', #6194 ) ;
#16021=ORIENTED_EDGE ( 'NONE', *, *, #11824, .T. ) ;
#16024=CARTESIAN_POINT ( 'NONE',  ( -15.34307810681595718, 12.82926163924266483, 7.652108011868850035 ) ) ;
#16028=CIRCLE ( 'NONE', #2585, 20.00000000000000000 ) ;
#16030=CARTESIAN_POINT ( 'NONE',  ( 0.3346962451677066297, -17.03061174119336840, 7.557577766377196582 ) ) ;
#16032=DIRECTION ( 'NONE',  ( -0.000000000000000000, -0.000000000000000000, 1.000000000000000000 ) ) ;
#16033=EDGE_CURVE ( 'NONE', #23120, #21154, #8725, .T. ) ;
#16034=DIRECTION ( 'NONE',  ( 0.000000000000000000, 0.000000000000000000, -1.000000000000000000 ) ) ;
#16039=CARTESIAN_POINT ( 'NONE',  ( 11.11866356627124297, -16.64591798801204447, 18.34798005862662507 ) ) ;
#16044=DIRECTION ( 'NONE',  ( 0.000000000000000000, 0.000000000000000000, 1.000000000000000000 ) ) ;
#16045=CARTESIAN_POINT ( 'NONE',  ( -4.568010850242218091, 16.39675899511905399, 6.641371103590088865 ) ) ;
#16048=EDGE_CURVE ( 'NONE', #27304, #2787, #3239, .T. ) ;
#16049=ORIENTED_EDGE ( 'NONE', *, *, #21517, .T. ) ;
#16050=EDGE_CURVE ( 'NONE', #15430, #25523, #2232, .T. ) ;
#16061=ORIENTED_EDGE ( 'NONE', *, *, #23639, .T. ) ;
#16062=ORIENTED_EDGE ( 'NONE', *, *, #12650, .F. ) ;
#16065=DIRECTION ( 'NONE',  ( 0.000000000000000000, 0.000000000000000000, -1.000000000000000000 ) ) ;
#16070=CARTESIAN_POINT ( 'NONE',  ( 11.08678458728283545, -16.66722406908985477, 18.34777357837152323 ) ) ;
#16073=VECTOR ( 'NONE', #23191, 1000.000000000000000 ) ;
#16074=CARTESIAN_POINT ( 'NONE',  ( -16.92011235424303450, 1.986018190673852546, 20.29090034784956131 ) ) ;
#16075=CARTESIAN_POINT ( 'NONE',  ( 17.92217092160593950, -8.916983838001998564, 6.641371103590088865 ) ) ;
#16076=CARTESIAN_POINT ( 'NONE',  ( -15.89252301733158568, 12.17122019226246721, 7.196036389296800451 ) ) ;
#16077=CARTESIAN_POINT ( 'NONE',  ( 5.225607896785843920, 19.32380464960333555, 18.34838970509067479 ) ) ;
#16078=ORIENTED_EDGE ( 'NONE', *, *, #20090, .T. ) ;
#16081=CARTESIAN_POINT ( 'NONE',  ( 10.66613195287249560, -13.33645323721333220, 6.392658652357120275 ) ) ;
#16083=CARTESIAN_POINT ( 'NONE',  ( -4.619434794156388691, 16.38343285047924169, 19.66989035740801839 ) ) ;
#16085=CARTESIAN_POINT ( 'NONE',  ( 11.75084321055180858, 12.38658771205033560, 6.147510495896842286 ) ) ;
#16090=ADVANCED_FACE ( 'NONE', ( #11958 ), #22330, .T. ) ;
#16091=CARTESIAN_POINT ( 'NONE',  ( -19.96188467872886463, 1.492656647078446364, 6.782048567692550378 ) ) ;
#16093=DIRECTION ( 'NONE',  ( 1.000000000000000000, 0.000000000000000000, 0.000000000000000000 ) ) ;
#16094=EDGE_LOOP ( 'NONE', ( #29424, #19361 ) ) ;
#16096=CIRCLE ( 'NONE', #17586, 0.7499999999999988898 ) ;
#16099=CARTESIAN_POINT ( 'NONE',  ( 16.06085112851925345, -5.768724642094694488, 5.872146474157316831 ) ) ;
#16103=DIRECTION ( 'NONE',  ( -0.000000000000000000, -0.000000000000000000, 1.000000000000000000 ) ) ;
#16105=CARTESIAN_POINT ( 'NONE',  ( 3.912171961291952105, 8.637616862297853970, 21.50000000000000000 ) ) ;
#16109=CARTESIAN_POINT ( 'NONE',  ( -16.87834697512587212, 2.265528671477828215, 7.453286057244489449 ) ) ;
#16110=VERTEX_POINT ( 'NONE', #8046 ) ;
#16111=CARTESIAN_POINT ( 'NONE',  ( 5.738360882149947884, 7.548823014270664267, 21.50000000000000000 ) ) ;
#16114=FACE_OUTER_BOUND ( 'NONE', #8, .T. ) ;
#16116=CARTESIAN_POINT ( 'NONE',  ( -17.99270058295304509, -8.773758909272052264, 18.35718225375110180 ) ) ;
#16123=DIRECTION ( 'NONE',  ( 1.000000000000000000, 0.000000000000000000, 0.000000000000000000 ) ) ;
#16124=DIRECTION ( 'NONE',  ( 1.000000000000000000, 0.000000000000000000, 0.000000000000000000 ) ) ;
#16128=CARTESIAN_POINT ( 'NONE',  ( -4.163336342344337027E-14, 1.387778780781445676E-14, 24.50000000000000000 ) ) ;
#16131=FACE_OUTER_BOUND ( 'NONE', #936, .T. ) ;
#16133=B_SPLINE_SURFACE_WITH_KNOTS ( 'NONE', 3, 1, ( 
 ( #1432, #8290 ),
 ( #11233, #20729 ),
 ( #30260, #8907 ),
 ( #29963, #27932 ),
 ( #15447, #4206 ),
 ( #27320, #3763 ),
 ( #13730, #30109 ),
 ( #13282, #11088 ),
 ( #3926, #29653 ),
 ( #22620, #22776 ),
 ( #10947, #1270 ),
 ( #13446, #10778 ),
 ( #17806, #20584 ),
 ( #20292, #29819 ),
 ( #8601, #18109 ),
 ( #22929, #27624 ),
 ( #1581, #23221 ),
 ( #11691, #11548 ),
 ( #27354, #21038 ),
 ( #21180, #25888 ),
 ( #18569, #4979 ),
 ( #6852, #9199 ),
 ( #21347, #11850 ),
 ( #2323, #140 ),
 ( #19169, #9659 ),
 ( #18711, #30559 ),
 ( #25731, #28219 ),
 ( #26188, #28387 ),
 ( #9053, #9504 ),
 ( #16373, #7168 ),
 ( #1875, #28077 ) ),
 .UNSPECIFIED., .F., .F., .F.,
 ( 4, 3, 3, 3, 3, 3, 3, 3, 3, 3, 4 ),
 ( 2, 2 ),
 ( 0.000000000000000000, 0.05425176834609614362, 0.1085332949128348518, 0.1623767749169379715, 0.2157504826133058717, 0.2688657508888169789, 0.3218907763505471364, 0.3749548578363334772, 0.4282048033836237666, 0.4818374082110496448, 0.4999999999131653494 ),
 ( 0.000000000000000000, 1.000000000000000000 ),
 .UNSPECIFIED. ) ;
#16137=AXIS2_PLACEMENT_3D ( 'NONE', #1635, #8962, #6611 ) ;
#16139=CARTESIAN_POINT ( 'NONE',  ( -10.14013680258725358, -17.25966085745526968, 5.749491821935610147 ) ) ;
#16141=ORIENTED_EDGE ( 'NONE', *, *, #4314, .F. ) ;
#16143=CARTESIAN_POINT ( 'NONE',  ( 0.4564504349074350875, -9.471281197126604212, 13.00000000000000178 ) ) ;
#16147=PLANE ( 'NONE',  #25789 ) ;
#16148=LINE ( 'NONE', #6487, #21998 ) ;
#16149=CARTESIAN_POINT ( 'NONE',  ( 3.068634486552013207, 16.80010772488889614, 19.21769074125272780 ) ) ;
#16150=CARTESIAN_POINT ( 'NONE',  ( -18.40637697828373121, -7.823545570387635983, 19.85261563089511228 ) ) ;
#16155=ORIENTED_EDGE ( 'NONE', *, *, #9417, .T. ) ;
#16159=CARTESIAN_POINT ( 'NONE',  ( -7.785146467913381052, -15.19543897952354783, 6.147510495896840510 ) ) ;
#16163=CARTESIAN_POINT ( 'NONE',  ( 15.48289691231202703, -7.082479268569363384, 18.71435384576123440 ) ) ;
#16164=CARTESIAN_POINT ( 'NONE',  ( 4.155601639749240128, 16.52779251924068760, 5.657991946698900598 ) ) ;
#16174=CARTESIAN_POINT ( 'NONE',  ( -14.67633008511251091, 13.58695459845237075, 6.781503518395064489 ) ) ;
#16183=CARTESIAN_POINT ( 'NONE',  ( -19.95735252415838090, 1.552219945263927592, 19.69140814234746273 ) ) ;
#16186=CARTESIAN_POINT ( 'NONE',  ( 10.38186781339405229, -13.54365823448425843, 20.13759033520874908 ) ) ;
#16197=EDGE_LOOP ( 'NONE', ( #428, #12578, #25618, #18624 ) ) ;
#16200=ORIENTED_EDGE ( 'NONE', *, *, #16237, .T. ) ;
#16204=ORIENTED_EDGE ( 'NONE', *, *, #4110, .F. ) ;
#16205=VERTEX_POINT ( 'NONE', #26760 ) ;
#16207=CARTESIAN_POINT ( 'NONE',  ( -0.1008988851360398120, -17.02363397670899303, 18.83976166372256600 ) ) ;
#16212=CYLINDRICAL_SURFACE ( 'NONE', #16350, 0.7499999999999997780 ) ;
#16215=ADVANCED_FACE ( 'NONE', ( #3352 ), #856, .F. ) ;
#16216=CARTESIAN_POINT ( 'NONE',  ( -19.81665592078380200, 2.832673353242753933, 18.39701043959520987 ) ) ;
#16218=CARTESIAN_POINT ( 'NONE',  ( -15.40257881337303481, 12.78582346615753629, 20.34789198813115263 ) ) ;
#16219=CARTESIAN_POINT ( 'NONE',  ( 4.537370253389201302, 19.49663512434673507, 19.97651184436794125 ) ) ;
#16224=EDGE_CURVE ( 'NONE', #13283, #29319, #11700, .T. ) ;
#16228=DIRECTION ( 'NONE',  ( -0.000000000000000000, -0.000000000000000000, 1.000000000000000000 ) ) ;
#16231=ORIENTED_EDGE ( 'NONE', *, *, #12650, .T. ) ;
#16232=CARTESIAN_POINT ( 'NONE',  ( -17.03551135121416849, 1.010186107319479554, 5.872146474157316831 ) ) ;
#16233=ADVANCED_FACE ( 'NONE', ( #16933 ), #7580, .F. ) ;
#16235=DIRECTION ( 'NONE',  ( -0.000000000000000000, -0.000000000000000000, 1.000000000000000000 ) ) ;
#16236=VERTEX_POINT ( 'NONE', #24094 ) ;
#16237=EDGE_CURVE ( 'NONE', #10573, #6567, #29094, .T. ) ;
#16240=CARTESIAN_POINT ( 'NONE',  ( 16.09309408545198039, -5.686824080536031722, 5.951255046771932733 ) ) ;
#16244=CARTESIAN_POINT ( 'NONE',  ( 7.730328572437743517, -4.608906612435629491, 21.50000000000000000 ) ) ;
#16248=CARTESIAN_POINT ( 'NONE',  ( -5.615427697021304176, 16.09608755218562948, 20.34789198813115263 ) ) ;
#16250=AXIS2_PLACEMENT_3D ( 'NONE', #6910, #1919, #9096 ) ;
#16255=EDGE_CURVE ( 'NONE', #12567, #28158, #3049, .T. ) ;
#16257=DIRECTION ( 'NONE',  ( 1.000000000000000000, 0.000000000000000000, 0.000000000000000000 ) ) ;
#16259=EDGE_LOOP ( 'NONE', ( #8220, #11986, #5443, #27907 ) ) ;
#16261=AXIS2_PLACEMENT_3D ( 'NONE', #24902, #27089, #8539 ) ;
#16262=CARTESIAN_POINT ( 'NONE',  ( -14.77047757180929466, -8.563270617688839792, 18.82680253904184298 ) ) ;
#16263=CIRCLE ( 'NONE', #2821, 9.482273699623480212 ) ;
#16266=AXIS2_PLACEMENT_3D ( 'NONE', #4729, #6198, #23910 ) ;
#16273=CARTESIAN_POINT ( 'NONE',  ( -6.096671963363472280, 19.04856480014128195, 7.652108011868850035 ) ) ;
#16275=B_SPLINE_CURVE_WITH_KNOTS ( 'NONE', 3,
 ( #297, #9819, #19333, #2185, #9209, #18441, #11703, #28235, #27943, #8919, #18119, #15771, #9064, #25601, #27635, #22940, #13457, #13741 ),
 .UNSPECIFIED., .F., .F.,
 ( 4, 2, 2, 2, 2, 2, 2, 2, 4 ),
 ( 0.003174295595554294403, 0.003570702171545527166, 0.003967108747536760363, 0.004363515323527992693, 0.004759921899519225889, 0.005156328475510459086, 0.005552735051501691416, 0.005949141627492923745, 0.006345548203484156942 ),
 .UNSPECIFIED. ) ;
#16279=DIRECTION ( 'NONE',  ( 0.9594929736144952592, -0.2817325568414371095, 0.000000000000000000 ) ) ;
#16281=ORIENTED_EDGE ( 'NONE', *, *, #14489, .T. ) ;
#16283=CARTESIAN_POINT ( 'NONE',  ( 16.16296542101254730, 5.939519782021115191, 1.500000000000000000 ) ) ;
#16284=VERTEX_POINT ( 'NONE', #25799 ) ;
#16285=DIRECTION ( 'NONE',  ( -0.000000000000000000, -0.000000000000000000, 1.000000000000000000 ) ) ;
#16286=VECTOR ( 'NONE', #4237, 1000.000000000000000 ) ;
#16289=CARTESIAN_POINT ( 'NONE',  ( -7.809214384344188353, -15.18204291278972029, 7.196036389296800451 ) ) ;
#16290=EDGE_CURVE ( 'NONE', #21154, #15490, #29139, .T. ) ;
#16295=CARTESIAN_POINT ( 'NONE',  ( 18.64396409872436777, -7.239577540284316548, 7.272192800924339728 ) ) ;
#16296=CARTESIAN_POINT ( 'NONE',  ( -4.163336342344337027E-14, 1.387778780781445676E-14, 1.500000000000000000 ) ) ;
#16298=CARTESIAN_POINT ( 'NONE',  ( -13.35701160122519404, 10.58771215013900857, 18.34777357837152323 ) ) ;
#16299=VERTEX_POINT ( 'NONE', #6617 ) ;
#16302=DIRECTION ( 'NONE',  ( -0.000000000000000000, -0.000000000000000000, 1.000000000000000000 ) ) ;
#16305=CARTESIAN_POINT ( 'NONE',  ( -18.25569084301827161, -8.169747224523364437, 18.47110296274026098 ) ) ;
#16306=CIRCLE ( 'NONE', #2858, 9.482273699623480212 ) ;
#16307=CARTESIAN_POINT ( 'NONE',  ( -18.39183130958319978, -7.903152449895381793, 19.96783386855779341 ) ) ;
#16308=DIRECTION ( 'NONE',  ( -0.9096319953545185522, 0.4154150130018859355, 0.000000000000000000 ) ) ;
#16310=ORIENTED_EDGE ( 'NONE', *, *, #24044, .T. ) ;
#16311=ORIENTED_EDGE ( 'NONE', *, *, #21608, .F. ) ;
#16314=CARTESIAN_POINT ( 'NONE',  ( -7.695850205876553218, -15.24499612924144465, 6.917457548096560771 ) ) ;
#16316=ORIENTED_EDGE ( 'NONE', *, *, #20649, .T. ) ;
#16319=CARTESIAN_POINT ( 'NONE',  ( -5.544451647051928944, 16.11829164193971664, 20.34789198813115263 ) ) ;
#16323=CARTESIAN_POINT ( 'NONE',  ( -16.83986259902030014, 2.499865191129254871, 6.111214848085761986 ) ) ;
#16324=CARTESIAN_POINT ( 'NONE',  ( 14.53258460577762889, 13.76634464516646617, 7.500147780736496017 ) ) ;
#16330=CARTESIAN_POINT ( 'NONE',  ( -14.71865621671073932, -8.659590923291235143, 6.392658652357120275 ) ) ;
#16332=VECTOR ( 'NONE', #4933, 1000.000000000000000 ) ;
#16333=ADVANCED_FACE ( 'NONE', ( #28444 ), #23439, .F. ) ;
#16334=ORIENTED_EDGE ( 'NONE', *, *, #4245, .F. ) ;
#16335=CIRCLE ( 'NONE', #26226, 0.7500000000000002220 ) ;
#16337=CARTESIAN_POINT ( 'NONE',  ( 16.87629972246788768, 2.221555249144609334, 19.08155846658118904 ) ) ;
#16342=CARTESIAN_POINT ( 'NONE',  ( 5.352643706120459477, 7.827050521741900191, 1.500000000000001332 ) ) ;
#16344=CARTESIAN_POINT ( 'NONE',  ( -9.406652940105978189, 1.195154792889487227, 21.50000000000000000 ) ) ;
#16345=ORIENTED_EDGE ( 'NONE', *, *, #15276, .F. ) ;
#16346=CIRCLE ( 'NONE', #13374, 0.7499999999999997780 ) ;
#16348=CARTESIAN_POINT ( 'NONE',  ( 11.89619695863782667, -16.09924856797056947, 19.69140814234746273 ) ) ;
#16350=AXIS2_PLACEMENT_3D ( 'NONE', #16521, #18873, #14172 ) ;
#16351=ORIENTED_EDGE ( 'NONE', *, *, #770, .T. ) ;
#16352=ORIENTED_EDGE ( 'NONE', *, *, #18174, .F. ) ;
#16360=CARTESIAN_POINT ( 'NONE',  ( 8.430595340551262140, -4.340342926364987086, 1.500000000000001332 ) ) ;
#16362=VERTEX_POINT ( 'NONE', #28594 ) ;
#16370=CARTESIAN_POINT ( 'NONE',  ( -0.02429396246983370547, -17.02566277816918117, 18.72771030977187934 ) ) ;
#16372=CARTESIAN_POINT ( 'NONE',  ( -8.999114229549592281, 0.1262659238205133538, 1.500000000000001332 ) ) ;
#16373=CARTESIAN_POINT ( 'NONE',  ( 19.76665705046225696, 3.161078882829539971, 18.34777357837152323 ) ) ;
#16375=CARTESIAN_POINT ( 'NONE',  ( -19.86132377132436488, 2.497833445081384607, 18.34798005862930381 ) ) ;
#16377=DIRECTION ( 'NONE',  ( -0.000000000000000000, -0.000000000000000000, 1.000000000000000000 ) ) ;
#16378=VERTEX_POINT ( 'NONE', #7218 ) ;
#16381=DIRECTION ( 'NONE',  ( 0.000000000000000000, 0.000000000000000000, 1.000000000000000000 ) ) ;
#16383=CYLINDRICAL_SURFACE ( 'NONE', #21315, 20.00000000000000000 ) ;
#16387=CARTESIAN_POINT ( 'NONE',  ( -5.000852292258042731, 19.36469665082833203, 6.781503518395070707 ) ) ;
#16389=CARTESIAN_POINT ( 'NONE',  ( -17.05973338880502865, 0.7261025713186443076, 6.233981582756856987 ) ) ;
#16391=CARTESIAN_POINT ( 'NONE',  ( 14.88222593340886668, 13.36111339922579866, 20.34789198813115263 ) ) ;
#16392=CARTESIAN_POINT ( 'NONE',  ( -6.437683520590124608, 6.962021646281596254, 13.00000000000000178 ) ) ;
#16395=ORIENTED_EDGE ( 'NONE', *, *, #12646, .T. ) ;
#16396=PLANE ( 'NONE',  #14423 ) ;
#16397=CARTESIAN_POINT ( 'NONE',  ( 11.10715495309693424, -16.63223102436629475, 20.34789198813115263 ) ) ;
#16398=EDGE_CURVE ( 'NONE', #7304, #13794, #10208, .T. ) ;
#16404=CARTESIAN_POINT ( 'NONE',  ( -18.25684187146043413, -8.167166100028891762, 7.526993102356321685 ) ) ;
#16408=CARTESIAN_POINT ( 'NONE',  ( -6.187077094091591789, 11.47693674426096955, 24.50000000000000000 ) ) ;
#16411=CARTESIAN_POINT ( 'NONE',  ( 15.38599937579231103, -7.279790735017091841, 6.714907520933426355 ) ) ;
#16419=CARTESIAN_POINT ( 'NONE',  ( -18.06093561247158519, -8.632161831585831280, 20.34789198813115263 ) ) ;
#16422=VECTOR ( 'NONE', #6641, 1000.000000000000000 ) ;
#16425=CARTESIAN_POINT ( 'NONE',  ( 2.352830851074115159, 9.185733585337917617, 21.50000000000000000 ) ) ;
#16428=DIRECTION ( 'NONE',  ( -0.000000000000000000, -0.000000000000000000, -1.000000000000000000 ) ) ;
#16430=CARTESIAN_POINT ( 'NONE',  ( -13.93204262646994529, 9.869472133046889084, 7.158811349119583944 ) ) ;
#16432=FACE_OUTER_BOUND ( 'NONE', #21744, .T. ) ;
#16435=ORIENTED_EDGE ( 'NONE', *, *, #18571, .F. ) ;
#16436=ADVANCED_FACE ( 'NONE', ( #29055 ), #24518, .F. ) ;
#16437=CARTESIAN_POINT ( 'NONE',  ( 8.840471615930072247, -1.687027447297460236, 21.50000000000000000 ) ) ;
#16438=EDGE_CURVE ( 'NONE', #27530, #23584, #15163, .T. ) ;
#16440=ORIENTED_EDGE ( 'NONE', *, *, #4209, .F. ) ;
#16441=CARTESIAN_POINT ( 'NONE',  ( 0.2430132208050651554, -17.02994525543106263, 18.49267272388512140 ) ) ;
#16443=CARTESIAN_POINT ( 'NONE',  ( -9.833673822381062024, -17.43574673801737163, 6.041646659195333058 ) ) ;
#16445=CARTESIAN_POINT ( 'NONE',  ( 0.7902931953360861073, -20.00234323981188922, 20.25542030744407640 ) ) ;
#16448=CARTESIAN_POINT ( 'NONE',  ( 18.71865409427298843, -7.043577866502358731, 6.523620417364442758 ) ) ;
#16449=CARTESIAN_POINT ( 'NONE',  ( 4.390207617113956573, -7.856594496258208160, 1.500000000000001332 ) ) ;
#16450=CARTESIAN_POINT ( 'NONE',  ( 11.66141461333273099, 12.47704237144457551, 19.47783254395485031 ) ) ;
#16451=CYLINDRICAL_SURFACE ( 'NONE', #19115, 0.7499999999999997780 ) ;
#16454=DIRECTION ( 'NONE',  ( 1.000000000000000000, 0.000000000000000000, 0.000000000000000000 ) ) ;
#16455=CARTESIAN_POINT ( 'NONE',  ( -12.97606618386100585, 11.02883152172955938, 18.54473042795395443 ) ) ;
#16457=CARTESIAN_POINT ( 'NONE',  ( 4.045242219987651211, 16.55840560649980731, 18.34798005863078885 ) ) ;
#16459=DIRECTION ( 'NONE',  ( -0.6548607339452851006, -0.7557495743542582689, 0.000000000000000000 ) ) ;
#16465=CARTESIAN_POINT ( 'NONE',  ( -8.546423435383420752, -14.74799740001550141, 5.652196082368483587 ) ) ;
#16466=EDGE_CURVE ( 'NONE', #10973, #26160, #27032, .T. ) ;
#16468=CARTESIAN_POINT ( 'NONE',  ( 11.22181534970139083, -16.55562029408562807, 18.34869673959212122 ) ) ;
#16470=CARTESIAN_POINT ( 'NONE',  ( -6.812559277181930106, 5.881244434206302607, 1.500000000000001332 ) ) ;
#16471=CARTESIAN_POINT ( 'NONE',  ( 6.124711512895117060, 19.05797279266333888, 6.111214848085761986 ) ) ;
#16474=CARTESIAN_POINT ( 'NONE',  ( 4.964892671625812604, 16.28226395658651171, 19.00652017443069752 ) ) ;
#16475=EDGE_CURVE ( 'NONE', #28836, #8257, #13201, .T. ) ;
#16476=CARTESIAN_POINT ( 'NONE',  ( 11.65981318837299341, 12.47865322263302978, 6.672349528511551497 ) ) ;
#16477=DIRECTION ( 'NONE',  ( -0.2817325568414293380, -0.9594929736144974797, 0.000000000000000000 ) ) ;
#16479=EDGE_LOOP ( 'NONE', ( #11072, #4236, #6065, #29320 ) ) ;
#16482=DIRECTION ( 'NONE',  ( -0.000000000000000000, -0.000000000000000000, 1.000000000000000000 ) ) ;
#16485=VERTEX_POINT ( 'NONE', #9711 ) ;
#16490=CARTESIAN_POINT ( 'NONE',  ( -0.02177409673011703947, -17.02558975896787885, 7.272049892295485485 ) ) ;
#16493=CARTESIAN_POINT ( 'NONE',  ( -17.04208893090348198, 0.9369385374313018433, 20.06253562465620632 ) ) ;
#16496=CARTESIAN_POINT ( 'NONE',  ( -6.507549961782351566, 15.78987431823413168, 6.588756557121048907 ) ) ;
#16503=EDGE_LOOP ( 'NONE', ( #5023, #9902, #9300, #26586 ) ) ;
#16507=CARTESIAN_POINT ( 'NONE',  ( 18.69797757513549996, -7.147916136757722860, 19.79423548914561692 ) ) ;
#16508=CARTESIAN_POINT ( 'NONE',  ( 16.57326105224177581, 4.109591991357616436, 18.92976555901915603 ) ) ;
#16512=AXIS2_PLACEMENT_3D ( 'NONE', #7326, #11546, #18709 ) ;
#16516=CARTESIAN_POINT ( 'NONE',  ( 0.1595703637281291887, -17.02896808596822709, 20.14907003336613300 ) ) ;
#16518=CARTESIAN_POINT ( 'NONE',  ( 1.780236034000288736, -16.98472935612792156, 6.447548852708279377 ) ) ;
#16519=DIRECTION ( 'NONE',  ( 1.000000000000000000, 0.000000000000000000, 0.000000000000000000 ) ) ;
#16520=CARTESIAN_POINT ( 'NONE',  ( 7.028330626922776325, 10.93629592680536966, 1.500000000000001332 ) ) ;
#16521=CARTESIAN_POINT ( 'NONE',  ( 2.959227181723801170, -8.499586724479446076, 1.500000000000001332 ) ) ;
#16522=ORIENTED_EDGE ( 'NONE', *, *, #13837, .T. ) ;
#16527=ORIENTED_EDGE ( 'NONE', *, *, #23679, .F. ) ;
#16532=CARTESIAN_POINT ( 'NONE',  ( -5.978582851986702806, 19.10413308555695622, 18.34798005862930381 ) ) ;
#16537=CARTESIAN_POINT ( 'NONE',  ( -17.01545599012841237, 1.214108451629968055, 7.559636331181775581 ) ) ;
#16538=LINE ( 'NONE', #14043, #3760 ) ;
#16539=CARTESIAN_POINT ( 'NONE',  ( 6.962021646281529641, 6.437683520590196551, 21.50000000000000000 ) ) ;
#16542=ORIENTED_EDGE ( 'NONE', *, *, #20992, .T. ) ;
#16545=DIRECTION ( 'NONE',  ( 0.000000000000000000, 0.000000000000000000, 1.000000000000000000 ) ) ;
#16546=ORIENTED_EDGE ( 'NONE', *, *, #17216, .T. ) ;
#16549=VECTOR ( 'NONE', #7289, 1000.000000000000000 ) ;
#16551=CARTESIAN_POINT ( 'NONE',  ( -15.16307827826492449, -7.786259562520723598, 18.34798005863078885 ) ) ;
#16552=CARTESIAN_POINT ( 'NONE',  ( -6.426383236738485216, 15.81971323177987898, 18.92976555901915603 ) ) ;
#16554=LINE ( 'NONE', #16408, #402 ) ;
#16556=CARTESIAN_POINT ( 'NONE',  ( 15.81223572262637589, -6.365019322297389870, 7.652108011868850923 ) ) ;
#16563=LINE ( 'NONE', #28432, #11742 ) ;
#16565=FACE_OUTER_BOUND ( 'NONE', #4958, .T. ) ;
#16569=EDGE_CURVE ( 'NONE', #28836, #154, #3782, .T. ) ;
#16575=ORIENTED_EDGE ( 'NONE', *, *, #1567, .F. ) ;
#16583=DIRECTION ( 'NONE',  ( 0.000000000000000000, 0.000000000000000000, 1.000000000000000000 ) ) ;
#16586=CARTESIAN_POINT ( 'NONE',  ( -0.07785784566753434222, -17.02422498921964689, 18.80699882434806369 ) ) ;
#16588=CARTESIAN_POINT ( 'NONE',  ( -8.172867764805141988, -14.97344430594796272, 7.559636331181775581 ) ) ;
#16590=CARTESIAN_POINT ( 'NONE',  ( 1.797484530300065053, -16.98352104300882459, 19.25672174529527325 ) ) ;
#16595=CARTESIAN_POINT ( 'NONE',  ( 14.26939381558975839, 14.03892697587676963, 19.79423548914561692 ) ) ;
#16599=EDGE_CURVE ( 'NONE', #21613, #6566, #7242, .T. ) ;
#16601=CARTESIAN_POINT ( 'NONE',  ( -14.87733195063809966, -8.360270151095063440, 5.872146474157316831 ) ) ;
#16602=CARTESIAN_POINT ( 'NONE',  ( 7.827050521741877098, -5.352643706120495004, 13.00000000000000178 ) ) ;
#16604=CARTESIAN_POINT ( 'NONE',  ( -18.45589647530844957, -7.705834498630346197, 19.47728749465736442 ) ) ;
#16608=CARTESIAN_POINT ( 'NONE',  ( 9.864937699929955173, -13.90063973435163724, 5.652196082368482699 ) ) ;
#16612=LINE ( 'NONE', #18358, #6967 ) ;
#16617=CARTESIAN_POINT ( 'NONE',  ( 11.93826604606910990, -16.04611492155650865, 19.48477075383301127 ) ) ;
#16618=VERTEX_POINT ( 'NONE', #24986 ) ;
#16621=CARTESIAN_POINT ( 'NONE',  ( -5.796781398543691566, 16.03935303270020185, 20.34789198813114552 ) ) ;
#16622=CARTESIAN_POINT ( 'NONE',  ( 6.218621694205430650, 19.02754758079138853, 6.310736198168394928 ) ) ;
#16623=EDGE_CURVE ( 'NONE', #4949, #13171, #20001, .T. ) ;
#16624=AXIS2_PLACEMENT_3D ( 'NONE', #19178, #16381, #2648 ) ;
#16626=ORIENTED_EDGE ( 'NONE', *, *, #2561, .F. ) ;
#16627=CIRCLE ( 'NONE', #5615, 0.7499999999999988898 ) ;
#16628=CARTESIAN_POINT ( 'NONE',  ( 5.997818345539173812, 19.09841206584651729, 20.05479082170252525 ) ) ;
#16629=CARTESIAN_POINT ( 'NONE',  ( 14.19872765237045087, 14.11031447301239616, 6.672349528511551497 ) ) ;
#16631=FACE_OUTER_BOUND ( 'NONE', #25118, .T. ) ;
#16635=EDGE_CURVE ( 'NONE', #13230, #5725, #10801, .T. ) ;
#16640=ORIENTED_EDGE ( 'NONE', *, *, #7260, .F. ) ;
#16641=CARTESIAN_POINT ( 'NONE',  ( -18.41388790264793940, -7.851569931599772012, 6.111214848085761986 ) ) ;
#16644=CARTESIAN_POINT ( 'NONE',  ( 0.5572578986459522099, -17.03042415120789954, 5.670038381137163519 ) ) ;
#16651=ADVANCED_FACE ( 'NONE', ( #18284 ), #6432, .F. ) ;
#16653=CARTESIAN_POINT ( 'NONE',  ( 9.922755320353058295, -13.86203410616581522, 20.34789198813115263 ) ) ;
#16654=PLANE ( 'NONE',  #8604 ) ;
#16657=ORIENTED_EDGE ( 'NONE', *, *, #18947, .F. ) ;
#16658=CARTESIAN_POINT ( 'NONE',  ( 4.307942169702174695, 19.53053083060025230, 19.21940439362674624 ) ) ;
#16664=CARTESIAN_POINT ( 'NONE',  ( 16.19464367748837219, -5.422319245274325183, 19.36813350477385143 ) ) ;
#16665=CARTESIAN_POINT ( 'NONE',  ( 16.57618148055192009, 4.095680178559272022, 19.79423548914561692 ) ) ;
#16666=DIRECTION ( 'NONE',  ( 0.000000000000000000, 0.000000000000000000, 1.000000000000000000 ) ) ;
#16668=CARTESIAN_POINT ( 'NONE',  ( 9.249586724479433641, 2.959227181723830036, 1.500000000000001332 ) ) ;
#16670=ORIENTED_EDGE ( 'NONE', *, *, #29023, .T. ) ;
#16673=CARTESIAN_POINT ( 'NONE',  ( 7.548823014270646503, -5.738360882149970976, 13.00000000000000178 ) ) ;
#16674=CARTESIAN_POINT ( 'NONE',  ( -17.76524000349413868, -9.187221810585024073, 5.853797745100182581 ) ) ;
#16675=EDGE_CURVE ( 'NONE', #24160, #10973, #7870, .T. ) ;
#16676=CARTESIAN_POINT ( 'NONE',  ( 1.316598178790385321, -17.01073877869967887, 7.500147780736496017 ) ) ;
#16677=CARTESIAN_POINT ( 'NONE',  ( -15.04923167470879797, -8.024232118851555740, 18.34938820207544907 ) ) ;
#16678=CARTESIAN_POINT ( 'NONE',  ( 1.588511040599926760, -16.99700008609428181, 19.96568007040468373 ) ) ;
#16681=CARTESIAN_POINT ( 'NONE',  ( 10.50588106577561653, -17.03964880432503293, 7.359006845440219102 ) ) ;
#16683=CARTESIAN_POINT ( 'NONE',  ( -13.71804704112738982, 10.14464636835443123, 7.500147780736496017 ) ) ;
#16687=VECTOR ( 'NONE', #13500, 1000.000000000000000 ) ;
#16690=PLANE ( 'NONE',  #15332 ) ;
#16691=CARTESIAN_POINT ( 'NONE',  ( -5.225937649208972857, 16.21530267322276586, 18.39701043959520987 ) ) ;
#16692=CARTESIAN_POINT ( 'NONE',  ( -15.56680656382032168, -6.886169722869405874, 6.385774490351136201 ) ) ;
#16696=CARTESIAN_POINT ( 'NONE',  ( 0.6154569680868984261, -19.99089747819056129, 7.626218077512941562 ) ) ;
#16697=CARTESIAN_POINT ( 'NONE',  ( -17.58178100985203685, -9.533151461302381335, 19.48477075383300772 ) ) ;
#16699=ORIENTED_EDGE ( 'NONE', *, *, #5162, .F. ) ;
#16700=CARTESIAN_POINT ( 'NONE',  ( 12.51082390549571421, 11.56795297236522657, 7.632642797338977658 ) ) ;
#16702=CARTESIAN_POINT ( 'NONE',  ( 18.62671295915898639, -7.331958482175751080, 7.366751648393900176 ) ) ;
#16710=EDGE_CURVE ( 'NONE', #6692, #19471, #2759, .T. ) ;
#16713=LINE ( 'NONE', #13920, #15334 ) ;
#16714=ORIENTED_EDGE ( 'NONE', *, *, #25270, .F. ) ;
#16723=B_SPLINE_CURVE_WITH_KNOTS ( 'NONE', 3,
 ( #7420, #16468, #9604, #21598, #9455, #8884, #14259, #28631, #25983, #16617, #18971, #2260, #23940, #25417, #2740, #19113, #235, #16928 ),
 .UNSPECIFIED., .F., .F.,
 ( 4, 2, 2, 2, 2, 2, 2, 2, 4 ),
 ( 0.000000000000000000, 0.0003967869494442910830, 0.0007935738988885821660, 0.001190360848332873249, 0.001587147797777164332, 0.001983934747221455415, 0.002380721696665746498, 0.002777508646110037581, 0.003174295595554328664 ),
 .UNSPECIFIED. ) ;
#16724=CARTESIAN_POINT ( 'NONE',  ( 4.823417668075713927, 16.32807078414248991, 7.267659094423558841 ) ) ;
#16725=DIRECTION ( 'NONE',  ( 1.000000000000000000, 0.000000000000000000, 0.000000000000000000 ) ) ;
#16728=CARTESIAN_POINT ( 'NONE',  ( -6.458857079295999171, 18.92875833827542209, 5.779535427900762024 ) ) ;
#16731=CARTESIAN_POINT ( 'NONE',  ( -3.196529495465446402, -8.413215745754985875, 21.50000000000000000 ) ) ;
#16735=DIRECTION ( 'NONE',  ( 1.000000000000000000, 0.000000000000000000, 0.000000000000000000 ) ) ;
#16736=AXIS2_PLACEMENT_3D ( 'NONE', #30830, #16032, #23186 ) ;
#16737=ORIENTED_EDGE ( 'NONE', *, *, #575, .T. ) ;
#16739=CARTESIAN_POINT ( 'NONE',  ( 0.3493064693810321586, -20.01473674030432193, 20.34789198813115263 ) ) ;
#16741=CYLINDRICAL_SURFACE ( 'NONE', #16845, 0.7500000000000006661 ) ;
#16746=CARTESIAN_POINT ( 'NONE',  ( 11.73047935159229027, 12.40726572549739615, 19.79423548914561692 ) ) ;
#16750=AXIS2_PLACEMENT_3D ( 'NONE', #25142, #22345, #24846 ) ;
#16752=CARTESIAN_POINT ( 'NONE',  ( -15.71962203721309592, -1.249857212218242752, -0.6213203435596476032 ) ) ;
#16753=DIRECTION ( 'NONE',  ( 1.000000000000000000, 0.000000000000000000, 0.000000000000000000 ) ) ;
#16757=EDGE_CURVE ( 'NONE', #2810, #950, #16538, .T. ) ;
#16759=VECTOR ( 'NONE', #23928, 1000.000000000000000 ) ;
#16760=ORIENTED_EDGE ( 'NONE', *, *, #8243, .F. ) ;
#16764=CARTESIAN_POINT ( 'NONE',  ( -7.850819104130406068, -15.15878979527105841, 6.037360021877317351 ) ) ;
#16769=FACE_OUTER_BOUND ( 'NONE', #16964, .T. ) ;
#16770=VECTOR ( 'NONE', #3051, 1000.000000000000000 ) ;
#16771=CARTESIAN_POINT ( 'NONE',  ( 4.659914667891708717, 16.37914622779767981, 7.429667576816606278 ) ) ;
#16773=VERTEX_POINT ( 'NONE', #26056 ) ;
#16774=CARTESIAN_POINT ( 'NONE',  ( 5.828790066614889298, 19.15065750257362609, 20.19668224736330941 ) ) ;
#16776=AXIS2_PLACEMENT_3D ( 'NONE', #6948, #10590, #8254 ) ;
#16777=DIRECTION ( 'NONE',  ( -0.000000000000000000, -0.000000000000000000, -1.000000000000000000 ) ) ;
#16783=DIRECTION ( 'NONE',  ( 1.000000000000000000, 0.000000000000000000, 0.000000000000000000 ) ) ;
#16789=PLANE ( 'NONE',  #11370 ) ;
#16792=CARTESIAN_POINT ( 'NONE',  ( -0.1765357775187666733, -17.02148976770177669, 6.310736198168394928 ) ) ;
#16795=AXIS2_PLACEMENT_3D ( 'NONE', #7402, #2719, #7232 ) ;
#16805=ORIENTED_EDGE ( 'NONE', *, *, #26164, .T. ) ;
#16817=CARTESIAN_POINT ( 'NONE',  ( 16.11883921216212201, -5.620554474281627577, 18.73743063545763121 ) ) ;
#16820=DIRECTION ( 'NONE',  ( 0.000000000000000000, 0.000000000000000000, -1.000000000000000000 ) ) ;
#16821=ORIENTED_EDGE ( 'NONE', *, *, #13732, .T. ) ;
#16822=VECTOR ( 'NONE', #27265, 1000.000000000000000 ) ;
#16823=CARTESIAN_POINT ( 'NONE',  ( -2.523760598493569596, 1.621922452366830747, 24.50000000000000000 ) ) ;
#16824=ADVANCED_FACE ( 'NONE', ( #5149 ), #12649, .F. ) ;
#16826=EDGE_CURVE ( 'NONE', #15068, #9540, #10290, .T. ) ;
#16827=ADVANCED_FACE ( 'NONE', ( #19186, #2978, #9834 ), #12495, .T. ) ;
#16828=EDGE_LOOP ( 'NONE', ( #6244, #22320, #22626, #15543 ) ) ;
#16829=EDGE_CURVE ( 'NONE', #28720, #27915, #5734, .T. ) ;
#16831=CARTESIAN_POINT ( 'NONE',  ( -12.77302042131097792, 11.25334833650868838, 19.77662771831109367 ) ) ;
#16833=VECTOR ( 'NONE', #9235, 1000.000000000000000 ) ;
#16834=CARTESIAN_POINT ( 'NONE',  ( -8.546421331151638157, -14.74799399427946156, 18.34798005862662507 ) ) ;
#16835=CARTESIAN_POINT ( 'NONE',  ( 16.16296542101254730, 5.939519782021115191, 24.50000000000000000 ) ) ;
#16840=CARTESIAN_POINT ( 'NONE',  ( -16.86382086101523470, 2.355052171780695591, 18.63641924841378028 ) ) ;
#16842=DIRECTION ( 'NONE',  ( 0.000000000000000000, 0.000000000000000000, 1.000000000000000000 ) ) ;
#16845=AXIS2_PLACEMENT_3D ( 'NONE', #26424, #14086, #14414 ) ;
#16849=CARTESIAN_POINT ( 'NONE',  ( 18.57699708025014829, -7.409721753143986511, 18.54958172136249672 ) ) ;
#16850=CARTESIAN_POINT ( 'NONE',  ( -15.22163550579135283, -7.663797071142820272, 7.652108011868851811 ) ) ;
#16852=CARTESIAN_POINT ( 'NONE',  ( -5.378544123449405134, 19.26344156360741167, 7.454139397117727661 ) ) ;
#16853=EDGE_CURVE ( 'NONE', #24237, #23890, #26818, .T. ) ;
#16854=ORIENTED_EDGE ( 'NONE', *, *, #20077, .T. ) ;
#16859=CARTESIAN_POINT ( 'NONE',  ( -17.92868989761418419, -8.864358285757582223, 20.32200205377525393 ) ) ;
#16862=CARTESIAN_POINT ( 'NONE',  ( 12.91913032519424398, 11.08701612049550178, 7.176035686813569292 ) ) ;
#16864=CARTESIAN_POINT ( 'NONE',  ( 15.89967663190788905, -6.161197767010750503, 7.627891251804737927 ) ) ;
#16865=CARTESIAN_POINT ( 'NONE',  ( 9.755064781586030520, 13.32952022457704544, 1.500000000000000000 ) ) ;
#16869=CARTESIAN_POINT ( 'NONE',  ( 10.66613195287592752, -13.33645323721078668, 19.08844262864050023 ) ) ;
#16870=CARTESIAN_POINT ( 'NONE',  ( -18.09892777451933554, -8.511549950051181312, 5.651480102388684479 ) ) ;
#16874=ORIENTED_EDGE ( 'NONE', *, *, #14707, .F. ) ;
#16882=CARTESIAN_POINT ( 'NONE',  ( 0.000000000000000000, 0.000000000000000000, 21.50000000000000000 ) ) ;
#16889=CARTESIAN_POINT ( 'NONE',  ( 0.3567147238643519902, -19.99681861211371370, 18.34798005863226678 ) ) ;
#16892=CARTESIAN_POINT ( 'NONE',  ( 19.74251403343738076, 3.198927889078825970, 5.652196082369965069 ) ) ;
#16895=DIRECTION ( 'NONE',  ( 1.000000000000000000, 0.000000000000000000, 0.000000000000000000 ) ) ;
#16899=ORIENTED_EDGE ( 'NONE', *, *, #11693, .F. ) ;
#16901=CARTESIAN_POINT ( 'NONE',  ( -9.815074746723995602, -17.42621888692031007, 6.037995405461177079 ) ) ;
#16906=CARTESIAN_POINT ( 'NONE',  ( -0.1834311997418882345, -17.02123387943971977, 19.66989035740801839 ) ) ;
#16907=CARTESIAN_POINT ( 'NONE',  ( -9.895604986052594754, -17.40083251127919084, 5.951255046771932733 ) ) ;
#16909=CARTESIAN_POINT ( 'NONE',  ( 1.315538599303259781, -19.97434797600633871, 19.03762469184452755 ) ) ;
#16910=EDGE_LOOP ( 'NONE', ( #7803, #11673 ) ) ;
#16912=DIRECTION ( 'NONE',  ( -0.9898214418809327952, -0.1423148382732853101, 0.000000000000000000 ) ) ;
#16913=CARTESIAN_POINT ( 'NONE',  ( 12.35522127307955209, 11.74279147895035891, 18.34798005862662507 ) ) ;
#16917=CARTESIAN_POINT ( 'NONE',  ( -17.61017686385352121, -9.517781650307568952, 6.892848776733236704 ) ) ;
#16918=CARTESIAN_POINT ( 'NONE',  ( -6.157909564977939176, 15.91569265719595982, 5.872146474157316831 ) ) ;
#16919=CARTESIAN_POINT ( 'NONE',  ( -19.94474618696874302, 1.485631111656370518, 6.788986777570692688 ) ) ;
#16921=CARTESIAN_POINT ( 'NONE',  ( -15.45998620766333076, -7.136073936211796642, 18.63641924841378028 ) ) ;
#16922=CYLINDRICAL_SURFACE ( 'NONE', #1652, 0.7500000000000006661 ) ;
#16926=CARTESIAN_POINT ( 'NONE',  ( -5.124412594240626895, 19.33243322302222111, 19.85261563089510872 ) ) ;
#16927=CARTESIAN_POINT ( 'NONE',  ( -15.28186893989758488, 12.93018916568089338, 7.652108011868850035 ) ) ;
#16928=CARTESIAN_POINT ( 'NONE',  ( 11.10715495309693424, -16.63223102436629475, 20.34789198813115263 ) ) ;
#16931=CIRCLE ( 'NONE', #20904, 9.482273699623480212 ) ;
#16932=CARTESIAN_POINT ( 'NONE',  ( 18.32239734440381440, -8.062462575157598010, 18.34969686940296185 ) ) ;
#16933=FACE_OUTER_BOUND ( 'NONE', #15569, .T. ) ;
#16934=ORIENTED_EDGE ( 'NONE', *, *, #3258, .T. ) ;
#16935=CARTESIAN_POINT ( 'NONE',  ( 4.476939094886639658, 16.43504713094787206, 20.25336174263950184 ) ) ;
#16937=VECTOR ( 'NONE', #6339, 1000.000000000000000 ) ;
#16938=CARTESIAN_POINT ( 'NONE',  ( -7.850819104082916056, -15.15878979529809811, 18.73314399819311760 ) ) ;
#16940=EDGE_LOOP ( 'NONE', ( #30206, #8198, #23845, #27297 ) ) ;
#16941=DIRECTION ( 'NONE',  ( 0.000000000000000000, 0.000000000000000000, -1.000000000000000000 ) ) ;
#16944=ORIENTED_EDGE ( 'NONE', *, *, #4936, .T. ) ;
#16946=CARTESIAN_POINT ( 'NONE',  ( 14.87898868866547097, 13.36471831362574747, 5.652196082369964181 ) ) ;
#16947=LINE ( 'NONE', #23802, #13301 ) ;
#16948=CIRCLE ( 'NONE', #27917, 1.000000000000011324 ) ;
#16949=DIRECTION ( 'NONE',  ( -0.000000000000000000, -0.000000000000000000, 1.000000000000000000 ) ) ;
#16957=EDGE_LOOP ( 'NONE', ( #24087, #30814, #12528, #9796 ) ) ;
#16959=DIRECTION ( 'NONE',  ( 1.000000000000000000, 0.000000000000000000, 0.000000000000000000 ) ) ;
#16960=ORIENTED_EDGE ( 'NONE', *, *, #21146, .T. ) ;
#16964=EDGE_LOOP ( 'NONE', ( #3780, #25379, #19611, #10869 ) ) ;
#16966=CARTESIAN_POINT ( 'NONE',  ( 15.98815986143406143, -5.948957736846852029, 18.44527579819791185 ) ) ;
#16976=CARTESIAN_POINT ( 'NONE',  ( -12.71685080539083934, 11.31419172277363927, 19.22654678686458141 ) ) ;
#16977=CARTESIAN_POINT ( 'NONE',  ( -9.661386603328292466, -17.53179420831166269, 19.14333282897057842 ) ) ;
#16982=CARTESIAN_POINT ( 'NONE',  ( 9.085188746210626221, -14.39608436040016315, 7.080843742048788414 ) ) ;
#16985=CARTESIAN_POINT ( 'NONE',  ( 4.049916830765387665, 16.55712665160098851, 20.34789198813115263 ) ) ;
#16986=ORIENTED_EDGE ( 'NONE', *, *, #9470, .F. ) ;
#16989=ADVANCED_FACE ( 'NONE', ( #15428 ), #8271, .F. ) ;
#16991=ADVANCED_FACE ( 'NONE', ( #3435 ), #17601, .T. ) ;
#16992=CARTESIAN_POINT ( 'NONE',  ( -5.020628478053031252, 16.27454347535058332, 7.500898271101006820 ) ) ;
#16993=CARTESIAN_POINT ( 'NONE',  ( -15.49717968184286931, -7.050617358874958107, 6.031926333436657295 ) ) ;
#16999=DIRECTION ( 'NONE',  ( 0.000000000000000000, 0.000000000000000000, 1.000000000000000000 ) ) ;
#17001=CARTESIAN_POINT ( 'NONE',  ( -4.163336342344337027E-14, 1.387778780781445676E-14, 21.50000000000000000 ) ) ;
#17002=ADVANCED_FACE ( 'NONE', ( #25842 ), #4620, .F. ) ;
#17004=CARTESIAN_POINT ( 'NONE',  ( 12.43449883826693103, 11.65450130491726632, 7.652108011868850035 ) ) ;
#17006=EDGE_CURVE ( 'NONE', #25672, #27411, #14269, .T. ) ;
#17007=CARTESIAN_POINT ( 'NONE',  ( 18.41033144393026078, -7.859752488074923882, 7.643931100913408550 ) ) ;
#17009=CARTESIAN_POINT ( 'NONE',  ( 16.74250988114177474, 3.198928528055117404, 18.34798005863078885 ) ) ;
#17010=VECTOR ( 'NONE', #20371, 1000.000000000000000 ) ;
#17011=LINE ( 'NONE', #29340, #9552 ) ;
#17013=EDGE_CURVE ( 'NONE', #160, #16773, #7118, .T. ) ;
#17014=DIRECTION ( 'NONE',  ( 1.000000000000000000, 0.000000000000000000, 0.000000000000000000 ) ) ;
#17018=CYLINDRICAL_SURFACE ( 'NONE', #10405, 0.7500000000000024425 ) ;
#17031=CARTESIAN_POINT ( 'NONE',  ( -14.67633008511251802, 13.58695459845238318, 19.47728749465736797 ) ) ;
#17032=CARTESIAN_POINT ( 'NONE',  ( 4.819993392629171147, 16.32915940664440058, 6.031926333436655518 ) ) ;
#17039=ORIENTED_EDGE ( 'NONE', *, *, #5164, .T. ) ;
#17040=CARTESIAN_POINT ( 'NONE',  ( -1.000000000000008438, 19.97498435543819539, 24.50000000000000000 ) ) ;
#17043=DIRECTION ( 'NONE',  ( 1.000000000000000000, 0.000000000000000000, 0.000000000000000000 ) ) ;
#17046=CARTESIAN_POINT ( 'NONE',  ( -9.748913725731204849, -17.46314199939011402, 6.149077423860693337 ) ) ;
#17049=CARTESIAN_POINT ( 'NONE',  ( 0.7788148826605763020, -17.02744010918315709, 20.34789198813115263 ) ) ;
#17054=VERTEX_POINT ( 'NONE', #24410 ) ;
#17057=CARTESIAN_POINT ( 'NONE',  ( 12.12755608862868328, 11.99246096336392320, 18.39992786714538298 ) ) ;
#17062=CIRCLE ( 'NONE', #21032, 0.7499999999999997780 ) ;
#17065=CARTESIAN_POINT ( 'NONE',  ( -6.123826420728666342, 19.05819691457235621, 5.661398277488801867 ) ) ;
#17066=VECTOR ( 'NONE', #18621, 1000.000000000000114 ) ;
#17068=CARTESIAN_POINT ( 'NONE',  ( 0.000000000000000000, 0.000000000000000000, 1.500000000000001332 ) ) ;
#17071=CARTESIAN_POINT ( 'NONE',  ( -18.05883950494727230, -8.636531109380523930, 18.34798005862930381 ) ) ;
#17072=DIRECTION ( 'NONE',  ( -0.000000000000000000, -0.000000000000000000, 1.000000000000000000 ) ) ;
#17075=CARTESIAN_POINT ( 'NONE',  ( 9.131494062835612269, 2.555255504830998170, 1.500000000000001332 ) ) ;
#17077=CARTESIAN_POINT ( 'NONE',  ( -12.71124774491287823, 11.32026698792773800, 6.755862304746362845 ) ) ;
#17078=CARTESIAN_POINT ( 'NONE',  ( -0.1008988851204854764, -17.02363397670944067, 6.143977687428010093 ) ) ;
#17084=CARTESIAN_POINT ( 'NONE',  ( 5.021901920966173272, 16.26348455184632513, 19.33715507985239412 ) ) ;
#17086=CARTESIAN_POINT ( 'NONE',  ( -13.38160118231794371, 10.55829203257429860, 18.34798005863078885 ) ) ;
#17088=VERTEX_POINT ( 'NONE', #7739 ) ;
#17091=VECTOR ( 'NONE', #16308, 1000.000000000000227 ) ;
#17094=ORIENTED_EDGE ( 'NONE', *, *, #19009, .T. ) ;
#17095=CARTESIAN_POINT ( 'NONE',  ( -18.43314756787626507, -7.806103702558631063, 6.211014596808754007 ) ) ;
#17099=CARTESIAN_POINT ( 'NONE',  ( 0.2775250113394570617, -20.01590685155468918, 5.653912893140659257 ) ) ;
#17100=EDGE_CURVE ( 'NONE', #25215, #29085, #1291, .T. ) ;
#17101=CARTESIAN_POINT ( 'NONE',  ( -16.96556290498877573, 1.647560670993253540, 5.652196082368482699 ) ) ;
#17108=CARTESIAN_POINT ( 'NONE',  ( 4.333676792162783009, 19.52490442444424801, 6.392525840300347539 ) ) ;
#17110=EDGE_LOOP ( 'NONE', ( #3684, #19569, #8193, #6775 ) ) ;
#17116=CARTESIAN_POINT ( 'NONE',  ( 14.89413762494257476, 13.37445394317134273, 18.34798005862930736 ) ) ;
#17117=CARTESIAN_POINT ( 'NONE',  ( -10.98804681698542751, -16.73276138505788779, 7.500898271101006820 ) ) ;
#17118=ORIENTED_EDGE ( 'NONE', *, *, #7062, .F. ) ;
#17123=CARTESIAN_POINT ( 'NONE',  ( 15.70758541206063796, -6.601999697741291584, 18.37259980046034613 ) ) ;
#17125=VERTEX_POINT ( 'NONE', #26767 ) ;
#17129=CARTESIAN_POINT ( 'NONE',  ( -6.300265418930215411, 19.00075578015506039, 18.39992786714538298 ) ) ;
#17130=CARTESIAN_POINT ( 'NONE',  ( -14.72004833196315410, 13.56602982695842208, 19.66989035740801839 ) ) ;
#17138=CARTESIAN_POINT ( 'NONE',  ( -19.87079772360653251, 2.422354609568012851, 5.652605728828373977 ) ) ;
#17140=CARTESIAN_POINT ( 'NONE',  ( -17.75446986341067301, 9.207540381081360081, 24.50000000000000000 ) ) ;
#17144=CARTESIAN_POINT ( 'NONE',  ( 10.36464550818151586, -17.10487384371580788, 6.144783687052520094 ) ) ;
#17147=FACE_BOUND ( 'NONE', #13969, .T. ) ;
#17148=DIRECTION ( 'NONE',  ( 0.000000000000000000, 0.000000000000000000, -1.000000000000000000 ) ) ;
#17150=AXIS2_PLACEMENT_3D ( 'NONE', #22135, #12642, #933 ) ;
#17152=ORIENTED_EDGE ( 'NONE', *, *, #19872, .T. ) ;
#17157=CARTESIAN_POINT ( 'NONE',  ( 15.52282850165806138, 12.63957212366657501, 6.974106381145714018 ) ) ;
#17159=CYLINDRICAL_SURFACE ( 'NONE', #9951, 20.00000000000000000 ) ;
#17161=DIRECTION ( 'NONE',  ( 0.6548607339452890974, 0.7557495743542548272, 0.000000000000000000 ) ) ;
#17163=EDGE_CURVE ( 'NONE', #7591, #8705, #3281, .T. ) ;
#17165=EDGE_CURVE ( 'NONE', #13536, #12805, #3785, .T. ) ;
#17169=AXIS2_PLACEMENT_3D ( 'NONE', #17904, #25210, #13072 ) ;
#17171=CARTESIAN_POINT ( 'NONE',  ( 10.50588106577561653, -17.03964880432502937, 20.05479082170252525 ) ) ;
#17176=CARTESIAN_POINT ( 'NONE',  ( -5.130938270761554065, 7.974144905643839820, 21.50000000000000000 ) ) ;
#17178=CARTESIAN_POINT ( 'NONE',  ( -8.884323311075783991, -1.438332125858144295, 21.50000000000000000 ) ) ;
#17179=EDGE_LOOP ( 'NONE', ( #8052, #7547, #4524, #23211 ) ) ;
#17184=CARTESIAN_POINT ( 'NONE',  ( 4.045242219987652987, 16.55840560649981441, 5.652196082368482699 ) ) ;
#17191=ORIENTED_EDGE ( 'NONE', *, *, #4245, .T. ) ;
#17194=DIRECTION ( 'NONE',  ( 0.000000000000000000, 0.000000000000000000, 1.000000000000000000 ) ) ;
#17195=ORIENTED_EDGE ( 'NONE', *, *, #18153, .T. ) ;
#17196=AXIS2_PLACEMENT_3D ( 'NONE', #2657, #21674, #21989 ) ;
#17199=ORIENTED_EDGE ( 'NONE', *, *, #20814, .F. ) ;
#17200=ORIENTED_EDGE ( 'NONE', *, *, #9944, .F. ) ;
#17202=EDGE_CURVE ( 'NONE', #28757, #29885, #23894, .T. ) ;
#17205=DIRECTION ( 'NONE',  ( 0.000000000000000000, 0.000000000000000000, -1.000000000000000000 ) ) ;
#17206=DIRECTION ( 'NONE',  ( 0.000000000000000000, 0.000000000000000000, 1.000000000000000000 ) ) ;
#17207=CARTESIAN_POINT ( 'NONE',  ( -11.82521593960875528, 5.400395169024524655, 24.50000000000000000 ) ) ;
#17213=CARTESIAN_POINT ( 'NONE',  ( 0.8978415369256436129, -19.99755156235222486, 5.810767894563978686 ) ) ;
#17214=FACE_OUTER_BOUND ( 'NONE', #3198, .T. ) ;
#17216=EDGE_CURVE ( 'NONE', #19423, #29398, #21230, .T. ) ;
#17218=CARTESIAN_POINT ( 'NONE',  ( -14.74412167020460984, -8.612351851578502249, 6.233981582756856987 ) ) ;
#17219=PLANE ( 'NONE',  #1399 ) ;
#17221=CARTESIAN_POINT ( 'NONE',  ( -19.92877566111875254, 1.688993080932622348, 6.037995405461178855 ) ) ;
#17222=EDGE_CURVE ( 'NONE', #13104, #30552, #21698, .T. ) ;
#17223=CARTESIAN_POINT ( 'NONE',  ( -15.30652580117162209, -7.480423316612002438, 18.39701043959520987 ) ) ;
#17224=AXIS2_PLACEMENT_3D ( 'NONE', #28202, #14014, #18857 ) ;
#17226=VERTEX_POINT ( 'NONE', #9550 ) ;
#17229=CARTESIAN_POINT ( 'NONE',  ( -5.378544123449399805, 19.26344156360739746, 20.14992337338002315 ) ) ;
#17232=VERTEX_POINT ( 'NONE', #19377 ) ;
#17234=CARTESIAN_POINT ( 'NONE',  ( 15.76815964721466479, -6.465453726329343453, 18.35377592296120497 ) ) ;
#17237=ADVANCED_FACE ( 'NONE', ( #339 ), #12051, .F. ) ;
#17238=ORIENTED_EDGE ( 'NONE', *, *, #23124, .T. ) ;
#17239=LINE ( 'NONE', #10681, #8327 ) ;
#17242=CARTESIAN_POINT ( 'NONE',  ( -7.786278744154469855, -15.19480685132476161, 19.85459532544248162 ) ) ;
#17245=B_SPLINE_CURVE_WITH_KNOTS ( 'NONE', 3,
 ( #2223, #9414, #9099, #8959, #18930, #8790, #20640, #18318, #28436, #27834, #26086, #6463, #4115, #4257, #18618, #6753, #28586, #16889 ),
 .UNSPECIFIED., .F., .F.,
 ( 4, 2, 2, 2, 2, 2, 2, 2, 4 ),
 ( 0.003174295595554302643, 0.003570702171545536274, 0.003967108747536769904, 0.004363515323528003101, 0.004759921899519237165, 0.005156328475510471229, 0.005552735051501704426, 0.005949141627492937623, 0.006345548203484171687 ),
 .UNSPECIFIED. ) ;
#17248=AXIS2_PLACEMENT_3D ( 'NONE', #17251, #24569, #22233 ) ;
#17251=CARTESIAN_POINT ( 'NONE',  ( 0.4269445148198864892, 2.969464325642835689, 24.50000000000000000 ) ) ;
#17252=ORIENTED_EDGE ( 'NONE', *, *, #28622, .T. ) ;
#17253=CARTESIAN_POINT ( 'NONE',  ( -15.19605639364643324, -7.717080560943921697, 5.653912893140659257 ) ) ;
#17254=CARTESIAN_POINT ( 'NONE',  ( 14.18307372309186576, 14.10107868313151691, 6.523620417364438318 ) ) ;
#17255=CARTESIAN_POINT ( 'NONE',  ( -0.1272161363927056532, -17.02285684280287725, 6.211014596808754007 ) ) ;
#17256=DIRECTION ( 'NONE',  ( 1.000000000000000000, 0.000000000000000000, 0.000000000000000000 ) ) ;
#17257=DIRECTION ( 'NONE',  ( 0.9898214418809327952, 0.1423148382732852546, 0.000000000000000000 ) ) ;
#17258=CYLINDRICAL_SURFACE ( 'NONE', #19981, 20.00000000000000000 ) ;
#17259=CIRCLE ( 'NONE', #3819, 0.7500000000000006661 ) ;
#17261=VERTEX_POINT ( 'NONE', #4714 ) ;
#17265=VERTEX_POINT ( 'NONE', #14685 ) ;
#17268=DIRECTION ( 'NONE',  ( -0.000000000000000000, -0.000000000000000000, 1.000000000000000000 ) ) ;
#17272=CARTESIAN_POINT ( 'NONE',  ( 15.11794152162359595, 13.12142272612526206, 18.39701043959520987 ) ) ;
#17273=CARTESIAN_POINT ( 'NONE',  ( -8.832446728800205094, -14.56826516372322544, 5.701226463332907279 ) ) ;
#17274=VERTEX_POINT ( 'NONE', #9244 ) ;
#17275=CARTESIAN_POINT ( 'NONE',  ( -19.72513283648485327, 3.411576116177899465, 7.080843742048788414 ) ) ;
#17280=EDGE_CURVE ( 'NONE', #27809, #17660, #25186, .T. ) ;
#17281=CARTESIAN_POINT ( 'NONE',  ( 15.38599937579231636, -7.279790735017073189, 19.41069149716887310 ) ) ;
#17285=AXIS2_PLACEMENT_3D ( 'NONE', #27854, #29891, #30336 ) ;
#17287=CARTESIAN_POINT ( 'NONE',  ( -6.307863225249116468, 15.86248630188382513, 18.73743063545763121 ) ) ;
#17288=CARTESIAN_POINT ( 'NONE',  ( -15.35487586320816078, 12.84287697592353084, 20.34789198813115263 ) ) ;
#17289=VECTOR ( 'NONE', #29156, 1000.000000000000114 ) ;
#17290=CARTESIAN_POINT ( 'NONE',  ( -10.52279982399694092, -17.02885636288122839, 18.34798005862662507 ) ) ;
#17293=CARTESIAN_POINT ( 'NONE',  ( -6.630478080506957639, -6.778663211761441154, 21.50000000000000000 ) ) ;
#17295=CARTESIAN_POINT ( 'NONE',  ( 10.30772981839320934, -17.16011447240169474, 6.310736198168394928 ) ) ;
#17296=B_SPLINE_CURVE_WITH_KNOTS ( 'NONE', 3,
 ( #1373, #1066, #8088, #27263, #3238, #10888, #10575, #6046, #20398, #22263, #1223, #18059, #29755, #22106, #5895, #12761, #10723, #8234, #27576, #17739 ),
 .UNSPECIFIED., .F., .F.,
 ( 4, 2, 2, 2, 2, 2, 2, 2, 2, 4 ),
 ( 0.000000000000000000, 0.06250000000000179023, 0.1250000000000035805, 0.1875000000000053846, 0.2187500000000055234, 0.2500000000000056621, 0.3125000000000042744, 0.3750000000000029421, 0.4375000000000015543, 0.5000000000000001110 ),
 .UNSPECIFIED. ) ;
#17299=CARTESIAN_POINT ( 'NONE',  ( 10.47960520055065992, -7.757439966934453146, 24.50000000000000000 ) ) ;
#17303=CARTESIAN_POINT ( 'NONE',  ( 10.42711161940499309, -17.06705191410859612, 7.267242832833948007 ) ) ;
#17305=DIRECTION ( 'NONE',  ( -0.000000000000000000, -0.000000000000000000, 1.000000000000000000 ) ) ;
#17308=CYLINDRICAL_SURFACE ( 'NONE', #19139, 20.00000000000000000 ) ;
#17313=CARTESIAN_POINT ( 'NONE',  ( 0.4831130459764271801, -19.99459506363783490, 7.652108011868850923 ) ) ;
#17314=CARTESIAN_POINT ( 'NONE',  ( -17.76524000349413157, -9.187221810585024073, 18.54958172136248251 ) ) ;
#17315=CARTESIAN_POINT ( 'NONE',  ( 16.75466217413942971, 3.123260753354264452, 5.653912893140659257 ) ) ;
#17317=CARTESIAN_POINT ( 'NONE',  ( 12.87427757126086547, 11.14157019477621269, 6.018569869498933578 ) ) ;
#17318=ORIENTED_EDGE ( 'NONE', *, *, #15278, .F. ) ;
#17324=AXIS2_PLACEMENT_3D ( 'NONE', #19917, #17422, #17257 ) ;
#17327=CARTESIAN_POINT ( 'NONE',  ( -7.869584159753960861, 10.39565510934976977, 1.500000000000001332 ) ) ;
#17331=AXIS2_PLACEMENT_3D ( 'NONE', #13510, #13662, #1792 ) ;
#17333=CARTESIAN_POINT ( 'NONE',  ( 9.579384792474774812, -14.08793303971872390, 20.29090034784956131 ) ) ;
#17334=CYLINDRICAL_SURFACE ( 'NONE', #19841, 0.7500000000000006661 ) ;
#17337=CARTESIAN_POINT ( 'NONE',  ( -15.63429437150529822, 12.50148542865849244, 20.25542030744407640 ) ) ;
#17338=DIRECTION ( 'NONE',  ( 1.000000000000000000, 0.000000000000000000, 0.000000000000000000 ) ) ;
#17349=CARTESIAN_POINT ( 'NONE',  ( 16.86471733739763934, 2.322843836264933515, 6.143977687428010093 ) ) ;
#17358=ORIENTED_EDGE ( 'NONE', *, *, #22155, .F. ) ;
#17360=CARTESIAN_POINT ( 'NONE',  ( -4.163336342344337027E-14, 1.387778780781445676E-14, 24.50000000000000000 ) ) ;
#17362=VERTEX_POINT ( 'NONE', #18764 ) ;
#17372=AXIS2_PLACEMENT_3D ( 'NONE', #15891, #25404, #23644 ) ;
#17374=EDGE_CURVE ( 'NONE', #21024, #2038, #16563, .T. ) ;
#17375=DIRECTION ( 'NONE',  ( -0.000000000000000000, -0.000000000000000000, 1.000000000000000000 ) ) ;
#17382=FACE_OUTER_BOUND ( 'NONE', #26679, .T. ) ;
#17383=CARTESIAN_POINT ( 'NONE',  ( 9.928183626064983613, -13.85837025666176991, 5.652605728828375753 ) ) ;
#17384=CARTESIAN_POINT ( 'NONE',  ( -15.42813811594281681, -7.209250886987517148, 18.55820869691756769 ) ) ;
#17385=AXIS2_PLACEMENT_3D ( 'NONE', #5033, #343, #11912 ) ;
#17389=CARTESIAN_POINT ( 'NONE',  ( 9.248129367672067502, 2.094186647214772101, 1.500000000000001332 ) ) ;
#17403=CARTESIAN_POINT ( 'NONE',  ( 5.908622583341373691, 19.12614776545568418, 18.55820869691756769 ) ) ;
#17405=DIRECTION ( 'NONE',  ( 1.000000000000000000, 0.000000000000000000, 0.000000000000000000 ) ) ;
#17407=CARTESIAN_POINT ( 'NONE',  ( -7.852931495992875988, -15.15760027748588179, 19.96568007040468373 ) ) ;
#17410=ADVANCED_FACE ( 'NONE', ( #20145 ), #15146, .F. ) ;
#17411=CARTESIAN_POINT ( 'NONE',  ( -9.056208293496290196, 2.810445847081948667, 13.00000000000000178 ) ) ;
#17417=LINE ( 'NONE', #12900, #8833 ) ;
#17419=B_SPLINE_SURFACE_WITH_KNOTS ( 'NONE', 3, 1, ( 
 ( #5217, #12400 ),
 ( #19559, #29079 ),
 ( #27515, #5835 ),
 ( #8337, #1305 ),
 ( #15335, #24865 ),
 ( #3648, #3502 ),
 ( #24692, #22203 ),
 ( #1148, #8505 ),
 ( #26902, #17851 ),
 ( #25010, #3187 ),
 ( #5522, #19875 ),
 ( #22366, #12868 ),
 ( #29392, #27050 ),
 ( #15173, #10661 ),
 ( #27369, #15492 ),
 ( #20019, #15025 ),
 ( #29539, #24539 ),
 ( #15644, #17531 ),
 ( #3336, #1003 ),
 ( #13163, #22656 ),
 ( #10825, #29863 ),
 ( #17682, #18007 ),
 ( #6135, #25156 ),
 ( #3800, #13324 ),
 ( #18519, #13077 ),
 ( #30210, #25220 ),
 ( #1672, #15702 ),
 ( #1370, #13228 ),
 ( #15393, #29916 ),
 ( #8554, #3555 ),
 ( #16016, #8698 ) ),
 .UNSPECIFIED., .F., .F., .F.,
 ( 4, 3, 3, 3, 3, 3, 3, 3, 3, 3, 4 ),
 ( 2, 2 ),
 ( 0.000000000000000000, 0.05425176834609614362, 0.1085332949128348518, 0.1623767749169379715, 0.2157504826133058717, 0.2688657508888169789, 0.3218907763505471364, 0.3749548578363334772, 0.4282048033836237666, 0.4818374082110496448, 0.4999999999131651274 ),
 ( 0.000000000000000000, 1.000000000000000000 ),
 .UNSPECIFIED. ) ;
#17422=DIRECTION ( 'NONE',  ( 0.1423148382732852546, -0.9898214418809327952, 0.000000000000000000 ) ) ;
#17423=DIRECTION ( 'NONE',  ( -1.000000000000000000, 0.000000000000000000, 0.000000000000000000 ) ) ;
#17429=DIRECTION ( 'NONE',  ( -0.000000000000000000, 0.000000000000000000, -1.000000000000000000 ) ) ;
#17439=CARTESIAN_POINT ( 'NONE',  ( -9.248129367672079937, -2.094186647214709485, 1.500000000000001332 ) ) ;
#17440=ORIENTED_EDGE ( 'NONE', *, *, #12471, .F. ) ;
#17441=CARTESIAN_POINT ( 'NONE',  ( -19.71348387055304130, 3.477795851889708523, 6.864725433338323413 ) ) ;
#17442=CARTESIAN_POINT ( 'NONE',  ( 17.90972305382299368, -8.901787470106556910, 6.781503518395063601 ) ) ;
#17445=CARTESIAN_POINT ( 'NONE',  ( 12.24063095261064404, 4.490763173670002217, 1.500000000000001332 ) ) ;
#17450=CARTESIAN_POINT ( 'NONE',  ( -5.971396161871752817, 19.08775596758252036, 20.34789198813115263 ) ) ;
#17452=CARTESIAN_POINT ( 'NONE',  ( 19.63374410927882607, 3.902325345048613947, 7.366751648393900176 ) ) ;
#17454=VECTOR ( 'NONE', #22018, 1000.000000000000114 ) ;
#17459=EDGE_CURVE ( 'NONE', #12805, #12720, #12236, .T. ) ;
#17460=CARTESIAN_POINT ( 'NONE',  ( 10.27954044202352968, -17.17695407163359889, 6.420335371522007506 ) ) ;
#17466=ORIENTED_EDGE ( 'NONE', *, *, #26931, .T. ) ;
#17467=CARTESIAN_POINT ( 'NONE',  ( 17.90987090234840906, -8.901490003858832267, 19.21471108562413832 ) ) ;
#17469=CARTESIAN_POINT ( 'NONE',  ( 12.72536390617885438, -2.839914339433650348, 24.50000000000000000 ) ) ;
#17471=CARTESIAN_POINT ( 'NONE',  ( -4.163336342344337027E-14, 1.387778780781445676E-14, 1.500000000000000000 ) ) ;
#17474=CARTESIAN_POINT ( 'NONE',  ( 5.780652116621846304, 19.14677724775280154, 5.775318986477950389 ) ) ;
#17476=CARTESIAN_POINT ( 'NONE',  ( -10.40347366321433142, -17.08171436691437606, 20.34789198813115263 ) ) ;
#17477=CARTESIAN_POINT ( 'NONE',  ( 14.23411040819766882, 14.07463391211592096, 6.341840715582230281 ) ) ;
#17478=CARTESIAN_POINT ( 'NONE',  ( 16.74328840634222715, 3.194145055459935101, 7.652108011868850035 ) ) ;
#17479=ORIENTED_EDGE ( 'NONE', *, *, #25619, .T. ) ;
#17481=VERTEX_POINT ( 'NONE', #970 ) ;
#17489=CARTESIAN_POINT ( 'NONE',  ( 0.000000000000000000, 0.000000000000000000, 1.500000000000001332 ) ) ;
#17493=CARTESIAN_POINT ( 'NONE',  ( 9.048061653868892051, -14.41834352799975427, 19.66989035740801839 ) ) ;
#17494=CARTESIAN_POINT ( 'NONE',  ( 10.25423333689187544, -17.17121715837755147, 19.21471108562414898 ) ) ;
#17497=EDGE_CURVE ( 'NONE', #19042, #7607, #4790, .T. ) ;
#17498=CARTESIAN_POINT ( 'NONE',  ( -15.64089046717304399, 12.49323067438739621, 18.44527579819791185 ) ) ;
#17503=CARTESIAN_POINT ( 'NONE',  ( -5.352643706120520761, -7.827050521741861999, 21.50000000000000000 ) ) ;
#17508=CARTESIAN_POINT ( 'NONE',  ( 19.55517958221000185, 4.194633687229720742, 6.523620417364448976 ) ) ;
#17509=ORIENTED_EDGE ( 'NONE', *, *, #8836, .F. ) ;
#17515=EDGE_LOOP ( 'NONE', ( #28906, #26803, #29060, #30711 ) ) ;
#17516=CARTESIAN_POINT ( 'NONE',  ( -10.08096377525214926, -17.27393813307045178, 7.528076282304592581 ) ) ;
#17520=VECTOR ( 'NONE', #15889, 1000.000000000000000 ) ;
#17524=ADVANCED_FACE ( 'NONE', ( #500 ), #10020, .F. ) ;
#17525=CARTESIAN_POINT ( 'NONE',  ( -6.587096388939656322, -18.88412458026101604, 24.50000000000000000 ) ) ;
#17526=CARTESIAN_POINT ( 'NONE',  ( 3.896869771148438577, -16.82098518409776489, 1.500000000000000000 ) ) ;
#17527=CARTESIAN_POINT ( 'NONE',  ( 0.8597189258598705308, -17.02598424914432940, 5.652605728828374865 ) ) ;
#17529=ORIENTED_EDGE ( 'NONE', *, *, #23142, .T. ) ;
#17530=AXIS2_PLACEMENT_3D ( 'NONE', #26531, #10003, #7359 ) ;
#17531=CARTESIAN_POINT ( 'NONE',  ( -9.351023488831160080, -14.22394595406099427, 19.00652017443069752 ) ) ;
#17533=CARTESIAN_POINT ( 'NONE',  ( -6.460166075217649961, 15.80732207284230029, 6.341840715582230281 ) ) ;
#17535=CARTESIAN_POINT ( 'NONE',  ( 10.56600709331201671, -13.41035981659392462, 7.196036389296800451 ) ) ;
#17542=DIRECTION ( 'NONE',  ( -1.000000000000000000, 0.000000000000000000, 0.000000000000000000 ) ) ;
#17544=CARTESIAN_POINT ( 'NONE',  ( -0.2239719228550731966, -17.01994463034866101, 6.782064869129511564 ) ) ;
#17546=EDGE_LOOP ( 'NONE', ( #10458, #30163, #5177, #17199 ) ) ;
#17547=CARTESIAN_POINT ( 'NONE',  ( 16.01802636628489296, -5.877265577766301874, 18.45571264222804331 ) ) ;
#17551=CARTESIAN_POINT ( 'NONE',  ( 4.045241160018713700, 16.55840174602106529, 18.34798005862930026 ) ) ;
#17559=CARTESIAN_POINT ( 'NONE',  ( -19.80980381183504235, 2.754394816484158515, 18.37250658438899009 ) ) ;
#17560=VERTEX_POINT ( 'NONE', #29968 ) ;
#17561=CARTESIAN_POINT ( 'NONE',  ( -15.25992540518562635, -7.581593484474010047, 5.670038381137163519 ) ) ;
#17563=CARTESIAN_POINT ( 'NONE',  ( 12.93287820104972141, 11.07039438042774293, 19.85270094495842130 ) ) ;
#17565=CARTESIAN_POINT ( 'NONE',  ( 16.17629920997981330, -5.470921186997150798, 6.329955581934032516 ) ) ;
#17568=CARTESIAN_POINT ( 'NONE',  ( -17.06430796154857887, 0.6673913134784715817, 6.917457548096561659 ) ) ;
#17569=DIRECTION ( 'NONE',  ( -0.7557495743542581579, -0.6548607339452852116, 0.000000000000000000 ) ) ;
#17572=EDGE_LOOP ( 'NONE', ( #13040, #516, #22120, #9133 ) ) ;
#17573=ADVANCED_FACE ( 'NONE', ( #6413 ), #7896, .T. ) ;
#17576=VERTEX_POINT ( 'NONE', #7331 ) ;
#17581=DIRECTION ( 'NONE',  ( 1.000000000000000000, 0.000000000000000000, 0.000000000000000000 ) ) ;
#17584=CARTESIAN_POINT ( 'NONE',  ( 12.99901289864994958, 10.98932263627886385, 19.56050940960062690 ) ) ;
#17586=AXIS2_PLACEMENT_3D ( 'NONE', #678, #10046, #19555 ) ;
#17590=CARTESIAN_POINT ( 'NONE',  ( 5.881244434206234217, 6.812559277181991391, 1.500000000000001332 ) ) ;
#17591=CARTESIAN_POINT ( 'NONE',  ( 19.68627777834516479, 3.628879393376897244, 20.25542030744407640 ) ) ;
#17594=CYLINDRICAL_SURFACE ( 'NONE', #23797, 0.7500000000000011102 ) ;
#17599=EDGE_CURVE ( 'NONE', #8468, #8832, #12772, .T. ) ;
#17601=B_SPLINE_SURFACE_WITH_KNOTS ( 'NONE', 3, 1, ( 
 ( #10454, #22755 ),
 ( #20430, #19968 ),
 ( #17628, #15587 ),
 ( #27300, #5930 ),
 ( #6077, #29799 ),
 ( #29487, #13111 ),
 ( #26999, #12956 ),
 ( #3747, #29950 ),
 ( #8587, #6233 ),
 ( #24950, #1977 ),
 ( #1097, #11499 ),
 ( #29332, #7974 ),
 ( #17477, #17947 ),
 ( #29637, #1253 ),
 ( #10760, #27457 ),
 ( #16629, #16476 ),
 ( #18663, #28169 ),
 ( #12110, #95 ),
 ( #6800, #14121 ),
 ( #5084, #30815 ),
 ( #19272, #23789 ),
 ( #9756, #9613 ),
 ( #18822, #7263 ),
 ( #25992, #6965 ),
 ( #16324, #28790 ),
 ( #2592, #11961 ),
 ( #23946, #13984 ),
 ( #14595, #24100 ),
 ( #23625, #9296 ),
 ( #28638, #2748 ),
 ( #18978, #21609 ) ),
 .UNSPECIFIED., .F., .F., .F.,
 ( 4, 3, 3, 3, 3, 3, 3, 3, 3, 3, 4 ),
 ( 2, 2 ),
 ( 0.4999999998345681651, 0.5360336730431942698, 0.5907651151589017324, 0.6456034593241839481, 0.6998270958050443191, 0.7529536536315944995, 0.8052385063053264513, 0.8575343587103996246, 0.9106564858195047574, 0.9648414833209688624, 1.000000006602610014 ),
 ( 0.000000000000000000, 1.000000000000000000 ),
 .UNSPECIFIED. ) ;
#17605=CARTESIAN_POINT ( 'NONE',  ( 1.665992581745963985, -16.99218467486907258, 6.147510495896842286 ) ) ;
#17607=VECTOR ( 'NONE', #4648, 1000.000000000000000 ) ;
#17608=FACE_OUTER_BOUND ( 'NONE', #22799, .T. ) ;
#17609=DIRECTION ( 'NONE',  ( 1.000000000000000000, 0.000000000000000000, 0.000000000000000000 ) ) ;
#17611=AXIS2_PLACEMENT_3D ( 'NONE', #24002, #28703, #2651 ) ;
#17612=CARTESIAN_POINT ( 'NONE',  ( -19.86132161767506332, 2.497832813224998727, 5.652196082364320695 ) ) ;
#17618=CARTESIAN_POINT ( 'NONE',  ( 17.96625477203412657, -8.787278772463423593, 19.85261563089510517 ) ) ;
#17619=CARTESIAN_POINT ( 'NONE',  ( -5.971396161871752817, 19.08775596758251680, 7.652108011868850035 ) ) ;
#17621=CARTESIAN_POINT ( 'NONE',  ( -5.435829780283180312, 16.15227280059888315, 7.652108011868850035 ) ) ;
#17624=CARTESIAN_POINT ( 'NONE',  ( 5.422617586916723020, 19.25129646183500398, 7.652108011868850035 ) ) ;
#17626=AXIS2_PLACEMENT_3D ( 'NONE', #29537, #5831, #29074 ) ;
#17627=CARTESIAN_POINT ( 'NONE',  ( -10.51513057463694523, -17.01270198993485394, 20.34789198813115263 ) ) ;
#17628=CARTESIAN_POINT ( 'NONE',  ( 14.79201625507351636, 13.48748956535167487, 5.661398277488801867 ) ) ;
#17629=CARTESIAN_POINT ( 'NONE',  ( 19.89739966441223018, 2.193321724558644714, 6.755862304746362845 ) ) ;
#17630=ORIENTED_EDGE ( 'NONE', *, *, #17006, .F. ) ;
#17631=CARTESIAN_POINT ( 'NONE',  ( 6.812559277181973627, -5.881244434206257310, 1.500000000000001332 ) ) ;
#17632=ORIENTED_EDGE ( 'NONE', *, *, #19082, .F. ) ;
#17634=CARTESIAN_POINT ( 'NONE',  ( -13.55077504527628562, 10.35587614683493918, 18.34938820207544552 ) ) ;
#17635=AXIS2_PLACEMENT_3D ( 'NONE', #8188, #26916, #17694 ) ;
#17640=CARTESIAN_POINT ( 'NONE',  ( 5.231931633751616850, 19.32210152104737233, 7.652108011868850035 ) ) ;
#17645=CARTESIAN_POINT ( 'NONE',  ( 9.002475149809907151, -14.44561766934883273, 19.33715507985239412 ) ) ;
#17649=B_SPLINE_CURVE_WITH_KNOTS ( 'NONE', 3,
 ( #2252, #9447, #6488, #18803, #28323, #27864, #16150, #18503, #16604, #30636, #21115, #6636, #11624, #18962, #16305, #28472, #7098, #4143 ),
 .UNSPECIFIED., .F., .F.,
 ( 4, 2, 2, 2, 2, 2, 2, 2, 4 ),
 ( 0.003174295595554298306, 0.003570702171545536707, 0.003967108747536774241, 0.004363515323528012642, 0.004759921899519251043, 0.005156328475510488576, 0.005552735051501727845, 0.005949141627492967113, 0.006345548203484206382 ),
 .UNSPECIFIED. ) ;
#17656=CARTESIAN_POINT ( 'NONE',  ( -15.26094448139682846, 12.92753815214665636, 18.34726407865098707 ) ) ;
#17658=DIRECTION ( 'NONE',  ( -0.000000000000000000, -0.000000000000000000, 1.000000000000000000 ) ) ;
#17659=CARTESIAN_POINT ( 'NONE',  ( 16.81826667484149240, 2.692788315428430224, 7.526951045817047437 ) ) ;
#17660=VERTEX_POINT ( 'NONE', #6702 ) ;
#17662=CARTESIAN_POINT ( 'NONE',  ( -4.163336342344337027E-14, 1.387778780781445676E-14, 1.500000000000000000 ) ) ;
#17663=CYLINDRICAL_SURFACE ( 'NONE', #23912, 0.7500000000000006661 ) ;
#17664=VERTEX_POINT ( 'NONE', #144 ) ;
#17669=EDGE_LOOP ( 'NONE', ( #573, #5042, #27244, #25796 ) ) ;
#17672=DIRECTION ( 'NONE',  ( 0.1423148382732746797, -0.9898214418809342385, 0.000000000000000000 ) ) ;
#17676=CARTESIAN_POINT ( 'NONE',  ( -11.03614041005515567, -16.67970391259860108, 7.454139397117727661 ) ) ;
#17679=CARTESIAN_POINT ( 'NONE',  ( 0.5800982118606525795, -20.00934090639729135, 5.678370764302467677 ) ) ;
#17682=CARTESIAN_POINT ( 'NONE',  ( -11.12409513110480574, -16.64241105543193200, 18.63641924841378028 ) ) ;
#17686=DIRECTION ( 'NONE',  ( 1.000000000000000000, 0.000000000000000000, 0.000000000000000000 ) ) ;
#17689=ORIENTED_EDGE ( 'NONE', *, *, #16033, .T. ) ;
#17693=CARTESIAN_POINT ( 'NONE',  ( -13.23566211985188623, 10.73140863935235068, 5.670038381137163519 ) ) ;
#17694=DIRECTION ( 'NONE',  ( 0.2817325568414296710, -0.9594929736144973687, 0.000000000000000000 ) ) ;
#17695=ORIENTED_EDGE ( 'NONE', *, *, #19859, .F. ) ;
#17703=LINE ( 'NONE', #25033, #5892 ) ;
#17704=FACE_OUTER_BOUND ( 'NONE', #14835, .T. ) ;
#17706=ORIENTED_EDGE ( 'NONE', *, *, #30525, .F. ) ;
#17707=CARTESIAN_POINT ( 'NONE',  ( -15.17962487735951527, -7.751670534285734604, 5.651989602109218858 ) ) ;
#17714=CARTESIAN_POINT ( 'NONE',  ( 11.40980092660686118, 6.310027164379057751, 1.500000000000001332 ) ) ;
#17727=DIRECTION ( 'NONE',  ( -0.7557495743542581579, -0.6548607339452852116, 0.000000000000000000 ) ) ;
#17728=CARTESIAN_POINT ( 'NONE',  ( 12.40635649856745815, 11.68570839673119188, 18.34969686940296185 ) ) ;
#17732=ORIENTED_EDGE ( 'NONE', *, *, #25909, .F. ) ;
#17735=CARTESIAN_POINT ( 'NONE',  ( 6.631244434206235105, 6.812559277181991391, 1.500000000000001332 ) ) ;
#17739=CARTESIAN_POINT ( 'NONE',  ( -5.549075634136965363, 16.11684027513961226, 18.34798005863078885 ) ) ;
#17744=CARTESIAN_POINT ( 'NONE',  ( -16.94861615806142296, 1.782241101945937212, 20.34789198813115618 ) ) ;
#17745=AXIS2_PLACEMENT_3D ( 'NONE', #13997, #11806, #21000 ) ;
#17751=CARTESIAN_POINT ( 'NONE',  ( 16.55532831589958320, 4.193940174973930013, 6.672349528511551497 ) ) ;
#17754=CARTESIAN_POINT ( 'NONE',  ( -7.673856334772117371, -15.25703464229374084, 19.47783254395485031 ) ) ;
#17758=CARTESIAN_POINT ( 'NONE',  ( -16.96555893289282935, 1.647560171710575228, 18.34798005862662507 ) ) ;
#17759=LINE ( 'NONE', #27439, #7379 ) ;
#17762=CARTESIAN_POINT ( 'NONE',  ( 11.71757112412214141, -16.22992597261981018, 18.64703902303423178 ) ) ;
#17767=CARTESIAN_POINT ( 'NONE',  ( 18.00031268893096481, -8.717656915646676552, 18.72886616302734097 ) ) ;
#17768=CARTESIAN_POINT ( 'NONE',  ( 10.99809977392671279, -16.70505906359366932, 7.652108011868849147 ) ) ;
#17769=FACE_OUTER_BOUND ( 'NONE', #9822, .T. ) ;
#17770=ORIENTED_EDGE ( 'NONE', *, *, #20619, .T. ) ;
#17772=CARTESIAN_POINT ( 'NONE',  ( 0.000000000000000000, 0.000000000000000000, 21.50000000000000000 ) ) ;
#17775=AXIS2_PLACEMENT_3D ( 'NONE', #30068, #4320, #13849 ) ;
#17778=B_SPLINE_CURVE_WITH_KNOTS ( 'NONE', 3,
 ( #16457, #18648, #13672, #20253, #23156, #9128, #25971, #16149, #30344, #4456, #21114, #20962, #1805, #30486, #4287, #14099 ),
 .UNSPECIFIED., .F., .F.,
 ( 4, 2, 2, 2, 2, 2, 2, 4 ),
 ( 0.5000000000000000000, 0.6250000000000008882, 0.6875000000000015543, 0.7187500000000019984, 0.7500000000000023315, 0.8125000000000014433, 0.8750000000000006661, 1.000000000000000000 ),
 .UNSPECIFIED. ) ;
#17779=ORIENTED_EDGE ( 'NONE', *, *, #20077, .F. ) ;
#17782=CARTESIAN_POINT ( 'NONE',  ( 7.827050521741877098, -5.352643706120495004, 21.50000000000000000 ) ) ;
#17783=VECTOR ( 'NONE', #11715, 1000.000000000000000 ) ;
#17786=CARTESIAN_POINT ( 'NONE',  ( 19.87213478643044340, 2.412525337365569733, 6.018569869498933578 ) ) ;
#17789=CARTESIAN_POINT ( 'NONE',  ( -11.40980092660686829, 6.310027164379044429, 1.500000000000001332 ) ) ;
#17793=ADVANCED_FACE ( 'NONE', ( #1239 ), #27334, .T. ) ;
#17797=ORIENTED_EDGE ( 'NONE', *, *, #15441, .T. ) ;
#17798=ADVANCED_FACE ( 'NONE', ( #2145 ), #30672, .F. ) ;
#17800=CARTESIAN_POINT ( 'NONE',  ( 4.469338653509386639, 19.51245501789046344, 7.196036389296800451 ) ) ;
#17802=CARTESIAN_POINT ( 'NONE',  ( -3.668292057955944596, 8.743977807160110416, 21.50000000000000000 ) ) ;
#17805=CARTESIAN_POINT ( 'NONE',  ( 10.58525311124732049, -16.99040216561238026, 18.55820869691756769 ) ) ;
#17806=CARTESIAN_POINT ( 'NONE',  ( 19.89475757678375345, 2.217009531549523960, 19.56050940960062690 ) ) ;
#17808=CARTESIAN_POINT ( 'NONE',  ( -5.815855718377446415, -16.25752007041490188, 1.500000000000000000 ) ) ;
#17809=CARTESIAN_POINT ( 'NONE',  ( 18.26182835180409825, -8.199456719779957936, 5.670038381137163519 ) ) ;
#17811=CARTESIAN_POINT ( 'NONE',  ( -15.85879827683069010, 12.21494667905098019, 18.73743063545763121 ) ) ;
#17812=CARTESIAN_POINT ( 'NONE',  ( 9.169883732660084164, -9.268939115642975679, 1.500000000000001332 ) ) ;
#17819=CARTESIAN_POINT ( 'NONE',  ( -4.935065328765587012, 16.29835470421560828, 20.12545155307891065 ) ) ;
#17821=EDGE_CURVE ( 'NONE', #15390, #8511, #2633, .T. ) ;
#17822=DIRECTION ( 'NONE',  ( 0.000000000000000000, 0.000000000000000000, 1.000000000000000000 ) ) ;
#17832=VERTEX_POINT ( 'NONE', #15065 ) ;
#17833=ORIENTED_EDGE ( 'NONE', *, *, #9993, .T. ) ;
#17834=CARTESIAN_POINT ( 'NONE',  ( -19.75697076387333695, 3.109827004491390934, 7.454139397117727661 ) ) ;
#17838=CARTESIAN_POINT ( 'NONE',  ( 0.3541519782205858613, -20.01464289576667710, 18.34798005862930381 ) ) ;
#17842=DIRECTION ( 'NONE',  ( 1.000000000000000000, 0.000000000000000000, 0.000000000000000000 ) ) ;
#17843=CARTESIAN_POINT ( 'NONE',  ( 19.91398265452213323, -1.852915226174633778, 24.50000000000000000 ) ) ;
#17846=CARTESIAN_POINT ( 'NONE',  ( 0.8008512464130215225, -20.00192252186466746, 5.749491821935610147 ) ) ;
#17851=CARTESIAN_POINT ( 'NONE',  ( -9.223046300750477045, -14.31106556781055339, 19.96783386855779341 ) ) ;
#17852=CARTESIAN_POINT ( 'NONE',  ( -15.13309390500917573, -7.848982836665745921, 7.652108011868850035 ) ) ;
#17853=CARTESIAN_POINT ( 'NONE',  ( -5.549075634136967139, 16.11684027513961226, 5.652196082368482699 ) ) ;
#17854=CARTESIAN_POINT ( 'NONE',  ( 11.94600218753717513, -16.06231219995581583, 6.672349528511551497 ) ) ;
#17863=CARTESIAN_POINT ( 'NONE',  ( -14.88989150774294146, 13.37932992012220446, 5.940635272151477686 ) ) ;
#17868=CARTESIAN_POINT ( 'NONE',  ( -11.05774036494469925, -16.68675304545164195, 5.862424720655265098 ) ) ;
#17871=B_SPLINE_SURFACE_WITH_KNOTS ( 'NONE', 3, 1, ( 
 ( #10202, #13166 ),
 ( #29866, #17383 ),
 ( #22207, #25014 ),
 ( #20022, #27203 ),
 ( #685, #15028 ),
 ( #3652, #29234 ),
 ( #8508, #24869 ),
 ( #3036, #8180 ),
 ( #22507, #8030 ),
 ( #5525, #843 ),
 ( #3339, #13018 ),
 ( #22659, #27519 ),
 ( #10828, #1007 ),
 ( #1152, #24543 ),
 ( #8340, #20337 ),
 ( #17854, #10513 ),
 ( #3190, #26905 ),
 ( #12710, #22369 ),
 ( #18010, #14881 ),
 ( #10665, #27372 ),
 ( #10364, #17535 ),
 ( #5838, #15338 ),
 ( #5680, #5993 ),
 ( #15176, #24696 ),
 ( #12871, #29544 ),
 ( #20172, #1476 ),
 ( #15967, #13327 ),
 ( #2063, #8647 ),
 ( #3804, #30009 ),
 ( #20930, #9095 ),
 ( #11586, #18158 ) ),
 .UNSPECIFIED., .F., .F., .F.,
 ( 4, 3, 3, 3, 3, 3, 3, 3, 3, 3, 4 ),
 ( 2, 2 ),
 ( 0.4999999998345684982, 0.5360336730431942698, 0.5907651151589017324, 0.6456034593241839481, 0.6998270958050443191, 0.7529536536315944995, 0.8052385063053264513, 0.8575343587103996246, 0.9106564858195047574, 0.9648414833209688624, 1.000000006602610236 ),
 ( 0.000000000000000000, 1.000000000000000000 ),
 .UNSPECIFIED. ) ;
#17873=AXIS2_PLACEMENT_3D ( 'NONE', #23188, #18535, #28040 ) ;
#17875=CARTESIAN_POINT ( 'NONE',  ( 19.58271949849003946, 4.064458250759533264, 19.85730954408918336 ) ) ;
#17877=CARTESIAN_POINT ( 'NONE',  ( 11.83211694375102496, -16.12463123479446381, 7.161525567826885208 ) ) ;
#17878=DIRECTION ( 'NONE',  ( -0.000000000000000000, -1.000000000000000000, -0.000000000000000000 ) ) ;
#17883=CARTESIAN_POINT ( 'NONE',  ( 9.349584168494304848, 12.69858007495367680, -0.6213203435596476032 ) ) ;
#17886=DIRECTION ( 'NONE',  ( -0.000000000000000000, -0.000000000000000000, 1.000000000000000000 ) ) ;
#17887=CARTESIAN_POINT ( 'NONE',  ( -17.06238204535203096, 0.6919203014629479176, 6.329955581934033404 ) ) ;
#17899=DIRECTION ( 'NONE',  ( 0.000000000000000000, -0.000000000000000000, -1.000000000000000000 ) ) ;
#17904=CARTESIAN_POINT ( 'NONE',  ( -8.072557715923444732, 14.41080185948837311, 24.50000000000000000 ) ) ;
#17907=CARTESIAN_POINT ( 'NONE',  ( -19.86072707285307359, 2.502642989097794590, 7.652108011868850035 ) ) ;
#17910=CARTESIAN_POINT ( 'NONE',  ( 18.08053511453367790, -8.550039048713399481, 7.454139397117720556 ) ) ;
#17911=CARTESIAN_POINT ( 'NONE',  ( 15.05429537369195359, 13.16750578773770464, 5.676722608126683944 ) ) ;
#17913=ORIENTED_EDGE ( 'NONE', *, *, #18066, .T. ) ;
#17914=DIRECTION ( 'NONE',  ( -0.000000000000000000, -0.000000000000000000, 1.000000000000000000 ) ) ;
#17916=CARTESIAN_POINT ( 'NONE',  ( -16.87834697510463045, 2.265528671608726619, 20.14907003336613300 ) ) ;
#17920=CARTESIAN_POINT ( 'NONE',  ( 19.72311808385369858, 3.421819763545496773, 5.678370764302467677 ) ) ;
#17923=CARTESIAN_POINT ( 'NONE',  ( -8.361245565923715262, -14.86101098545372956, 20.32367522806703874 ) ) ;
#17926=CARTESIAN_POINT ( 'NONE',  ( -9.353104432029162751, -14.22246372587116348, 6.973843882838226094 ) ) ;
#17927=FACE_BOUND ( 'NONE', #12378, .T. ) ;
#17929=CARTESIAN_POINT ( 'NONE',  ( 2.703030265324084080, -12.75514121382991384, 24.50000000000000000 ) ) ;
#17931=CARTESIAN_POINT ( 'NONE',  ( 10.46384303394385817, -13.48464439008897209, 18.64703902303423178 ) ) ;
#17934=VERTEX_POINT ( 'NONE', #4950 ) ;
#17937=DIRECTION ( 'NONE',  ( -0.000000000000000000, -0.000000000000000000, 1.000000000000000000 ) ) ;
#17938=EDGE_CURVE ( 'NONE', #194, #2397, #9781, .T. ) ;
#17939=CARTESIAN_POINT ( 'NONE',  ( -5.023839636758347105, 19.37724795171757464, 6.420335371522007506 ) ) ;
#17940=EDGE_LOOP ( 'NONE', ( #10133, #17358, #6359, #22718 ) ) ;
#17941=CARTESIAN_POINT ( 'NONE',  ( 8.884323311075775109, 1.438332125858202692, 21.50000000000000000 ) ) ;
#17947=CARTESIAN_POINT ( 'NONE',  ( 11.69519594420021313, 12.44297266173655458, 6.341840715582230281 ) ) ;
#17948=CARTESIAN_POINT ( 'NONE',  ( 16.79398274391852652, 2.865066961627992903, 5.701226463332907279 ) ) ;
#17950=ADVANCED_FACE ( 'NONE', ( #12595 ), #5419, .F. ) ;
#17951=CARTESIAN_POINT ( 'NONE',  ( 12.35522127274689730, 11.74279147932066181, 5.652196082367002106 ) ) ;
#17952=ORIENTED_EDGE ( 'NONE', *, *, #29989, .F. ) ;
#17953=CARTESIAN_POINT ( 'NONE',  ( -14.01107592578418881, 9.765138712360661444, 19.47952243369110192 ) ) ;
#17954=VERTEX_POINT ( 'NONE', #7451 ) ;
#17956=LINE ( 'NONE', #13441, #3629 ) ;
#17957=DIRECTION ( 'NONE',  ( -0.9898214418809326842, 0.1423148382732851158, -0.000000000000000000 ) ) ;
#17965=CARTESIAN_POINT ( 'NONE',  ( -19.72513283648485682, 3.411576116177901241, 19.77662771831109367 ) ) ;
#17966=CARTESIAN_POINT ( 'NONE',  ( 18.30707599941031916, -8.097116190180054573, 5.657991946698900598 ) ) ;
#17968=CARTESIAN_POINT ( 'NONE',  ( -14.00200865723717314, 9.777219707070196719, 19.14333282897057842 ) ) ;
#17969=CARTESIAN_POINT ( 'NONE',  ( 4.782940318440150662, 19.43789448792816543, 20.19593175699879595 ) ) ;
#17973=EDGE_CURVE ( 'NONE', #19924, #11902, #28211, .T. ) ;
#17974=CARTESIAN_POINT ( 'NONE',  ( -5.976020107417634009, 19.08630880174946043, 5.652196082369965069 ) ) ;
#17975=ADVANCED_FACE ( 'NONE', ( #10406, #7600, #21786 ), #5569, .T. ) ;
#17976=CARTESIAN_POINT ( 'NONE',  ( -5.754904482333549787, 19.17304367822655209, 20.32842677360128292 ) ) ;
#17979=EDGE_CURVE ( 'NONE', #20736, #11391, #13298, .T. ) ;
#17980=DIRECTION ( 'NONE',  ( 0.000000000000000000, 0.000000000000000000, 1.000000000000000000 ) ) ;
#17981=CARTESIAN_POINT ( 'NONE',  ( 16.85582347139597914, 2.398957759888394214, 6.031926333436654630 ) ) ;
#17984=FACE_OUTER_BOUND ( 'NONE', #23179, .T. ) ;
#17987=ORIENTED_EDGE ( 'NONE', *, *, #18187, .T. ) ;
#17990=CARTESIAN_POINT ( 'NONE',  ( -19.77456323383487913, 2.996942905618070530, 5.775318986477955718 ) ) ;
#17992=VECTOR ( 'NONE', #26979, 1000.000000000000000 ) ;
#17993=DIRECTION ( 'NONE',  ( 1.000000000000000000, 0.000000000000000000, 0.000000000000000000 ) ) ;
#17995=CARTESIAN_POINT ( 'NONE',  ( -0.5282983270408738719, -19.99308596983832231, 6.144783687052519205 ) ) ;
#17999=CARTESIAN_POINT ( 'NONE',  ( -6.123826420728668118, 19.05819691457235976, 18.35718225375110180 ) ) ;
#18005=ORIENTED_EDGE ( 'NONE', *, *, #11521, .T. ) ;
#18007=CARTESIAN_POINT ( 'NONE',  ( -9.147715168420964105, -14.36154699054606887, 18.63641924841378028 ) ) ;
#18008=CARTESIAN_POINT ( 'NONE',  ( -15.06839649859471564, -7.981447355247934361, 7.627891251804737927 ) ) ;
#18009=CARTESIAN_POINT ( 'NONE',  ( -5.861334694664001255, 16.01657976118488236, 7.603368798681074736 ) ) ;
#18010=CARTESIAN_POINT ( 'NONE',  ( 11.89619695863782312, -16.09924856797056592, 6.995624166085161910 ) ) ;
#18012=VECTOR ( 'NONE', #15099, 1000.000000000000000 ) ;
#18017=CARTESIAN_POINT ( 'NONE',  ( -13.38159811102998198, 10.55828946469181417, 5.652196082367002106 ) ) ;
#18020=CARTESIAN_POINT ( 'NONE',  ( 0.000000000000000000, 0.000000000000000000, 1.500000000000001332 ) ) ;
#18022=CARTESIAN_POINT ( 'NONE',  ( -9.213835811784830909, -14.31736145455815645, 6.018569869498933578 ) ) ;
#18028=ADVANCED_FACE ( 'NONE', ( #3843 ), #24736, .F. ) ;
#18048=ORIENTED_EDGE ( 'NONE', *, *, #590, .F. ) ;
#18049=VECTOR ( 'NONE', #16482, 1000.000000000000000 ) ;
#18050=CARTESIAN_POINT ( 'NONE',  ( -6.385759811041538114, 15.83451745216639672, 18.84329447212442687 ) ) ;
#18053=ORIENTED_EDGE ( 'NONE', *, *, #29078, .F. ) ;
#18054=CARTESIAN_POINT ( 'NONE',  ( -16.86382086101523825, 2.355052171780695147, 5.940635272151477686 ) ) ;
#18056=CARTESIAN_POINT ( 'NONE',  ( 7.856594496258195726, 4.390207617113981442, 1.500000000000001332 ) ) ;
#18059=CARTESIAN_POINT ( 'NONE',  ( -4.574230723432976653, 16.39514892286269188, 19.21496526180054332 ) ) ;
#18063=FACE_OUTER_BOUND ( 'NONE', #9221, .T. ) ;
#18066=EDGE_CURVE ( 'NONE', #11919, #15501, #29225, .T. ) ;
#18068=CARTESIAN_POINT ( 'NONE',  ( -9.406652940105978189, 1.195154792889487227, 13.00000000000000178 ) ) ;
#18069=CARTESIAN_POINT ( 'NONE',  ( 19.74834695364560133, 3.274018421667482137, 5.652605728828373977 ) ) ;
#18071=CARTESIAN_POINT ( 'NONE',  ( 1.664698296075797890, -16.99226504953965389, 7.158811349119584833 ) ) ;
#18073=CARTESIAN_POINT ( 'NONE',  ( -8.770223337696748445, -14.60814232176959671, 5.676815824193227833 ) ) ;
#18076=CARTESIAN_POINT ( 'NONE',  ( 9.864935476092961508, -13.90063640548120460, 18.34798005862662507 ) ) ;
#18079=ORIENTED_EDGE ( 'NONE', *, *, #39, .F. ) ;
#18081=VECTOR ( 'NONE', #9254, 1000.000000000000000 ) ;
#18083=CARTESIAN_POINT ( 'NONE',  ( 11.11118388262826251, -16.62953976291647962, 5.652196082369964181 ) ) ;
#18085=CARTESIAN_POINT ( 'NONE',  ( -5.332709978455699051, 16.18357461815305243, 5.670038381137163519 ) ) ;
#18086=VERTEX_POINT ( 'NONE', #8216 ) ;
#18090=VERTEX_POINT ( 'NONE', #22697 ) ;
#18096=ORIENTED_EDGE ( 'NONE', *, *, #23178, .F. ) ;
#18099=AXIS2_PLACEMENT_3D ( 'NONE', #3329, #12859, #22360 ) ;
#18100=CARTESIAN_POINT ( 'NONE',  ( 3.060137030613569120, 16.80197902060525195, 6.560937769032974209 ) ) ;
#18102=CIRCLE ( 'NONE', #28561, 9.482273699623480212 ) ;
#18103=DIRECTION ( 'NONE',  ( 0.000000000000000000, 0.000000000000000000, 1.000000000000000000 ) ) ;
#18104=CARTESIAN_POINT ( 'NONE',  ( 6.067212148875117173, 19.05774739413747909, 18.72886616302736229 ) ) ;
#18108=CARTESIAN_POINT ( 'NONE',  ( 9.769531821641352920, -13.96399651007160081, 18.35377592296120497 ) ) ;
#18109=CARTESIAN_POINT ( 'NONE',  ( 16.87995935610570442, 2.188012981718272076, 19.33715507985239412 ) ) ;
#18111=CARTESIAN_POINT ( 'NONE',  ( -16.95074943597165174, 1.765291926024246116, 20.34789198813115263 ) ) ;
#18113=CARTESIAN_POINT ( 'NONE',  ( -15.81542570303654749, 12.27127866024200920, 5.951255046771932733 ) ) ;
#18114=CARTESIAN_POINT ( 'NONE',  ( 4.877030535751917029, 19.41475911700131363, 20.25542030744407640 ) ) ;
#18119=CARTESIAN_POINT ( 'NONE',  ( 15.52007383991469069, 12.61466978257045035, 19.08232364404839387 ) ) ;
#18120=B_SPLINE_SURFACE_WITH_KNOTS ( 'NONE', 3, 1, ( 
 ( #27476, #22009 ),
 ( #8294, #3293 ),
 ( #20139, #12823 ),
 ( #19831, #22165 ),
 ( #24352, #7995 ),
 ( #17498, #644 ),
 ( #3609, #27167 ),
 ( #22324, #964 ),
 ( #29355, #2999 ),
 ( #17811, #13130 ),
 ( #15141, #6097 ),
 ( #29657, #22624 ),
 ( #10159, #27325 ),
 ( #12671, #17968 ),
 ( #8465, #27018 ),
 ( #10474, #19987 ),
 ( #5646, #5954 ),
 ( #19666, #26867 ),
 ( #29506, #1274 ),
 ( #3460, #10782 ),
 ( #8143, #5793 ),
 ( #15291, #24821 ),
 ( #12976, #15453 ),
 ( #29823, #7826 ),
 ( #22467, #20297 ),
 ( #17337, #5490 ),
 ( #14991, #15932 ),
 ( #21042, #11238 ),
 ( #28081, #13286 ),
 ( #16218, #6703 ),
 ( #11095, #30564 ) ),
 .UNSPECIFIED., .F., .F., .F.,
 ( 4, 3, 3, 3, 3, 3, 3, 3, 3, 3, 4 ),
 ( 2, 2 ),
 ( 0.4999999998345683316, 0.5360336730431939367, 0.5907651151589012883, 0.6456034593241830599, 0.6998270958050434309, 0.7529536536315937223, 0.8052385063053260073, 0.8575343587103997356, 0.9106564858195042023, 0.9648414833209685293, 1.000000006602610014 ),
 ( 0.000000000000000000, 1.000000000000000000 ),
 .UNSPECIFIED. ) ;
#18121=CARTESIAN_POINT ( 'NONE',  ( -5.119216485953539397, 16.24645747311529931, 20.25336174263950184 ) ) ;
#18123=CIRCLE ( 'NONE', #26074, 20.00000000000000000 ) ;
#18124=DIRECTION ( 'NONE',  ( -0.000000000000000000, -0.000000000000000000, 1.000000000000000000 ) ) ;
#18126=VECTOR ( 'NONE', #15252, 1000.000000000000000 ) ;
#18133=DIRECTION ( 'NONE',  ( -0.4154150130018840481, 0.9096319953545194403, 0.000000000000000000 ) ) ;
#18136=ORIENTED_EDGE ( 'NONE', *, *, #30147, .F. ) ;
#18138=FACE_OUTER_BOUND ( 'NONE', #14657, .T. ) ;
#18144=CARTESIAN_POINT ( 'NONE',  ( -1.246245039005656974, 2.728895986063601509, 24.50000000000000000 ) ) ;
#18149=CARTESIAN_POINT ( 'NONE',  ( 0.7788148826605760799, -17.02744010918315709, 7.652108011868850035 ) ) ;
#18152=ORIENTED_EDGE ( 'NONE', *, *, #18538, .F. ) ;
#18153=EDGE_CURVE ( 'NONE', #315, #23230, #5667, .T. ) ;
#18154=CARTESIAN_POINT ( 'NONE',  ( 9.824744466605370263, -8.513189541288715745, 24.50000000000000000 ) ) ;
#18157=EDGE_CURVE ( 'NONE', #4887, #2392, #3174, .T. ) ;
#18158=CARTESIAN_POINT ( 'NONE',  ( 9.860909911264741368, -13.90333503211347477, 7.652108011868850035 ) ) ;
#18165=LINE ( 'NONE', #15974, #6607 ) ;
#18166=EDGE_LOOP ( 'NONE', ( #21165, #16640, #5258, #14406 ) ) ;
#18167=B_SPLINE_CURVE_WITH_KNOTS ( 'NONE', 3,
 ( #30826, #20852, #27735, #1987, #6366, #18528, #28031, #6809, #9158, #18672, #18834, #28179, #16337, #4484, #26003, #13994, #21141, #30660, #9308, #28351 ),
 .UNSPECIFIED., .F., .F.,
 ( 4, 2, 2, 2, 2, 2, 2, 2, 2, 4 ),
 ( 0.000000000000000000, 0.06250000000000183187, 0.1250000000000036637, 0.1875000000000054956, 0.2187500000000056344, 0.2500000000000057732, 0.3125000000000043299, 0.3750000000000028866, 0.4375000000000014433, 0.5000000000000000000 ),
 .UNSPECIFIED. ) ;
#18168=CYLINDRICAL_SURFACE ( 'NONE', #10426, 9.482273699623480212 ) ;
#18170=CARTESIAN_POINT ( 'NONE',  ( -9.376411575904491258, -14.20642299464377345, 6.864725433338323413 ) ) ;
#18174=EDGE_CURVE ( 'NONE', #24299, #8908, #22250, .T. ) ;
#18187=EDGE_CURVE ( 'NONE', #23990, #8702, #27191, .T. ) ;
#18192=PLANE ( 'NONE',  #24834 ) ;
#18193=CARTESIAN_POINT ( 'NONE',  ( 9.181265710901294952, -14.33790826719505773, 7.267659094423557065 ) ) ;
#18196=ORIENTED_EDGE ( 'NONE', *, *, #8031, .T. ) ;
#18197=DIRECTION ( 'NONE',  ( 1.000000000000000000, 0.000000000000000000, 0.000000000000000000 ) ) ;
#18201=ORIENTED_EDGE ( 'NONE', *, *, #28308, .T. ) ;
#18206=ORIENTED_EDGE ( 'NONE', *, *, #21784, .T. ) ;
#18207=CARTESIAN_POINT ( 'NONE',  ( -19.75958569938476117, 3.205325445645398563, 5.940635272151477686 ) ) ;
#18209=CARTESIAN_POINT ( 'NONE',  ( 14.88222593340885958, 13.36111339922579155, 7.652108011868850035 ) ) ;
#18215=CARTESIAN_POINT ( 'NONE',  ( 5.881244434206234217, 6.812559277181991391, 1.500000000000001332 ) ) ;
#18216=DIRECTION ( 'NONE',  ( 0.000000000000000000, 0.000000000000000000, 1.000000000000000000 ) ) ;
#18218=CARTESIAN_POINT ( 'NONE',  ( -3.912171961292012057, -8.637616862297827325, 13.00000000000000178 ) ) ;
#18222=AXIS2_PLACEMENT_3D ( 'NONE', #24536, #15328, #3183 ) ;
#18223=CARTESIAN_POINT ( 'NONE',  ( 0.7836604620899301210, -17.02735026737548552, 5.652196082368483587 ) ) ;
#18224=CARTESIAN_POINT ( 'NONE',  ( 0.000000000000000000, 0.000000000000000000, 21.50000000000000000 ) ) ;
#18225=DIRECTION ( 'NONE',  ( -0.7557495743542581579, -0.6548607339452852116, 0.000000000000000000 ) ) ;
#18226=CYLINDRICAL_SURFACE ( 'NONE', #17372, 20.00000000000000000 ) ;
#18231=ORIENTED_EDGE ( 'NONE', *, *, #2926, .F. ) ;
#18236=ORIENTED_EDGE ( 'NONE', *, *, #11504, .T. ) ;
#18237=CARTESIAN_POINT ( 'NONE',  ( -4.163336342344337027E-14, 1.387778780781445676E-14, 24.50000000000000000 ) ) ;
#18239=DIRECTION ( 'NONE',  ( 1.000000000000000000, 0.000000000000000000, 0.000000000000000000 ) ) ;
#18240=EDGE_CURVE ( 'NONE', #24029, #6719, #26733, .T. ) ;
#18250=ORIENTED_EDGE ( 'NONE', *, *, #18947, .T. ) ;
#18251=ORIENTED_EDGE ( 'NONE', *, *, #15844, .T. ) ;
#18253=CARTESIAN_POINT ( 'NONE',  ( 4.877030535751920581, 19.41475911700131363, 7.559636331181775581 ) ) ;
#18254=CIRCLE ( 'NONE', #11286, 9.482273699623480212 ) ;
#18255=DIRECTION ( 'NONE',  ( 1.000000000000000000, 0.000000000000000000, 0.000000000000000000 ) ) ;
#18256=LINE ( 'NONE', #20288, #28260 ) ;
#18264=CARTESIAN_POINT ( 'NONE',  ( 15.72291199960845454, -6.567794255929247704, 5.670038381137163519 ) ) ;
#18266=CARTESIAN_POINT ( 'NONE',  ( 4.772488686130579083, 19.44046140540703504, 18.50655187082627862 ) ) ;
#18270=VECTOR ( 'NONE', #19211, 1000.000000000000000 ) ;
#18278=AXIS2_PLACEMENT_3D ( 'NONE', #11020, #10555, #29584 ) ;
#18280=CARTESIAN_POINT ( 'NONE',  ( 2.878478920843542177, 0.8451976705242683074, 24.50000000000000000 ) ) ;
#18283=CARTESIAN_POINT ( 'NONE',  ( 0.3567147238643512130, -19.99681861211370659, 5.652196082369963293 ) ) ;
#18284=FACE_OUTER_BOUND ( 'NONE', #9805, .T. ) ;
#18287=CARTESIAN_POINT ( 'NONE',  ( 4.119120293826439294, 16.53802619141619346, 18.34969686940295830 ) ) ;
#18289=CARTESIAN_POINT ( 'NONE',  ( -19.71415773217920986, 3.369653345580889692, 7.156831654632820339 ) ) ;
#18299=CIRCLE ( 'NONE', #17285, 0.7499999999999997780 ) ;
#18301=CARTESIAN_POINT ( 'NONE',  ( 1.653546806191835250, -16.99301016096993422, 6.131018562779544823 ) ) ;
#18302=CARTESIAN_POINT ( 'NONE',  ( -16.94912694330537306, 1.778434104809240912, 5.651492010659113774 ) ) ;
#18305=DIRECTION ( 'NONE',  ( 0.9594929736144952592, -0.2817325568414371095, 0.000000000000000000 ) ) ;
#18308=CARTESIAN_POINT ( 'NONE',  ( -4.773373620198770872, 16.34284820692472451, 6.031926333436658183 ) ) ;
#18318=CARTESIAN_POINT ( 'NONE',  ( -0.6312581325461337212, -19.99009984789270433, 19.60917204426171168 ) ) ;
#18329=CIRCLE ( 'NONE', #12331, 0.7500000000000015543 ) ;
#18331=AXIS2_PLACEMENT_3D ( 'NONE', #20013, #675, #10504 ) ;
#18334=EDGE_LOOP ( 'NONE', ( #17632, #28995, #10932, #12178 ) ) ;
#18338=CARTESIAN_POINT ( 'NONE',  ( 0.000000000000000000, 0.000000000000000000, 1.500000000000001332 ) ) ;
#18341=AXIS2_PLACEMENT_3D ( 'NONE', #5710, #26788, #12904 ) ;
#18344=CARTESIAN_POINT ( 'NONE',  ( 16.55667234708964486, 4.187688857956195498, 6.521906765011494578 ) ) ;
#18345=DIRECTION ( 'NONE',  ( -0.8412535328311804284, 0.5406408174555987767, 0.000000000000000000 ) ) ;
#18348=DIRECTION ( 'NONE',  ( 0.000000000000000000, 0.000000000000000000, 1.000000000000000000 ) ) ;
#18350=CARTESIAN_POINT ( 'NONE',  ( 1.750000000000008660, 16.48749217771910125, 1.500000000000000000 ) ) ;
#18353=DIRECTION ( 'NONE',  ( 0.8412535328311810945, 0.5406408174555976665, 0.000000000000000000 ) ) ;
#18355=EDGE_LOOP ( 'NONE', ( #18780, #9484, #11009, #2555 ) ) ;
#18356=EDGE_CURVE ( 'NONE', #13536, #24159, #1905, .T. ) ;
#18358=CARTESIAN_POINT ( 'NONE',  ( -14.44122519041009234, -13.83658248990211348, 24.50000000000000000 ) ) ;
#18359=DIRECTION ( 'NONE',  ( 1.000000000000000000, 0.000000000000000000, 0.000000000000000000 ) ) ;
#18367=VECTOR ( 'NONE', #14954, 1000.000000000000000 ) ;
#18371=VERTEX_POINT ( 'NONE', #4396 ) ;
#18372=CARTESIAN_POINT ( 'NONE',  ( -19.86132377132435778, 2.497833445081380166, 5.652196082367002106 ) ) ;
#18374=CARTESIAN_POINT ( 'NONE',  ( 15.21452331804151115, 12.98203751624682667, 5.775318986477954830 ) ) ;
#18375=PLANE ( 'NONE',  #7519 ) ;
#18380=B_SPLINE_CURVE_WITH_KNOTS ( 'NONE', 3,
 ( #25188, #3834, #22853, #1504, #11012, #20513, #8676, #18955, #21429, #25964, #19406, #21580, #26109, #2244, #14571, #19096, #12230, #28924 ),
 .UNSPECIFIED., .F., .F.,
 ( 4, 2, 2, 2, 2, 2, 2, 2, 4 ),
 ( 0.000000000000000000, 0.0003967869494442878304, 0.0007935738988885756608, 0.001190360848332863491, 0.001587147797777151322, 0.001983934747221438935, 0.002380721696665726982, 0.002777508646110015030, 0.003174295595554302643 ),
 .UNSPECIFIED. ) ;
#18381=DIRECTION ( 'NONE',  ( 1.000000000000000000, 0.000000000000000000, 0.000000000000000000 ) ) ;
#18382=CARTESIAN_POINT ( 'NONE',  ( -15.34618562042307310, 12.82554431217321245, 5.652196082369965069 ) ) ;
#18389=B_SPLINE_SURFACE_WITH_KNOTS ( 'NONE', 3, 1, ( 
 ( #6291, #27829 ),
 ( #15803, #6602 ),
 ( #16116, #11444 ),
 ( #30307, #25325 ),
 ( #11137, #6458 ),
 ( #4109, #30601 ),
 ( #4252, #28124 ),
 ( #3968, #13642 ),
 ( #23122, #1768 ),
 ( #18762, #6140 ),
 ( #23275, #16262 ),
 ( #18470, #13776 ),
 ( #1918, #4413 ),
 ( #11285, #15647 ),
 ( #20779, #25159 ),
 ( #2839, #7373 ),
 ( #19061, #23574 ),
 ( #7207, #4561 ),
 ( #24187, #30759 ),
 ( #25930, #14064 ),
 ( #14539, #24036 ),
 ( #5025, #26080 ),
 ( #26232, #37 ),
 ( #2218, #10019 ),
 ( #11736, #11904 ),
 ( #21697, #21229 ),
 ( #18923, #9549 ),
 ( #12361, #14684 ),
 ( #14214, #4713 ),
 ( #21865, #499 ),
 ( #16419, #2537 ) ),
 .UNSPECIFIED., .F., .F., .F.,
 ( 4, 3, 3, 3, 3, 3, 3, 3, 3, 3, 4 ),
 ( 2, 2 ),
 ( 0.4999999998345689423, 0.5360336730431939367, 0.5907651151589012883, 0.6456034593241830599, 0.6998270958050434309, 0.7529536536315937223, 0.8052385063053260073, 0.8575343587103997356, 0.9106564858195042023, 0.9648414833209685293, 1.000000006602610014 ),
 ( 0.000000000000000000, 1.000000000000000000 ),
 .UNSPECIFIED. ) ;
#18390=FACE_OUTER_BOUND ( 'NONE', #8584, .T. ) ;
#18391=VECTOR ( 'NONE', #5673, 1000.000000000000000 ) ;
#18393=CARTESIAN_POINT ( 'NONE',  ( 10.16054539467770113, 13.96046037420044961, 24.50000000000000000 ) ) ;
#18395=CARTESIAN_POINT ( 'NONE',  ( -16.99246856547861739, 1.423159825038152082, 18.37415474056476938 ) ) ;
#18397=ORIENTED_EDGE ( 'NONE', *, *, #11138, .F. ) ;
#18403=ORIENTED_EDGE ( 'NONE', *, *, #3258, .F. ) ;
#18406=CARTESIAN_POINT ( 'NONE',  ( -4.596254364928610059, 16.38944764646978314, 6.864725433338323413 ) ) ;
#18408=CIRCLE ( 'NONE', #22372, 1.000000000000007772 ) ;
#18410=CARTESIAN_POINT ( 'NONE',  ( -12.71614549213497014, 11.31496011770333077, 6.782064869129508899 ) ) ;
#18411=DIRECTION ( 'NONE',  ( 0.000000000000000000, 0.000000000000000000, 1.000000000000000000 ) ) ;
#18418=ORIENTED_EDGE ( 'NONE', *, *, #3520, .T. ) ;
#18425=CARTESIAN_POINT ( 'NONE',  ( -17.58129253318380947, -9.534052292972809539, 6.523620417364448976 ) ) ;
#18427=EDGE_LOOP ( 'NONE', ( #12409, #28475, #28912, #2735 ) ) ;
#18430=CARTESIAN_POINT ( 'NONE',  ( 9.582629137048305878, -14.08615220418400860, 18.39701043959520987 ) ) ;
#18433=CARTESIAN_POINT ( 'NONE',  ( -19.73500371898430217, 3.353449004226455088, 19.87181966307587544 ) ) ;
#18434=CARTESIAN_POINT ( 'NONE',  ( 15.81223571690235730, -6.365019318618788446, 7.652108011868850035 ) ) ;
#18435=CARTESIAN_POINT ( 'NONE',  ( -13.97362136398187182, 9.814707526993062814, 6.995624166085161910 ) ) ;
#18436=CARTESIAN_POINT ( 'NONE',  ( 3.283642163210877207, 16.75135354181591296, 19.97651184436794125 ) ) ;
#18441=CARTESIAN_POINT ( 'NONE',  ( 15.40940123050674693, 12.74987339073082637, 19.96302680909623817 ) ) ;
#18442=CARTESIAN_POINT ( 'NONE',  ( -5.216068956281039171, 19.32652695433950285, 18.71435384576123440 ) ) ;
#18443=CARTESIAN_POINT ( 'NONE',  ( 0.000000000000000000, 0.000000000000000000, 1.500000000000001332 ) ) ;
#18446=CARTESIAN_POINT ( 'NONE',  ( -2.703030265324078307, -12.75514121382991384, 24.50000000000000000 ) ) ;
#18447=ORIENTED_EDGE ( 'NONE', *, *, #15276, .T. ) ;
#18448=CARTESIAN_POINT ( 'NONE',  ( -17.00407983531365019, 1.321870115990435801, 7.603368798681074736 ) ) ;
#18450=CARTESIAN_POINT ( 'NONE',  ( 4.102102735472461958, -8.549050687778175117, 1.500000000000001332 ) ) ;
#18454=CARTESIAN_POINT ( 'NONE',  ( 7.869584159753955532, 10.39565510934977333, 1.500000000000001332 ) ) ;
#18457=CARTESIAN_POINT ( 'NONE',  ( -0.2646837113541495867, -19.99846847964001739, 5.849008070840544526 ) ) ;
#18458=CARTESIAN_POINT ( 'NONE',  ( 9.634323311075775109, 1.438332125858202692, 1.500000000000001332 ) ) ;
#18460=DIRECTION ( 'NONE',  ( -1.000000000000000000, 0.000000000000000000, 0.000000000000000000 ) ) ;
#18461=CIRCLE ( 'NONE', #26419, 10.00000000000000000 ) ;
#18466=CARTESIAN_POINT ( 'NONE',  ( -19.84344116185557283, 2.497567387674354489, 20.34789198813115263 ) ) ;
#18470=CARTESIAN_POINT ( 'NONE',  ( -17.63988435498684382, -9.462624493092880229, 18.92976555901915603 ) ) ;
#18473=VERTEX_POINT ( 'NONE', #12811 ) ;
#18474=LINE ( 'NONE', #7060, #23367 ) ;
#18480=PLANE ( 'NONE',  #14101 ) ;
#18487=CARTESIAN_POINT ( 'NONE',  ( -10.23401665697056195, -17.20427178438287186, 5.704143890883081269 ) ) ;
#18491=CARTESIAN_POINT ( 'NONE',  ( 12.18183868328554809, 11.93592587881222933, 20.34789198813114908 ) ) ;
#18495=EDGE_CURVE ( 'NONE', #23990, #2092, #9806, .T. ) ;
#18498=VECTOR ( 'NONE', #24145, 1000.000000000000000 ) ;
#18503=CARTESIAN_POINT ( 'NONE',  ( -18.44586851731391519, -7.729974993529595828, 19.60917204426171168 ) ) ;
#18504=CARTESIAN_POINT ( 'NONE',  ( -15.56851150445305088, -6.881932713941044888, 19.56050940960062690 ) ) ;
#18505=CARTESIAN_POINT ( 'NONE',  ( -9.290115248478288734, -14.26557846606243807, 19.85270094495842130 ) ) ;
#18506=VERTEX_POINT ( 'NONE', #487 ) ;
#18508=EDGE_CURVE ( 'NONE', #23584, #7538, #633, .T. ) ;
#18514=CARTESIAN_POINT ( 'NONE',  ( 15.58729175431054337, -6.863221649612937014, 20.19668224736330941 ) ) ;
#18517=CARTESIAN_POINT ( 'NONE',  ( -19.70840172719294614, 3.506524300503914837, 6.641371103590088865 ) ) ;
#18518=AXIS2_PLACEMENT_3D ( 'NONE', #4392, #16545, #7192 ) ;
#18519=CARTESIAN_POINT ( 'NONE',  ( -10.89423172471906831, -16.79374140667819759, 18.44501272782439827 ) ) ;
#18526=FACE_OUTER_BOUND ( 'NONE', #212, .T. ) ;
#18528=CARTESIAN_POINT ( 'NONE',  ( 16.85625572095001701, 2.395390699382102362, 19.96344307082652492 ) ) ;
#18530=CARTESIAN_POINT ( 'NONE',  ( -5.976020107417636673, 19.08630880174946043, 18.34798005863226678 ) ) ;
#18531=CARTESIAN_POINT ( 'NONE',  ( -0.1401636875787305447, -17.02258069761206372, 7.080843742048788414 ) ) ;
#18532=CARTESIAN_POINT ( 'NONE',  ( 15.81416692036122207, -6.360574302898111654, 18.34798005863078885 ) ) ;
#18533=DIRECTION ( 'NONE',  ( 0.9096319953545183301, 0.4154150130018865461, 0.000000000000000000 ) ) ;
#18534=CARTESIAN_POINT ( 'NONE',  ( -17.06249589246193565, 0.6902251470929382515, 19.03762469184452755 ) ) ;
#18535=DIRECTION ( 'NONE',  ( 0.000000000000000000, 0.000000000000000000, 1.000000000000000000 ) ) ;
#18538=EDGE_CURVE ( 'NONE', #14619, #8580, #18785, .T. ) ;
#18539=CARTESIAN_POINT ( 'NONE',  ( -6.458576814766982643, 15.80792270644319331, 6.329955581934036069 ) ) ;
#18542=ADVANCED_FACE ( 'NONE', ( #15132 ), #12506, .F. ) ;
#18545=ADVANCED_FACE ( 'NONE', ( #29026 ), #3153, .T. ) ;
#18549=CARTESIAN_POINT ( 'NONE',  ( -11.82521593960875528, 5.400395169024524655, 1.500000000000001332 ) ) ;
#18565=CARTESIAN_POINT ( 'NONE',  ( 0.2718907110559959928, -17.03030470364380733, 20.22273502201483453 ) ) ;
#18568=CARTESIAN_POINT ( 'NONE',  ( 8.549050687778162683, 4.102102735472485051, 21.50000000000000000 ) ) ;
#18569=CARTESIAN_POINT ( 'NONE',  ( 19.87213478643044340, 2.412525337365567513, 18.71435384576123440 ) ) ;
#18570=ORIENTED_EDGE ( 'NONE', *, *, #1000, .T. ) ;
#18571=EDGE_CURVE ( 'NONE', #8044, #8694, #5094, .T. ) ;
#18572=VECTOR ( 'NONE', #27091, 1000.000000000000000 ) ;
#18573=CARTESIAN_POINT ( 'NONE',  ( 10.74273727477993390, -16.89139546617319354, 7.557577766377196582 ) ) ;
#18575=CARTESIAN_POINT ( 'NONE',  ( -13.99683207193583279, 9.784088562599672301, 6.892848776733236704 ) ) ;
#18576=CARTESIAN_POINT ( 'NONE',  ( 4.400293182487616583, 19.52803631353506120, 18.92976555901915603 ) ) ;
#18578=EDGE_LOOP ( 'NONE', ( #20572, #27919, #12941, #23206 ) ) ;
#18584=DIRECTION ( 'NONE',  ( -1.000000000000000000, 0.000000000000000000, 0.000000000000000000 ) ) ;
#18585=ADVANCED_FACE ( 'NONE', ( #14606 ), #29305, .T. ) ;
#18587=ADVANCED_FACE ( 'NONE', ( #3063 ), #29267, .T. ) ;
#18589=CARTESIAN_POINT ( 'NONE',  ( 1.368946144808715015, -19.95309466511745811, 6.523620417364439206 ) ) ;
#18590=CARTESIAN_POINT ( 'NONE',  ( -5.604556300746500241, -15.53790034020399169, 24.50000000000000000 ) ) ;
#18593=FACE_OUTER_BOUND ( 'NONE', #21752, .T. ) ;
#18595=EDGE_LOOP ( 'NONE', ( #25412, #29069 ) ) ;
#18603=CARTESIAN_POINT ( 'NONE',  ( 13.00999358272542850, -0.8602714556717643291, 1.500000000000001332 ) ) ;
#18604=CARTESIAN_POINT ( 'NONE',  ( -6.656778417335413423, 18.87854210339739325, 20.06253562465620632 ) ) ;
#18609=CARTESIAN_POINT ( 'NONE',  ( 0.000000000000000000, 0.000000000000000000, 1.500000000000001332 ) ) ;
#18610=CARTESIAN_POINT ( 'NONE',  ( 15.81223572262636878, -6.365019322297388094, 20.34789198813115263 ) ) ;
#18611=ORIENTED_EDGE ( 'NONE', *, *, #22710, .T. ) ;
#18613=AXIS2_PLACEMENT_3D ( 'NONE', #11209, #17937, #4036 ) ;
#18615=VECTOR ( 'NONE', #11559, 1000.000000000000227 ) ;
#18617=VERTEX_POINT ( 'NONE', #15198 ) ;
#18618=CARTESIAN_POINT ( 'NONE',  ( -0.1522245795255700584, -19.99979613760744002, 18.47110296274026098 ) ) ;
#18621=DIRECTION ( 'NONE',  ( -0.2817325568414293380, -0.9594929736144974797, 0.000000000000000000 ) ) ;
#18622=VERTEX_POINT ( 'NONE', #14748 ) ;
#18623=CARTESIAN_POINT ( 'NONE',  ( -13.99139173414245185, 9.791236547353763697, 6.392658652357120275 ) ) ;
#18624=ORIENTED_EDGE ( 'NONE', *, *, #23873, .F. ) ;
#18627=CARTESIAN_POINT ( 'NONE',  ( 4.102102735472459294, -8.549050687778176894, 13.00000000000000178 ) ) ;
#18628=EDGE_CURVE ( 'NONE', #24994, #5507, #17417, .T. ) ;
#18631=CARTESIAN_POINT ( 'NONE',  ( 16.65271093598738261, 3.715728438010606816, 18.45571264222803620 ) ) ;
#18634=VECTOR ( 'NONE', #13786, 1000.000000000000114 ) ;
#18637=CARTESIAN_POINT ( 'NONE',  ( 7.028330626922776325, 10.93629592680536966, 1.500000000000001332 ) ) ;
#18645=CARTESIAN_POINT ( 'NONE',  ( -18.58529988941444344, 7.388276390372320535, 24.50000000000000000 ) ) ;
#18648=CARTESIAN_POINT ( 'NONE',  ( 3.790840891470688589, 16.62820496721823815, 18.34938820207545618 ) ) ;
#18650=CARTESIAN_POINT ( 'NONE',  ( -15.57772019539775421, -6.859948791675929414, 19.45164628100866722 ) ) ;
#18654=DIRECTION ( 'NONE',  ( 0.5406408174555974444, 0.8412535328311813165, 0.000000000000000000 ) ) ;
#18655=CARTESIAN_POINT ( 'NONE',  ( -7.671651850954201990, -15.25824679864873445, 6.588756557121049795 ) ) ;
#18659=CARTESIAN_POINT ( 'NONE',  ( 15.51152286861889529, -7.023094163498092790, 20.05479082170252525 ) ) ;
#18660=CARTESIAN_POINT ( 'NONE',  ( 5.021901920966175048, 16.26348455184633579, 6.641371103590088865 ) ) ;
#18662=CARTESIAN_POINT ( 'NONE',  ( -16.83148396119934631, 2.548526378087588640, 6.211014596808754007 ) ) ;
#18663=CARTESIAN_POINT ( 'NONE',  ( 14.20032907733019556, 14.10870362182394722, 6.782048567692550378 ) ) ;
#18667=CARTESIAN_POINT ( 'NONE',  ( -1.195154792889455697, -9.406652940105981742, 13.00000000000000178 ) ) ;
#18668=CARTESIAN_POINT ( 'NONE',  ( -14.70620249426165849, -8.682611668023952234, 6.521906765011494578 ) ) ;
#18669=CARTESIAN_POINT ( 'NONE',  ( -14.94050307174418712, 13.29624634855319698, 5.849008070840538309 ) ) ;
#18672=CARTESIAN_POINT ( 'NONE',  ( 16.87858066272376689, 2.200498455871256365, 19.47784884541372108 ) ) ;
#18678=CARTESIAN_POINT ( 'NONE',  ( -2.810445847081918913, -9.056208293496299078, 13.00000000000000178 ) ) ;
#18679=CARTESIAN_POINT ( 'NONE',  ( -19.96205336850438883, 1.490391487655212899, 19.36813350477385143 ) ) ;
#18681=ORIENTED_EDGE ( 'NONE', *, *, #23679, .T. ) ;
#18684=ORIENTED_EDGE ( 'NONE', *, *, #7846, .T. ) ;
#18686=CARTESIAN_POINT ( 'NONE',  ( 10.47960520055065992, -7.757439966934453146, 1.500000000000001332 ) ) ;
#18702=EDGE_CURVE ( 'NONE', #13171, #7773, #22758, .T. ) ;
#18707=CARTESIAN_POINT ( 'NONE',  ( -17.64439154790314390, -9.416908767371234390, 7.161525567826898531 ) ) ;
#18708=VECTOR ( 'NONE', #9701, 1000.000000000000000 ) ;
#18709=DIRECTION ( 'NONE',  ( 1.000000000000000000, 0.000000000000000000, 0.000000000000000000 ) ) ;
#18711=CARTESIAN_POINT ( 'NONE',  ( 19.81199842303382042, 2.865066961627989350, 18.39701043959520987 ) ) ;
#18713=CARTESIAN_POINT ( 'NONE',  ( -16.92089108241427198, 1.982400079378048963, 18.39701043959520987 ) ) ;
#18716=CARTESIAN_POINT ( 'NONE',  ( -15.76141475779636814, 12.34077778289584160, 5.872146474157316831 ) ) ;
#18717=DIRECTION ( 'NONE',  ( -0.7557495743542579358, 0.6548607339452854337, -0.000000000000000000 ) ) ;
#18721=EDGE_CURVE ( 'NONE', #14619, #5400, #20196, .T. ) ;
#18722=CARTESIAN_POINT ( 'NONE',  ( 6.187077094091595342, 11.47693674426096599, 1.500000000000001332 ) ) ;
#18723=EDGE_CURVE ( 'NONE', #8908, #30200, #8367, .T. ) ;
#18724=CARTESIAN_POINT ( 'NONE',  ( 5.687793815610356241, -6.974883619896809606, 21.50000000000000000 ) ) ;
#18732=CARTESIAN_POINT ( 'NONE',  ( 1.159631224985658848, -19.96657546246603587, 7.272192800924335288 ) ) ;
#18733=CARTESIAN_POINT ( 'NONE',  ( 14.46116907065692914, 13.81605838820131638, 20.15039051365863543 ) ) ;
#18734=CARTESIAN_POINT ( 'NONE',  ( -8.999114229549592281, 0.1262659238205133538, 21.50000000000000000 ) ) ;
#18735=EDGE_CURVE ( 'NONE', #16362, #26160, #12926, .T. ) ;
#18738=VERTEX_POINT ( 'NONE', #30032 ) ;
#18739=EDGE_CURVE ( 'NONE', #23193, #1001, #30475, .T. ) ;
#18740=CARTESIAN_POINT ( 'NONE',  ( 16.14429390779611850, -5.555032456232104288, 6.131018562779544823 ) ) ;
#18741=AXIS2_PLACEMENT_3D ( 'NONE', #7074, #16583, #9568 ) ;
#18742=ORIENTED_EDGE ( 'NONE', *, *, #575, .F. ) ;
#18748=CARTESIAN_POINT ( 'NONE',  ( -6.922783288613183039, 18.78247243577000347, 19.14333282897057842 ) ) ;
#18750=DIRECTION ( 'NONE',  ( -0.000000000000000000, -0.000000000000000000, 1.000000000000000000 ) ) ;
#18751=CARTESIAN_POINT ( 'NONE',  ( 0.9307681286968572110, -9.436481611552755666, 1.500000000000001332 ) ) ;
#18754=EDGE_CURVE ( 'NONE', #4645, #12148, #18299, .T. ) ;
#18758=CARTESIAN_POINT ( 'NONE',  ( -8.743977807160096205, -3.668292057955974350, 21.50000000000000000 ) ) ;
#18760=DIRECTION ( 'NONE',  ( -1.000000000000000000, 0.000000000000000000, 0.000000000000000000 ) ) ;
#18762=CARTESIAN_POINT ( 'NONE',  ( -17.69908921317806971, -9.351398086983023106, 18.73743063545763121 ) ) ;
#18763=EDGE_CURVE ( 'NONE', #17664, #16485, #30247, .T. ) ;
#18764=CARTESIAN_POINT ( 'NONE',  ( -13.37849590498012553, 10.56201291617987792, 20.34789198813115263 ) ) ;
#18769=ORIENTED_EDGE ( 'NONE', *, *, #9731, .F. ) ;
#18770=FACE_OUTER_BOUND ( 'NONE', #17179, .T. ) ;
#18773=PLANE ( 'NONE',  #21035 ) ;
#18776=DIRECTION ( 'NONE',  ( 1.000000000000000000, 0.000000000000000000, 0.000000000000000000 ) ) ;
#18780=ORIENTED_EDGE ( 'NONE', *, *, #29254, .F. ) ;
#18784=CARTESIAN_POINT ( 'NONE',  ( 0.4458717728788682555, -17.03078575579515785, 18.39701043959520987 ) ) ;
#18785=CIRCLE ( 'NONE', #25262, 0.7500000000000006661 ) ;
#18789=CARTESIAN_POINT ( 'NONE',  ( 1.653546806191835694, -16.99301016096993067, 18.82680253904184298 ) ) ;
#18790=ORIENTED_EDGE ( 'NONE', *, *, #13948, .F. ) ;
#18792=DIRECTION ( 'NONE',  ( 1.000000000000000000, 0.000000000000000000, 0.000000000000000000 ) ) ;
#18800=CARTESIAN_POINT ( 'NONE',  ( -13.29701885108704751, 10.65950381955433102, 18.34727598691067740 ) ) ;
#18803=CARTESIAN_POINT ( 'NONE',  ( -18.25684187146043058, -8.167166100028884657, 20.22277707861863050 ) ) ;
#18805=FACE_OUTER_BOUND ( 'NONE', #3171, .T. ) ;
#18816=CARTESIAN_POINT ( 'NONE',  ( 18.16954353748349860, -8.401983848419027012, 20.25336174263950184 ) ) ;
#18817=CARTESIAN_POINT ( 'NONE',  ( 6.262709072525336929, 19.01302309856008321, 6.530762810602277924 ) ) ;
#18818=AXIS2_PLACEMENT_3D ( 'NONE', #9614, #19124, #14446 ) ;
#18822=CARTESIAN_POINT ( 'NONE',  ( 14.40720023010961981, 13.89764844773314501, 7.366751648393900176 ) ) ;
#18829=CARTESIAN_POINT ( 'NONE',  ( -15.25895845836713605, 12.92986402562788406, 7.652108011868849147 ) ) ;
#18832=AXIS2_PLACEMENT_3D ( 'NONE', #23596, #28759, #14235 ) ;
#18833=CARTESIAN_POINT ( 'NONE',  ( -15.51938817160315232, -6.998174447281578558, 7.176035686813569292 ) ) ;
#18834=CARTESIAN_POINT ( 'NONE',  ( 16.87927834490895052, 2.194149605794880831, 19.41069149716888020 ) ) ;
#18837=CARTESIAN_POINT ( 'NONE',  ( 0.05528831664089196157, -17.02727625121208632, 7.359006845440219102 ) ) ;
#18840=CARTESIAN_POINT ( 'NONE',  ( 0.000000000000000000, 0.000000000000000000, 21.50000000000000000 ) ) ;
#18841=DIRECTION ( 'NONE',  ( -0.000000000000000000, -0.000000000000000000, 1.000000000000000000 ) ) ;
#18845=CARTESIAN_POINT ( 'NONE',  ( -5.800828033475949219, 16.03801949186916431, 5.653604225791663218 ) ) ;
#18851=DIRECTION ( 'NONE',  ( -0.000000000000000000, -0.000000000000000000, 1.000000000000000000 ) ) ;
#18857=DIRECTION ( 'NONE',  ( 1.000000000000000000, 0.000000000000000000, 0.000000000000000000 ) ) ;
#18858=CYLINDRICAL_SURFACE ( 'NONE', #15976, 0.7500000000000006661 ) ;
#18861=ORIENTED_EDGE ( 'NONE', *, *, #25566, .T. ) ;
#18864=AXIS2_PLACEMENT_3D ( 'NONE', #15618, #24668, #5966 ) ;
#18868=CARTESIAN_POINT ( 'NONE',  ( -0.2028048457280972328, -17.02068360090513721, 19.08155846658119259 ) ) ;
#18870=CARTESIAN_POINT ( 'NONE',  ( 0.4236634240584232769, -20.01342612130734722, 7.652108011868850035 ) ) ;
#18873=DIRECTION ( 'NONE',  ( -0.000000000000000000, -0.000000000000000000, 1.000000000000000000 ) ) ;
#18875=EDGE_CURVE ( 'NONE', #15172, #4676, #2338, .T. ) ;
#18880=ORIENTED_EDGE ( 'NONE', *, *, #6578, .F. ) ;
#18884=CARTESIAN_POINT ( 'NONE',  ( 1.000000000000008438, 19.97498435543819184, 24.50000000000000000 ) ) ;
#18888=CARTESIAN_POINT ( 'NONE',  ( 4.340342926364955112, 8.430595340551274575, 13.00000000000000178 ) ) ;
#18894=CARTESIAN_POINT ( 'NONE',  ( -19.95825857724417318, 1.540497788607360752, 6.341840715582230281 ) ) ;
#18895=VECTOR ( 'NONE', #30399, 1000.000000000000000 ) ;
#18899=CARTESIAN_POINT ( 'NONE',  ( -9.824744466605366711, -8.513189541288717521, 1.500000000000001332 ) ) ;
#18900=EDGE_LOOP ( 'NONE', ( #16699, #25441, #27718, #8589 ) ) ;
#18903=CARTESIAN_POINT ( 'NONE',  ( 0.3518703668723787148, -19.99690444156084723, 7.652108011868850035 ) ) ;
#18909=B_SPLINE_CURVE_WITH_KNOTS ( 'NONE', 3,
 ( #25969, #28320, #23765, #2248, #23458, #23153, #25665, #6946, #4454, #11945, #20960, #11769, #2418, #11621, #11476, #16455, #30796, #30484, #18800, #21112 ),
 .UNSPECIFIED., .F., .F.,
 ( 4, 2, 2, 2, 2, 2, 2, 2, 2, 4 ),
 ( 0.000000000000000000, 0.06250000000000177636, 0.1250000000000035527, 0.1875000000000053291, 0.2187500000000054678, 0.2500000000000056066, 0.3125000000000042188, 0.3750000000000028311, 0.4375000000000014433, 0.5000000000000000000 ),
 .UNSPECIFIED. ) ;
#18911=CARTESIAN_POINT ( 'NONE',  ( -18.44586851731391519, -7.729974993529599381, 6.913388067999409081 ) ) ;
#18912=DIRECTION ( 'NONE',  ( -0.000000000000000000, -0.000000000000000000, -1.000000000000000000 ) ) ;
#18913=DIRECTION ( 'NONE',  ( 0.7557495743542581579, 0.6548607339452852116, -0.000000000000000000 ) ) ;
#18921=EDGE_CURVE ( 'NONE', #15693, #8747, #12305, .T. ) ;
#18923=CARTESIAN_POINT ( 'NONE',  ( -17.91516185886248635, -8.931344358737691280, 20.29915277494337644 ) ) ;
#18930=CARTESIAN_POINT ( 'NONE',  ( -0.2664633505552017056, -19.99844781589862563, 20.14992337338002670 ) ) ;
#18934=CARTESIAN_POINT ( 'NONE',  ( -6.809999484610175458, 18.80496293131999863, 7.161525567826885208 ) ) ;
#18935=VERTEX_POINT ( 'NONE', #4900 ) ;
#18938=FACE_BOUND ( 'NONE', #10834, .T. ) ;
#18940=VERTEX_POINT ( 'NONE', #5056 ) ;
#18943=ORIENTED_EDGE ( 'NONE', *, *, #9181, .F. ) ;
#18945=CARTESIAN_POINT ( 'NONE',  ( 0.6650193650332599793, -17.02944248263315785, 20.34789198813115263 ) ) ;
#18947=EDGE_CURVE ( 'NONE', #24164, #30839, #29325, .T. ) ;
#18948=CARTESIAN_POINT ( 'NONE',  ( -10.06548534245862747, -17.30301317789299631, 7.500147780736496017 ) ) ;
#18950=CARTESIAN_POINT ( 'NONE',  ( 0.9949940796826611811, -19.99317329078838057, 18.56793045041961321 ) ) ;
#18955=CARTESIAN_POINT ( 'NONE',  ( 1.342668813586976206, -19.95494644892924185, 19.08830981656263859 ) ) ;
#18956=DIRECTION ( 'NONE',  ( -0.000000000000000000, -0.000000000000000000, 1.000000000000000000 ) ) ;
#18961=DIRECTION ( 'NONE',  ( 0.000000000000000000, 0.000000000000000000, 1.000000000000000000 ) ) ;
#18962=CARTESIAN_POINT ( 'NONE',  ( -18.30120037456298121, -8.066899270990504078, 18.54479204710284890 ) ) ;
#18967=ORIENTED_EDGE ( 'NONE', *, *, #17100, .F. ) ;
#18971=CARTESIAN_POINT ( 'NONE',  ( 11.91611018267552247, -16.06265986513583854, 19.61564845152809156 ) ) ;
#18972=ORIENTED_EDGE ( 'NONE', *, *, #12625, .F. ) ;
#18974=CARTESIAN_POINT ( 'NONE',  ( 17.92822150912323309, -8.904799031605451276, 19.22654678686458141 ) ) ;
#18975=CARTESIAN_POINT ( 'NONE',  ( 5.624045005368200734, 19.21181948662072969, 5.701226463332907279 ) ) ;
#18977=ORIENTED_EDGE ( 'NONE', *, *, #15917, .T. ) ;
#18978=CARTESIAN_POINT ( 'NONE',  ( 14.89737979318874572, 13.37085219355980570, 7.652108011868850035 ) ) ;
#18988=CARTESIAN_POINT ( 'NONE',  ( -15.56851150445305443, -6.881932713941046664, 6.864725433338323413 ) ) ;
#18991=CARTESIAN_POINT ( 'NONE',  ( -0.2073672225646047973, -17.02047435233534145, 6.864725433338323413 ) ) ;
#19001=CARTESIAN_POINT ( 'NONE',  ( -15.97601187733368278, 12.03191775062556879, 6.523620417364449864 ) ) ;
#19002=DIRECTION ( 'NONE',  ( 1.000000000000000000, 0.000000000000000000, 0.000000000000000000 ) ) ;
#19003=EDGE_LOOP ( 'NONE', ( #13871, #24203, #3477, #27255 ) ) ;
#19004=CARTESIAN_POINT ( 'NONE',  ( 14.89738168138696217, 13.37085340703111669, 20.34789198813115263 ) ) ;
#19007=CARTESIAN_POINT ( 'NONE',  ( 16.17688602565675282, -5.469326772727303165, 19.03762469184452755 ) ) ;
#19008=CARTESIAN_POINT ( 'NONE',  ( 16.56029649016583605, 4.170884463584000557, 19.58863275299554019 ) ) ;
#19009=EDGE_CURVE ( 'NONE', #16284, #13582, #30137, .T. ) ;
#19010=DIRECTION ( 'NONE',  ( 1.000000000000000000, 0.000000000000000000, 0.000000000000000000 ) ) ;
#19011=EDGE_CURVE ( 'NONE', #23254, #19951, #11122, .T. ) ;
#19012=ORIENTED_EDGE ( 'NONE', *, *, #25792, .T. ) ;
#19014=CARTESIAN_POINT ( 'NONE',  ( 15.40017468080184315, -7.251222802971749815, 19.60617949693493500 ) ) ;
#19017=ORIENTED_EDGE ( 'NONE', *, *, #8613, .F. ) ;
#19018=CARTESIAN_POINT ( 'NONE',  ( -4.163336342344337027E-14, 1.387778780781445676E-14, 24.50000000000000000 ) ) ;
#19021=CARTESIAN_POINT ( 'NONE',  ( 1.153863525602934592, -19.98436899483066753, 6.041646659195333058 ) ) ;
#19023=CARTESIAN_POINT ( 'NONE',  ( 1.762690206876408761, -16.98588469933353196, 19.08844262864050023 ) ) ;
#19025=CARTESIAN_POINT ( 'NONE',  ( 10.44014025173321514, -17.07989312292649942, 7.272049892295485485 ) ) ;
#19031=DIRECTION ( 'NONE',  ( 0.000000000000000000, 0.000000000000000000, 1.000000000000000000 ) ) ;
#19033=CARTESIAN_POINT ( 'NONE',  ( -6.187077094091591789, 11.47693674426096955, 1.500000000000001332 ) ) ;
#19038=EDGE_LOOP ( 'NONE', ( #2757, #4403, #6121, #14368 ) ) ;
#19040=CARTESIAN_POINT ( 'NONE',  ( 14.33033395197103843, 13.95171706641511378, 19.96797677718662811 ) ) ;
#19042=VERTEX_POINT ( 'NONE', #13627 ) ;
#19044=VERTEX_POINT ( 'NONE', #10974 ) ;
#19050=AXIS2_PLACEMENT_3D ( 'NONE', #9782, #6823, #19146 ) ;
#19051=CARTESIAN_POINT ( 'NONE',  ( 10.67036453489834003, -13.33339184394925070, 19.61324152429827095 ) ) ;
#19052=CARTESIAN_POINT ( 'NONE',  ( -18.15587082468813307, -8.389233089038013347, 7.626647697317579855 ) ) ;
#19054=CARTESIAN_POINT ( 'NONE',  ( 10.68225562352957247, -16.90870462272444286, 20.22277707861861984 ) ) ;
#19061=CARTESIAN_POINT ( 'NONE',  ( -17.59999711780629994, -9.536506973003673338, 19.47783254395485031 ) ) ;
#19067=CARTESIAN_POINT ( 'NONE',  ( 6.974883619896790954, 5.687793815610376669, 21.50000000000000000 ) ) ;
#19079=EDGE_CURVE ( 'NONE', #25672, #25827, #25563, .T. ) ;
#19082=EDGE_CURVE ( 'NONE', #6597, #19542, #30270, .T. ) ;
#19086=EDGE_CURVE ( 'NONE', #11240, #17664, #18329, .T. ) ;
#19087=CARTESIAN_POINT ( 'NONE',  ( -8.266165397079792143, -14.91833037834293840, 7.603368798681074736 ) ) ;
#19090=CARTESIAN_POINT ( 'NONE',  ( 0.7788148826605766351, -17.02744010918315354, 20.34789198813115263 ) ) ;
#19094=VECTOR ( 'NONE', #19958, 1000.000000000000000 ) ;
#19096=CARTESIAN_POINT ( 'NONE',  ( 0.6154569680869020898, -19.99089747819055418, 20.32200205377525037 ) ) ;
#19097=CARTESIAN_POINT ( 'NONE',  ( -4.163336342344337027E-14, 1.387778780781445676E-14, 24.50000000000000000 ) ) ;
#19102=DIRECTION ( 'NONE',  ( 0.000000000000000000, 0.000000000000000000, 1.000000000000000000 ) ) ;
#19103=CARTESIAN_POINT ( 'NONE',  ( -19.87500762523393050, 2.235808837979148311, 7.626218077512941562 ) ) ;
#19104=CARTESIAN_POINT ( 'NONE',  ( 19.74328841314636307, 3.194145055459935101, 7.652108011868850035 ) ) ;
#19105=CARTESIAN_POINT ( 'NONE',  ( -18.10797733959156020, -8.533081443083743167, 18.35377592296120497 ) ) ;
#19107=ORIENTED_EDGE ( 'NONE', *, *, #21639, .T. ) ;
#19112=EDGE_CURVE ( 'NONE', #25215, #29598, #23414, .T. ) ;
#19113=CARTESIAN_POINT ( 'NONE',  ( 11.32565050298867959, -16.48467196965850690, 20.32200205377525393 ) ) ;
#19115=AXIS2_PLACEMENT_3D ( 'NONE', #19407, #18956, #28925 ) ;
#19116=CARTESIAN_POINT ( 'NONE',  ( 15.45343642833785935, -7.142940632752240226, 18.80699882434806369 ) ) ;
#19117=CARTESIAN_POINT ( 'NONE',  ( 4.870982490315499902, 16.31268916845847627, 6.111214848085761986 ) ) ;
#19124=DIRECTION ( 'NONE',  ( 0.4154150130018859910, 0.9096319953545186632, 0.000000000000000000 ) ) ;
#19132=CARTESIAN_POINT ( 'NONE',  ( -15.45998620766333431, -7.136073936211801083, 5.940635272151477686 ) ) ;
#19136=CARTESIAN_POINT ( 'NONE',  ( -0.01062192699083326121, -17.02590662965304347, 6.018569869498933578 ) ) ;
#19138=DIRECTION ( 'NONE',  ( 0.000000000000000000, 0.000000000000000000, -1.000000000000000000 ) ) ;
#19139=AXIS2_PLACEMENT_3D ( 'NONE', #22598, #1090, #7644 ) ;
#19140=DIRECTION ( 'NONE',  ( -0.000000000000000000, -0.000000000000000000, 1.000000000000000000 ) ) ;
#19145=CARTESIAN_POINT ( 'NONE',  ( -6.047835543919368284, 15.95440705812618809, 5.759928666072748449 ) ) ;
#19146=DIRECTION ( 'NONE',  ( -1.000000000000000000, 0.000000000000000000, 0.000000000000000000 ) ) ;
#19150=CARTESIAN_POINT ( 'NONE',  ( -15.89797731339010234, 12.13494807016273924, 6.149077423860697778 ) ) ;
#19157=CARTESIAN_POINT ( 'NONE',  ( 18.71162862491809875, -7.111980085401800267, 19.69140814234746273 ) ) ;
#19158=CARTESIAN_POINT ( 'NONE',  ( -8.824744466605359605, -8.513189541288717521, 24.50000000000000000 ) ) ;
#19160=CARTESIAN_POINT ( 'NONE',  ( 15.38884489568443037, -7.274072546993983757, 19.47784884541372818 ) ) ;
#19165=LINE ( 'NONE', #29143, #8663 ) ;
#19167=CARTESIAN_POINT ( 'NONE',  ( -14.71622834324241147, -8.664216105422211101, 19.61324152429827095 ) ) ;
#19168=CARTESIAN_POINT ( 'NONE',  ( 1.664698296051879023, -16.99226504954120287, 19.85459532544248873 ) ) ;
#19169=CARTESIAN_POINT ( 'NONE',  ( 19.82606750293204811, 2.764250834391621225, 18.44501272782439827 ) ) ;
#19171=CARTESIAN_POINT ( 'NONE',  ( -16.89118935510124331, 2.183074208216233547, 18.49267272388512140 ) ) ;
#19178=CARTESIAN_POINT ( 'NONE',  ( -4.163336342344337027E-14, 1.387778780781445676E-14, 1.500000000000000000 ) ) ;
#19179=CYLINDRICAL_SURFACE ( 'NONE', #8875, 0.7500000000000006661 ) ;
#19180=CARTESIAN_POINT ( 'NONE',  ( -5.369726540290506556, 19.28438192063506662, 18.55820869691756769 ) ) ;
#19181=CARTESIAN_POINT ( 'NONE',  ( -15.52715705409340785, -6.980092275572870264, 6.143977687428009204 ) ) ;
#19182=CARTESIAN_POINT ( 'NONE',  ( 0.000000000000000000, 0.000000000000000000, 21.50000000000000000 ) ) ;
#19183=CARTESIAN_POINT ( 'NONE',  ( -5.976020107417634009, 19.08630880174946043, 5.652196082369965069 ) ) ;
#19186=FACE_OUTER_BOUND ( 'NONE', #16503, .T. ) ;
#19189=CARTESIAN_POINT ( 'NONE',  ( 13.01404215953674104, 10.97082360537801549, 6.755862304746362845 ) ) ;
#19190=ORIENTED_EDGE ( 'NONE', *, *, #26687, .T. ) ;
#19191=CARTESIAN_POINT ( 'NONE',  ( 16.15906311113807803, -5.516254886378326283, 7.098451512883313441 ) ) ;
#19193=B_SPLINE_CURVE_WITH_KNOTS ( 'NONE', 3,
 ( #4548, #21385, #19052, #16404, #26069, #14673, #21215, #18911, #6890, #25918, #28724, #14526, #24024, #4700, #21686, #28886, #16870, #7197 ),
 .UNSPECIFIED., .F., .F.,
 ( 4, 2, 2, 2, 2, 2, 2, 2, 4 ),
 ( 0.003174295595554331266, 0.003570702171545574004, 0.003967108747536816742, 0.004363515323528056010, 0.004759921899519296146, 0.005156328475510535414, 0.005552735051501772948, 0.005949141627493012216, 0.006345548203484250617 ),
 .UNSPECIFIED. ) ;
#19194=DIRECTION ( 'NONE',  ( 1.000000000000000000, 0.000000000000000000, 0.000000000000000000 ) ) ;
#19195=ORIENTED_EDGE ( 'NONE', *, *, #18739, .F. ) ;
#19197=CARTESIAN_POINT ( 'NONE',  ( 3.971879806607525598, 16.57852306707252055, 5.652605728828375753 ) ) ;
#19203=CARTESIAN_POINT ( 'NONE',  ( 15.70571165143382508, -6.606148062399648246, 7.626437579292364433 ) ) ;
#19205=CIRCLE ( 'NONE', #6281, 0.7500000000000006661 ) ;
#19209=CARTESIAN_POINT ( 'NONE',  ( 9.056208293496309736, -2.810445847081889159, 21.50000000000000000 ) ) ;
#19211=DIRECTION ( 'NONE',  ( -0.000000000000000000, -0.000000000000000000, 1.000000000000000000 ) ) ;
#19222=FACE_OUTER_BOUND ( 'NONE', #30287, .T. ) ;
#19223=ORIENTED_EDGE ( 'NONE', *, *, #8248, .T. ) ;
#19225=CARTESIAN_POINT ( 'NONE',  ( 7.869584159753955532, 10.39565510934977333, 24.50000000000000000 ) ) ;
#19230=CARTESIAN_POINT ( 'NONE',  ( -0.6060441907983137311, -20.00878639882294507, 19.00652017443069752 ) ) ;
#19232=DIRECTION ( 'NONE',  ( 0.7557495743542581579, 0.6548607339452852116, -0.000000000000000000 ) ) ;
#19234=CARTESIAN_POINT ( 'NONE',  ( 1.424502173535765914, -17.00587888132690040, 18.56793045041961321 ) ) ;
#19236=ADVANCED_FACE ( 'NONE', ( #18063 ), #20088, .F. ) ;
#19240=CARTESIAN_POINT ( 'NONE',  ( 11.67645754117907586, 12.46194352177088582, 19.58863275299554019 ) ) ;
#19241=FACE_OUTER_BOUND ( 'NONE', #3627, .T. ) ;
#19246=CARTESIAN_POINT ( 'NONE',  ( -14.80332652839583574, -8.501125445468646902, 6.041646659195333058 ) ) ;
#19247=CARTESIAN_POINT ( 'NONE',  ( -6.842536740270957374, 18.81187820119070508, 7.098451512883313441 ) ) ;
#19251=CARTESIAN_POINT ( 'NONE',  ( -18.07538971572905950, -8.601943808150396720, 18.34777357837151968 ) ) ;
#19255=ORIENTED_EDGE ( 'NONE', *, *, #12223, .T. ) ;
#19257=VECTOR ( 'NONE', #9159, 1000.000000000000000 ) ;
#19259=CARTESIAN_POINT ( 'NONE',  ( -13.23068377149358987, 10.73719040084102794, 7.632642797338977658 ) ) ;
#19265=EDGE_CURVE ( 'NONE', #17481, #1130, #638, .T. ) ;
#19266=CARTESIAN_POINT ( 'NONE',  ( 4.370315982788584463, 16.46653586241586709, 5.701226463332907279 ) ) ;
#19272=CARTESIAN_POINT ( 'NONE',  ( 14.30907656312162324, 13.99861481489062243, 7.196036389296800451 ) ) ;
#19276=CYLINDRICAL_SURFACE ( 'NONE', #2887, 9.482273699623480212 ) ;
#19279=CIRCLE ( 'NONE', #23252, 20.00000000000000000 ) ;
#19281=CARTESIAN_POINT ( 'NONE',  ( -15.35255149521179874, -7.379222211227442152, 7.557577766377196582 ) ) ;
#19284=DIRECTION ( 'NONE',  ( -0.000000000000000000, -0.000000000000000000, 1.000000000000000000 ) ) ;
#19286=CARTESIAN_POINT ( 'NONE',  ( -0.5567245496722502685, -20.01015347392404564, 6.211014596808754007 ) ) ;
#19287=AXIS2_PLACEMENT_3D ( 'NONE', #17631, #27460, #3908 ) ;
#19288=EDGE_CURVE ( 'NONE', #14448, #315, #1040, .T. ) ;
#19290=VECTOR ( 'NONE', #12434, 1000.000000000000000 ) ;
#19291=DIRECTION ( 'NONE',  ( 1.000000000000000000, 0.000000000000000000, 0.000000000000000000 ) ) ;
#19294=VERTEX_POINT ( 'NONE', #25850 ) ;
#19304=EDGE_CURVE ( 'NONE', #17232, #13976, #14315, .T. ) ;
#19310=CARTESIAN_POINT ( 'NONE',  ( 15.87456320658223241, -6.220724357885990763, 18.35718225375110180 ) ) ;
#19311=CARTESIAN_POINT ( 'NONE',  ( 16.61290147319822452, 3.916522693408248657, 18.64703902303423178 ) ) ;
#19312=DIRECTION ( 'NONE',  ( 1.000000000000000000, 0.000000000000000000, 0.000000000000000000 ) ) ;
#19316=ORIENTED_EDGE ( 'NONE', *, *, #30693, .T. ) ;
#19318=EDGE_CURVE ( 'NONE', #12217, #1853, #22786, .T. ) ;
#19319=EDGE_CURVE ( 'NONE', #4512, #6958, #6365, .T. ) ;
#19320=CARTESIAN_POINT ( 'NONE',  ( 2.703030265324084080, -12.75514121382991384, 24.50000000000000000 ) ) ;
#19321=CARTESIAN_POINT ( 'NONE',  ( -12.74366836927934798, 11.28516576207253408, 19.66989035740801839 ) ) ;
#19325=CARTESIAN_POINT ( 'NONE',  ( -9.772441304892783620, -17.47026709695451174, 18.82680253904184298 ) ) ;
#19326=CARTESIAN_POINT ( 'NONE',  ( 19.74328841314636307, 3.194145055459935101, 7.652108011868850035 ) ) ;
#19327=DIRECTION ( 'NONE',  ( -0.000000000000000000, -0.000000000000000000, 1.000000000000000000 ) ) ;
#19332=VECTOR ( 'NONE', #29420, 1000.000000000000000 ) ;
#19333=CARTESIAN_POINT ( 'NONE',  ( 15.05691039802740150, 13.16451011206821597, 20.32243167357989577 ) ) ;
#19335=ORIENTED_EDGE ( 'NONE', *, *, #20814, .T. ) ;
#19339=DIRECTION ( 'NONE',  ( -0.5406408174555974444, -0.8412535328311813165, 0.000000000000000000 ) ) ;
#19341=CARTESIAN_POINT ( 'NONE',  ( -13.89991139849285773, 7.447222512978775022, -0.6213203435596476032 ) ) ;
#19342=CARTESIAN_POINT ( 'NONE',  ( -15.52789627658390614, -6.978352780205158368, 7.156916968540300239 ) ) ;
#19345=ORIENTED_EDGE ( 'NONE', *, *, #16438, .F. ) ;
#19346=VECTOR ( 'NONE', #17375, 1000.000000000000000 ) ;
#19351=DIRECTION ( 'NONE',  ( 0.000000000000000000, 0.000000000000000000, 1.000000000000000000 ) ) ;
#19356=CARTESIAN_POINT ( 'NONE',  ( 18.73355814148580833, -7.053980495653730642, 6.672349528511551497 ) ) ;
#19361=ORIENTED_EDGE ( 'NONE', *, *, #3335, .F. ) ;
#19362=CARTESIAN_POINT ( 'NONE',  ( 5.225607896785846584, 19.32380464960333555, 5.652605728828375753 ) ) ;
#19369=ORIENTED_EDGE ( 'NONE', *, *, #12030, .F. ) ;
#19371=CIRCLE ( 'NONE', #28356, 1.000000000000010436 ) ;
#19375=EDGE_LOOP ( 'NONE', ( #9958, #15410, #8695, #26565 ) ) ;
#19376=CARTESIAN_POINT ( 'NONE',  ( -15.75094665830067697, -12.32508334119358828, 1.500000000000001332 ) ) ;
#19377=CARTESIAN_POINT ( 'NONE',  ( 6.437793815610357129, -6.974883619896809606, 21.50000000000000000 ) ) ;
#19380=CIRCLE ( 'NONE', #11932, 9.482273699623480212 ) ;
#19384=CARTESIAN_POINT ( 'NONE',  ( 19.65639872822723433, 3.693339721720553914, 7.528076282304597022 ) ) ;
#19385=EDGE_LOOP ( 'NONE', ( #4422, #24147, #9054, #622 ) ) ;
#19396=ORIENTED_EDGE ( 'NONE', *, *, #4224, .T. ) ;
#19398=CARTESIAN_POINT ( 'NONE',  ( -0.5696721008582762424, -20.00987732873323210, 19.77662771831109367 ) ) ;
#19400=CARTESIAN_POINT ( 'NONE',  ( -9.723733991145046218, -17.49730778217155702, 6.233981582756856987 ) ) ;
#19401=CARTESIAN_POINT ( 'NONE',  ( 4.641725321057754705, 16.38498716467266547, 18.54473042795394733 ) ) ;
#19402=CARTESIAN_POINT ( 'NONE',  ( 1.068432182113367768, -19.98925970413800002, 20.06253562465620632 ) ) ;
#19406=CARTESIAN_POINT ( 'NONE',  ( 1.340340228783118537, -19.95510490826381655, 19.61564845152807735 ) ) ;
#19407=CARTESIAN_POINT ( 'NONE',  ( -6.812559277181930106, 5.881244434206302607, 1.500000000000001332 ) ) ;
#19408=EDGE_LOOP ( 'NONE', ( #16986, #29990, #20713, #30566 ) ) ;
#19411=CARTESIAN_POINT ( 'NONE',  ( -17.81743587613173574, -9.123988531026229865, 5.810767894563978686 ) ) ;
#19412=CARTESIAN_POINT ( 'NONE',  ( -6.723597995833586083, 18.85470073956823356, 7.280727868105637768 ) ) ;
#19413=CARTESIAN_POINT ( 'NONE',  ( -8.840471615930058036, 1.687027447297517080, 21.50000000000000000 ) ) ;
#19415=CARTESIAN_POINT ( 'NONE',  ( -15.51812306427840937, -7.001296657735109896, 18.80699882434806369 ) ) ;
#19423=VERTEX_POINT ( 'NONE', #30376 ) ;
#19424=AXIS2_PLACEMENT_3D ( 'NONE', #4725, #2394, #17043 ) ;
#19426=CARTESIAN_POINT ( 'NONE',  ( 3.685570353517261477, -16.10136545388692397, 24.50000000000000000 ) ) ;
#19428=CARTESIAN_POINT ( 'NONE',  ( 6.184030279945252673, 19.03884152227148263, 19.77662771831109367 ) ) ;
#19435=ADVANCED_FACE ( 'NONE', ( #18526 ), #28029, .F. ) ;
#19439=CARTESIAN_POINT ( 'NONE',  ( -15.26311659977724311, -7.574663188999290142, 7.632642797338977658 ) ) ;
#19441=CARTESIAN_POINT ( 'NONE',  ( 14.70507365826912327, 13.55638513645770438, 7.626218077512938009 ) ) ;
#19442=CARTESIAN_POINT ( 'NONE',  ( 0.7070334246190017602, -17.02861022043351724, 5.653912893140659257 ) ) ;
#19451=LINE ( 'NONE', #15209, #11595 ) ;
#19452=ORIENTED_EDGE ( 'NONE', *, *, #6578, .T. ) ;
#19453=ORIENTED_EDGE ( 'NONE', *, *, #803, .F. ) ;
#19458=CARTESIAN_POINT ( 'NONE',  ( 13.01739631533118668, 10.96666867565305381, 19.33715507985239412 ) ) ;
#19460=CARTESIAN_POINT ( 'NONE',  ( -11.19021577446866900, -16.59822551944401781, 6.018569869498933578 ) ) ;
#19462=ADVANCED_FACE ( 'NONE', ( #7272 ), #14911, .F. ) ;
#19463=CARTESIAN_POINT ( 'NONE',  ( 18.55936137128098196, -7.500557692851354652, 20.19593175699879595 ) ) ;
#19468=CARTESIAN_POINT ( 'NONE',  ( 15.75996277359000075, -6.485024779738598255, 20.34789198813116329 ) ) ;
#19471=VERTEX_POINT ( 'NONE', #21617 ) ;
#19474=CARTESIAN_POINT ( 'NONE',  ( -6.157909564977937400, 15.91569265719595627, 18.56793045041961321 ) ) ;
#19475=CARTESIAN_POINT ( 'NONE',  ( -14.74940038399478581, 13.53421240139457815, 19.77662771831109367 ) ) ;
#19477=CARTESIAN_POINT ( 'NONE',  ( -7.715867830805694716, -15.23386229593460683, 19.03762469184452755 ) ) ;
#19483=CARTESIAN_POINT ( 'NONE',  ( 11.11866449908640675, -16.64592002940951332, 5.652196082367002106 ) ) ;
#19485=CIRCLE ( 'NONE', #20957, 0.7500000000000004441 ) ;
#19486=CARTESIAN_POINT ( 'NONE',  ( 9.007989464659763357, -14.44232047555455445, 6.519181285484531685 ) ) ;
#19487=ORIENTED_EDGE ( 'NONE', *, *, #12500, .F. ) ;
#19488=ORIENTED_EDGE ( 'NONE', *, *, #21231, .T. ) ;
#19489=CARTESIAN_POINT ( 'NONE',  ( 9.169883732660084164, -9.268939115642975679, 1.500000000000001332 ) ) ;
#19490=CARTESIAN_POINT ( 'NONE',  ( 10.25423333689188077, -17.17121715837755147, 6.518927109361853489 ) ) ;
#19491=FACE_BOUND ( 'NONE', #887, .T. ) ;
#19494=LINE ( 'NONE', #29008, #974 ) ;
#19496=ORIENTED_EDGE ( 'NONE', *, *, #10148, .F. ) ;
#19498=AXIS2_PLACEMENT_3D ( 'NONE', #18840, #26153, #4326 ) ;
#19501=EDGE_CURVE ( 'NONE', #24485, #21278, #5870, .T. ) ;
#19504=CARTESIAN_POINT ( 'NONE',  ( 15.45804667738991967, 12.71867858434618093, 7.176035686813569292 ) ) ;
#19505=ORIENTED_EDGE ( 'NONE', *, *, #24631, .T. ) ;
#19508=CARTESIAN_POINT ( 'NONE',  ( 16.59744209609359444, 3.993643014828355486, 18.73314399819311760 ) ) ;
#19511=VERTEX_POINT ( 'NONE', #3828 ) ;
#19512=ADVANCED_FACE ( 'NONE', ( #17704 ), #6014, .T. ) ;
#19513=DIRECTION ( 'NONE',  ( 0.000000000000000000, 0.000000000000000000, 1.000000000000000000 ) ) ;
#19519=CARTESIAN_POINT ( 'NONE',  ( 10.27641578865089933, -17.15802603149301220, 19.60917204426171878 ) ) ;
#19521=B_SPLINE_CURVE_WITH_KNOTS ( 'NONE', 3,
 ( #5616, #17768, #7791, #5141, #9986, #17303, #26835, #24625, #5460, #19490, #3259, #17144, #24321, #609, #24474, #23043, #27288, #18083 ),
 .UNSPECIFIED., .F., .F.,
 ( 4, 2, 2, 2, 2, 2, 2, 2, 4 ),
 ( 0.003174295595554316955, 0.003570702171545545815, 0.003967108747536775108, 0.004363515323528003968, 0.004759921899519232828, 0.005156328475510462556, 0.005552735051501691416, 0.005949141627492920276, 0.006345548203484149136 ),
 .UNSPECIFIED. ) ;
#19525=EDGE_LOOP ( 'NONE', ( #26224, #19223, #15533, #16231 ) ) ;
#19527=CARTESIAN_POINT ( 'NONE',  ( -12.86767874445213877, -1.850092897552710225, 1.500000000000001332 ) ) ;
#19529=CARTESIAN_POINT ( 'NONE',  ( -14.81512577538152442, 13.43580467474268758, 18.72886616302735163 ) ) ;
#19533=CARTESIAN_POINT ( 'NONE',  ( -1.000000000000008438, 13.00000000000001421, 1.500000000000001332 ) ) ;
#19535=CARTESIAN_POINT ( 'NONE',  ( 0.4269445148198162121, -2.969464325642846347, 24.50000000000000000 ) ) ;
#19536=ORIENTED_EDGE ( 'NONE', *, *, #13572, .T. ) ;
#19538=ORIENTED_EDGE ( 'NONE', *, *, #8981, .T. ) ;
#19539=DIRECTION ( 'NONE',  ( 0.000000000000000000, 0.000000000000000000, 1.000000000000000000 ) ) ;
#19540=DIRECTION ( 'NONE',  ( -0.000000000000000000, -0.000000000000000000, 1.000000000000000000 ) ) ;
#19541=VERTEX_POINT ( 'NONE', #1186 ) ;
#19542=VERTEX_POINT ( 'NONE', #15051 ) ;
#19544=CIRCLE ( 'NONE', #4601, 9.482273699623480212 ) ;
#19545=ORIENTED_EDGE ( 'NONE', *, *, #5839, .F. ) ;
#19551=CARTESIAN_POINT ( 'NONE',  ( 4.819993392704754243, 16.32915940662073595, 18.72771030977187579 ) ) ;
#19554=DIRECTION ( 'NONE',  ( 1.000000000000000000, 0.000000000000000000, 0.000000000000000000 ) ) ;
#19555=DIRECTION ( 'NONE',  ( 1.000000000000000000, 0.000000000000000000, 0.000000000000000000 ) ) ;
#19559=CARTESIAN_POINT ( 'NONE',  ( -10.62374177707235035, -16.96647932868177122, 20.34789198813115263 ) ) ;
#19560=CARTESIAN_POINT ( 'NONE',  ( -14.96594037876678307, -8.187306180225535357, 5.749491821935610147 ) ) ;
#19561=CARTESIAN_POINT ( 'NONE',  ( -6.803558837019166639, 18.82611028990652358, 6.131018562779544823 ) ) ;
#19562=VECTOR ( 'NONE', #20495, 1000.000000000000000 ) ;
#19565=CIRCLE ( 'NONE', #3633, 0.7499999999999997780 ) ;
#19566=CARTESIAN_POINT ( 'NONE',  ( -15.55662731361435114, -6.910399801605404235, 19.00652017443069752 ) ) ;
#19569=ORIENTED_EDGE ( 'NONE', *, *, #25406, .T. ) ;
#19571=CARTESIAN_POINT ( 'NONE',  ( -5.125804696664928883, 19.33206434738277579, 18.84056766331481825 ) ) ;
#19572=CARTESIAN_POINT ( 'NONE',  ( -12.70761245252103677, 11.32417831140434039, 6.641371103590088865 ) ) ;
#19573=CARTESIAN_POINT ( 'NONE',  ( -0.1027882698832301017, -17.02358378464768762, 7.156916968540298463 ) ) ;
#19579=DIRECTION ( 'NONE',  ( -0.000000000000000000, -0.000000000000000000, -1.000000000000000000 ) ) ;
#19580=DIRECTION ( 'NONE',  ( 0.000000000000000000, 0.000000000000000000, 1.000000000000000000 ) ) ;
#19584=DIRECTION ( 'NONE',  ( -1.000000000000000000, 0.000000000000000000, 0.000000000000000000 ) ) ;
#19589=ORIENTED_EDGE ( 'NONE', *, *, #7466, .F. ) ;
#19593=CARTESIAN_POINT ( 'NONE',  ( 0.7453234696411443760, -17.02803278171227674, 5.651989602109218858 ) ) ;
#19595=DIRECTION ( 'NONE',  ( 1.000000000000000000, 0.000000000000000000, 0.000000000000000000 ) ) ;
#19597=CARTESIAN_POINT ( 'NONE',  ( 0.000000000000000000, 0.000000000000000000, 21.50000000000000000 ) ) ;
#19604=VECTOR ( 'NONE', #7962, 1000.000000000000000 ) ;
#19609=CARTESIAN_POINT ( 'NONE',  ( 15.48724201788533605, 12.68311944884417919, 18.90679857307105749 ) ) ;
#19610=CARTESIAN_POINT ( 'NONE',  ( -9.147715168420965881, -14.36154699054607420, 5.940635272151477686 ) ) ;
#19611=ORIENTED_EDGE ( 'NONE', *, *, #21099, .F. ) ;
#19613=CARTESIAN_POINT ( 'NONE',  ( 16.74328840634221649, 3.194145055459935101, 20.34789198813115263 ) ) ;
#19620=CARTESIAN_POINT ( 'NONE',  ( -6.587417658830998946, 18.90298706665744177, 18.56793045041961321 ) ) ;
#19621=CARTESIAN_POINT ( 'NONE',  ( -12.72607405277288350, 11.30422146305940423, 19.11611934778430921 ) ) ;
#19622=CARTESIAN_POINT ( 'NONE',  ( -10.45807895166739243, -17.06883091098138649, 18.34838970509067479 ) ) ;
#19626=CARTESIAN_POINT ( 'NONE',  ( -16.99246856547862450, 1.423159825038152970, 5.678370764302467677 ) ) ;
#19628=DIRECTION ( 'NONE',  ( 0.000000000000000000, 0.000000000000000000, 1.000000000000000000 ) ) ;
#19634=CARTESIAN_POINT ( 'NONE',  ( 18.33599632111990374, -7.986941774664180649, 20.34789198813115263 ) ) ;
#19635=FACE_OUTER_BOUND ( 'NONE', #14770, .T. ) ;
#19636=CARTESIAN_POINT ( 'NONE',  ( 6.437683520590171682, -6.962021646281551845, 1.500000000000001332 ) ) ;
#19639=B_SPLINE_CURVE_WITH_KNOTS ( 'NONE', 3,
 ( #16892, #3161, #12685, #14851, #22178, #10330, #19844, #29367, #17508, #27028, #26410, #5036, #21705, #345, #19384, #14691, #4516, #19326 ),
 .UNSPECIFIED., .F., .F.,
 ( 4, 2, 2, 2, 2, 2, 2, 2, 4 ),
 ( 0.000000000000000000, 0.0003967869494442895651, 0.0007935738988885791302, 0.001190360848332868695, 0.001587147797777158260, 0.001983934747221447609, 0.002380721696665737391, 0.002777508646110027173, 0.003174295595554316521 ),
 .UNSPECIFIED. ) ;
#19643=DIRECTION ( 'NONE',  ( -0.000000000000000000, -0.000000000000000000, -1.000000000000000000 ) ) ;
#19644=CARTESIAN_POINT ( 'NONE',  ( 19.77267785325472005, 3.123260753354264452, 5.653912893140659257 ) ) ;
#19646=EDGE_CURVE ( 'NONE', #7775, #18617, #11836, .T. ) ;
#19647=CARTESIAN_POINT ( 'NONE',  ( 13.00026995858111611, 10.98778251907842574, 6.420335371522007506 ) ) ;
#19649=CARTESIAN_POINT ( 'NONE',  ( 15.94288127717319981, -6.058927977062421810, 7.603368798681074736 ) ) ;
#19653=DIRECTION ( 'NONE',  ( 1.000000000000000000, 0.000000000000000000, 0.000000000000000000 ) ) ;
#19659=CARTESIAN_POINT ( 'NONE',  ( -12.72536390617885260, -2.839914339433650348, 24.50000000000000000 ) ) ;
#19665=EDGE_CURVE ( 'NONE', #17265, #21024, #22315, .T. ) ;
#19666=CARTESIAN_POINT ( 'NONE',  ( -15.97321056478111245, 12.06495093120146578, 19.58863275299554019 ) ) ;
#19667=CARTESIAN_POINT ( 'NONE',  ( -3.662523238938586001, -12.47340865698848056, 1.500000000000001332 ) ) ;
#19669=ORIENTED_EDGE ( 'NONE', *, *, #985, .T. ) ;
#19672=EDGE_CURVE ( 'NONE', #2092, #13119, #25957, .T. ) ;
#19680=DIRECTION ( 'NONE',  ( 0.000000000000000000, 0.000000000000000000, -1.000000000000000000 ) ) ;
#19682=CARTESIAN_POINT ( 'NONE',  ( -4.163336342344337027E-14, 1.387778780781445676E-14, 24.50000000000000000 ) ) ;
#19683=ORIENTED_EDGE ( 'NONE', *, *, #11839, .F. ) ;
#19690=CARTESIAN_POINT ( 'NONE',  ( 1.000000000000008438, 19.97498435543819184, 24.50000000000000000 ) ) ;
#19694=DIRECTION ( 'NONE',  ( 0.6548607339452782172, -0.7557495743542642641, 0.000000000000000000 ) ) ;
#19697=CARTESIAN_POINT ( 'NONE',  ( 11.80555446153501897, -11.55276080277260320, 1.500000000000000000 ) ) ;
#19700=CARTESIAN_POINT ( 'NONE',  ( -11.35999944890270363, -16.46057145267185007, 6.781503518395074259 ) ) ;
#19705=ORIENTED_EDGE ( 'NONE', *, *, #8836, .T. ) ;
#19708=CARTESIAN_POINT ( 'NONE',  ( -15.10044507415839199, -7.916284227987608446, 7.643931100913408550 ) ) ;
#19709=CARTESIAN_POINT ( 'NONE',  ( -6.485206790418930112, 15.79815780198025621, 6.892848776733236704 ) ) ;
#19710=AXIS2_PLACEMENT_3D ( 'NONE', #3052, #19580, #29253 ) ;
#19712=CARTESIAN_POINT ( 'NONE',  ( -18.45239215198389715, -7.760673075470068127, 19.00652017443069752 ) ) ;
#19714=LINE ( 'NONE', #1009, #10618 ) ;
#19717=LINE ( 'NONE', #28627, #20411 ) ;
#19723=CARTESIAN_POINT ( 'NONE',  ( 16.18315216712441895, -5.452792103149284308, 19.08844262864049313 ) ) ;
#19727=CARTESIAN_POINT ( 'NONE',  ( 4.467866064779364876, 16.43745301482979215, 18.44501272782439827 ) ) ;
#19739=CARTESIAN_POINT ( 'NONE',  ( -18.24419300814587075, -8.237927942618478383, 5.749228751562096562 ) ) ;
#19740=CARTESIAN_POINT ( 'NONE',  ( 12.24063095261064404, 4.490763173670002217, 1.500000000000001332 ) ) ;
#19744=CYLINDRICAL_SURFACE ( 'NONE', #14328, 9.482273699623480212 ) ;
#19748=ORIENTED_EDGE ( 'NONE', *, *, #8281, .T. ) ;
#19750=CARTESIAN_POINT ( 'NONE',  ( 2.094186647214743235, -9.248129367672072831, 21.50000000000000000 ) ) ;
#19756=AXIS2_PLACEMENT_3D ( 'NONE', #6777, #11320, #6176 ) ;
#19760=CARTESIAN_POINT ( 'NONE',  ( 12.98391214946238037, 11.00790965981589231, 19.66989035740801839 ) ) ;
#19762=CARTESIAN_POINT ( 'NONE',  ( -19.71764211798356570, 3.454211555243455578, 6.974106381145714018 ) ) ;
#19765=CARTESIAN_POINT ( 'NONE',  ( 8.480328572437745294, -4.608906612435629491, 1.500000000000001332 ) ) ;
#19767=DIRECTION ( 'NONE',  ( 1.000000000000000000, 0.000000000000000000, 0.000000000000000000 ) ) ;
#19768=ORIENTED_EDGE ( 'NONE', *, *, #2285, .T. ) ;
#19771=VERTEX_POINT ( 'NONE', #25509 ) ;
#19773=DIRECTION ( 'NONE',  ( 0.2817325568414296710, -0.9594929736144973687, 0.000000000000000000 ) ) ;
#19774=CARTESIAN_POINT ( 'NONE',  ( 19.58625041283695367, 4.133291823432031720, 6.995624166085161910 ) ) ;
#19775=CARTESIAN_POINT ( 'NONE',  ( -12.70761245252103500, 11.32417831140434217, 19.33715507985239412 ) ) ;
#19783=CARTESIAN_POINT ( 'NONE',  ( -17.01654212181477277, 1.203597991882926710, 5.749491821935610147 ) ) ;
#19785=AXIS2_PLACEMENT_3D ( 'NONE', #20770, #23110, #6595 ) ;
#19787=CARTESIAN_POINT ( 'NONE',  ( -9.824744466605366711, -8.513189541288717521, 24.50000000000000000 ) ) ;
#19788=AXIS2_PLACEMENT_3D ( 'NONE', #27168, #24504, #3149 ) ;
#19789=LINE ( 'NONE', #17299, #27359 ) ;
#19790=ORIENTED_EDGE ( 'NONE', *, *, #18495, .T. ) ;
#19792=CARTESIAN_POINT ( 'NONE',  ( 18.22972622987023783, -8.227512309863355355, 20.32243167357988511 ) ) ;
#19794=CARTESIAN_POINT ( 'NONE',  ( -5.544451646083597751, 16.11829163520482666, 7.652108011868850035 ) ) ;
#19795=ORIENTED_EDGE ( 'NONE', *, *, #6690, .F. ) ;
#19797=AXIS2_PLACEMENT_3D ( 'NONE', #21955, #585, #10105 ) ;
#19799=AXIS2_PLACEMENT_3D ( 'NONE', #15671, #3209, #6169 ) ;
#19801=ORIENTED_EDGE ( 'NONE', *, *, #17374, .T. ) ;
#19803=CARTESIAN_POINT ( 'NONE',  ( -9.752241470433741455, -17.46128603886499420, 19.85730954408916915 ) ) ;
#19804=CARTESIAN_POINT ( 'NONE',  ( -17.92585835919032178, -8.870080556897411483, 18.37545668562167478 ) ) ;
#19806=CARTESIAN_POINT ( 'NONE',  ( 4.049916833591940879, 16.55712665779027049, 7.652108011868850923 ) ) ;
#19808=CARTESIAN_POINT ( 'NONE',  ( 13.01739631533119201, 10.96666867565305736, 6.641371103590088865 ) ) ;
#19811=CARTESIAN_POINT ( 'NONE',  ( 18.73275811567551230, -7.056106374802665115, 6.782048567692550378 ) ) ;
#19813=DIRECTION ( 'NONE',  ( 0.000000000000000000, 0.000000000000000000, -1.000000000000000000 ) ) ;
#19814=DIRECTION ( 'NONE',  ( -0.8412535328311884220, -0.5406408174555862312, 0.000000000000000000 ) ) ;
#19817=EDGE_CURVE ( 'NONE', #13440, #29598, #30332, .T. ) ;
#19826=CARTESIAN_POINT ( 'NONE',  ( 9.252152043196039344, -14.29436518012014545, 20.05479082170252525 ) ) ;
#19830=DIRECTION ( 'NONE',  ( 1.000000000000000000, 0.000000000000000000, 0.000000000000000000 ) ) ;
#19831=CARTESIAN_POINT ( 'NONE',  ( -15.50193441389835414, 12.66492269502747980, 18.37415474056476938 ) ) ;
#19832=LINE ( 'NONE', #5491, #2356 ) ;
#19833=ADVANCED_FACE ( 'NONE', ( #4130 ), #3987, .F. ) ;
#19835=AXIS2_PLACEMENT_3D ( 'NONE', #3261, #930, #5619 ) ;
#19836=DIRECTION ( 'NONE',  ( 1.000000000000000000, 0.000000000000000000, 0.000000000000000000 ) ) ;
#19837=LINE ( 'NONE', #29361, #26798 ) ;
#19841=AXIS2_PLACEMENT_3D ( 'NONE', #26863, #20136, #25278 ) ;
#19842=CARTESIAN_POINT ( 'NONE',  ( 3.474270935886293987, -15.38174572367601911, 24.50000000000000000 ) ) ;
#19843=CARTESIAN_POINT ( 'NONE',  ( 16.74250988114178185, 3.198928528055117848, 5.652196082368483587 ) ) ;
#19844=CARTESIAN_POINT ( 'NONE',  ( 19.58194293052863344, 4.068188588073704537, 6.149077423860700442 ) ) ;
#19852=ORIENTED_EDGE ( 'NONE', *, *, #24823, .F. ) ;
#19854=CARTESIAN_POINT ( 'NONE',  ( -9.752241470433746784, -17.46128603886497643, 7.161525567826878103 ) ) ;
#19856=CARTESIAN_POINT ( 'NONE',  ( 0.7070334246189989846, -17.02861022043351724, 18.34969686940295830 ) ) ;
#19859=EDGE_CURVE ( 'NONE', #1364, #1974, #7389, .T. ) ;
#19865=AXIS2_PLACEMENT_3D ( 'NONE', #19182, #28705, #20073 ) ;
#19867=EDGE_CURVE ( 'NONE', #27304, #17934, #12077, .T. ) ;
#19869=CARTESIAN_POINT ( 'NONE',  ( 19.74251403343738076, 3.198927889078825970, 18.34798005863226678 ) ) ;
#19870=CARTESIAN_POINT ( 'NONE',  ( 12.20938699334972277, 11.90340052968385365, 20.32367522806703874 ) ) ;
#19872=EDGE_CURVE ( 'NONE', #28669, #1242, #12532, .T. ) ;
#19874=EDGE_CURVE ( 'NONE', #4888, #4677, #16335, .T. ) ;
#19875=CARTESIAN_POINT ( 'NONE',  ( -9.321015140911132590, -14.24452793913984294, 19.77662771831109367 ) ) ;
#19877=CARTESIAN_POINT ( 'NONE',  ( -6.300265418930216299, 19.00075578015505684, 5.704143890883081269 ) ) ;
#19884=ORIENTED_EDGE ( 'NONE', *, *, #2506, .F. ) ;
#19886=DIRECTION ( 'NONE',  ( -0.9594929736144975907, 0.2817325568414293380, 0.000000000000000000 ) ) ;
#19887=CARTESIAN_POINT ( 'NONE',  ( 0.000000000000000000, 0.000000000000000000, 21.50000000000000000 ) ) ;
#19888=CARTESIAN_POINT ( 'NONE',  ( -12.81506474335657586, 11.20733750501348069, 6.111214848085761986 ) ) ;
#19889=FACE_OUTER_BOUND ( 'NONE', #15416, .T. ) ;
#19890=ORIENTED_EDGE ( 'NONE', *, *, #11520, .F. ) ;
#19893=DIRECTION ( 'NONE',  ( 0.000000000000000000, 0.000000000000000000, 1.000000000000000000 ) ) ;
#19896=CARTESIAN_POINT ( 'NONE',  ( 4.370315982788584463, 16.46653586241585998, 18.39701043959520987 ) ) ;
#19897=ADVANCED_FACE ( 'NONE', ( #2866 ), #5208, .F. ) ;
#19898=CIRCLE ( 'NONE', #23866, 0.7499999999999997780 ) ;
#19900=ADVANCED_FACE ( 'NONE', ( #65 ), #16741, .F. ) ;
#19909=CARTESIAN_POINT ( 'NONE',  ( -9.824744466605366711, -8.513189541288717521, 1.500000000000001332 ) ) ;
#19910=VERTEX_POINT ( 'NONE', #9723 ) ;
#19911=DIRECTION ( 'NONE',  ( -0.4154150130018973153, -0.9096319953545134451, 0.000000000000000000 ) ) ;
#19912=CARTESIAN_POINT ( 'NONE',  ( 12.44591117081739817, 11.64178973126078454, 20.34789198813115974 ) ) ;
#19916=CARTESIAN_POINT ( 'NONE',  ( -7.028330626922778990, 10.93629592680536788, 1.500000000000001332 ) ) ;
#19917=CARTESIAN_POINT ( 'NONE',  ( -12.72536390617885260, -2.839914339433650348, 1.500000000000001332 ) ) ;
#19921=DIRECTION ( 'NONE',  ( 1.000000000000000000, 0.000000000000000000, 0.000000000000000000 ) ) ;
#19924=VERTEX_POINT ( 'NONE', #22355 ) ;
#19930=CIRCLE ( 'NONE', #10965, 1.000000000000000888 ) ;
#19931=CARTESIAN_POINT ( 'NONE',  ( 15.55295851173241672, 12.60248606922869463, 19.45164628100866722 ) ) ;
#19933=ORIENTED_EDGE ( 'NONE', *, *, #27507, .T. ) ;
#19935=CARTESIAN_POINT ( 'NONE',  ( 17.96688762764193470, -8.785985129476816979, 6.144783687052512988 ) ) ;
#19936=CARTESIAN_POINT ( 'NONE',  ( 18.33792385446292528, -7.982495159855863776, 5.652196082369963293 ) ) ;
#19940=CARTESIAN_POINT ( 'NONE',  ( -16.82262805705560993, 2.599658093694372063, 19.66962785902261501 ) ) ;
#19941=ORIENTED_EDGE ( 'NONE', *, *, #19288, .T. ) ;
#19945=CARTESIAN_POINT ( 'NONE',  ( -13.38159811102998376, 10.55828946469181773, 18.34798005862930736 ) ) ;
#19949=DIRECTION ( 'NONE',  ( 0.000000000000000000, 0.000000000000000000, 1.000000000000000000 ) ) ;
#19951=VERTEX_POINT ( 'NONE', #5513 ) ;
#19952=CARTESIAN_POINT ( 'NONE',  ( 11.08678458728283189, -16.66722406908985477, 5.651989602109218858 ) ) ;
#19954=DIRECTION ( 'NONE',  ( 1.000000000000000000, 0.000000000000000000, 0.000000000000000000 ) ) ;
#19956=VERTEX_POINT ( 'NONE', #27357 ) ;
#19958=DIRECTION ( 'NONE',  ( -0.7557495743542581579, -0.6548607339452852116, 0.000000000000000000 ) ) ;
#19962=VECTOR ( 'NONE', #6685, 1000.000000000000000 ) ;
#19967=CARTESIAN_POINT ( 'NONE',  ( -9.635826629942098265, -17.52571954072712757, 19.21940439362673203 ) ) ;
#19968=CARTESIAN_POINT ( 'NONE',  ( 12.30438418247799426, 11.79938075381829421, 5.652605728828373977 ) ) ;
#19969=CARTESIAN_POINT ( 'NONE',  ( 19.89137488457043901, 2.247671665613723668, 6.310736198168394928 ) ) ;
#19971=DIRECTION ( 'NONE',  ( -0.000000000000000000, -0.000000000000000000, 1.000000000000000000 ) ) ;
#19976=CARTESIAN_POINT ( 'NONE',  ( 3.338654329031698342, 16.73860904129764648, 5.951255046771932733 ) ) ;
#19981=AXIS2_PLACEMENT_3D ( 'NONE', #5414, #29275, #17423 ) ;
#19983=CARTESIAN_POINT ( 'NONE',  ( 9.402326492558371385, -14.20083561530969263, 20.19668224736330941 ) ) ;
#19987=CARTESIAN_POINT ( 'NONE',  ( -14.01100295375883498, 9.765235586930179679, 19.36813350477385143 ) ) ;
#19992=CARTESIAN_POINT ( 'NONE',  ( 0.000000000000000000, 0.000000000000000000, 21.50000000000000000 ) ) ;
#19995=DIRECTION ( 'NONE',  ( 1.000000000000000000, 0.000000000000000000, 0.000000000000000000 ) ) ;
#20001=LINE ( 'NONE', #27183, #6245 ) ;
#20010=CIRCLE ( 'NONE', #13550, 9.482273699623480212 ) ;
#20013=CARTESIAN_POINT ( 'NONE',  ( -9.824744466605366711, -8.513189541288717521, 1.500000000000001332 ) ) ;
#20014=CARTESIAN_POINT ( 'NONE',  ( -10.73812863781237681, -16.87327681817511404, 7.626647697317578078 ) ) ;
#20015=CARTESIAN_POINT ( 'NONE',  ( 19.91398265452213678, -1.852915226174634444, 1.500000000000001332 ) ) ;
#20017=ORIENTED_EDGE ( 'NONE', *, *, #27745, .F. ) ;
#20019=CARTESIAN_POINT ( 'NONE',  ( -11.36561296172221169, -16.47845303048202936, 19.22654678686458141 ) ) ;
#20020=CARTESIAN_POINT ( 'NONE',  ( -17.67332396526446203, -9.400239829055445639, 7.196036389296800451 ) ) ;
#20022=CARTESIAN_POINT ( 'NONE',  ( 11.30587609449920272, -16.51930395566529697, 5.678370764302467677 ) ) ;
#20023=EDGE_CURVE ( 'NONE', #25701, #27848, #12546, .T. ) ;
#20024=EDGE_CURVE ( 'NONE', #23909, #23911, #20820, .T. ) ;
#20026=CARTESIAN_POINT ( 'NONE',  ( -5.738360882150002062, -7.548823014270625187, 1.500000000000001332 ) ) ;
#20032=CARTESIAN_POINT ( 'NONE',  ( -14.83674576813424473, 13.43848929326658315, 6.018569869498933578 ) ) ;
#20039=CARTESIAN_POINT ( 'NONE',  ( 5.624045005368206063, 19.21181948662073324, 18.39701043959520987 ) ) ;
#20045=ADVANCED_FACE ( 'NONE', ( #11575 ), #30591, .F. ) ;
#20049=ORIENTED_EDGE ( 'NONE', *, *, #6301, .F. ) ;
#20050=CARTESIAN_POINT ( 'NONE',  ( 1.687027447297431371, 8.840471615930075799, 21.50000000000000000 ) ) ;
#20060=ORIENTED_EDGE ( 'NONE', *, *, #30578, .T. ) ;
#20065=CARTESIAN_POINT ( 'NONE',  ( 4.308942857043136954, 19.53031007734546165, 6.788986777570708675 ) ) ;
#20073=DIRECTION ( 'NONE',  ( -1.000000000000000000, 0.000000000000000000, 0.000000000000000000 ) ) ;
#20075=EDGE_CURVE ( 'NONE', #28626, #4819, #8943, .T. ) ;
#20077=EDGE_CURVE ( 'NONE', #19924, #9077, #904, .T. ) ;
#20080=VECTOR ( 'NONE', #11587, 1000.000000000000000 ) ;
#20081=CYLINDRICAL_SURFACE ( 'NONE', #26250, 0.7500000000000006661 ) ;
#20084=ORIENTED_EDGE ( 'NONE', *, *, #5186, .F. ) ;
#20087=ORIENTED_EDGE ( 'NONE', *, *, #23639, .F. ) ;
#20088=CYLINDRICAL_SURFACE ( 'NONE', #387, 9.482273699623480212 ) ;
#20089=VERTEX_POINT ( 'NONE', #11125 ) ;
#20090=EDGE_CURVE ( 'NONE', #321, #25215, #6736, .T. ) ;
#20093=B_SPLINE_SURFACE_WITH_KNOTS ( 'NONE', 3, 1, ( 
 ( #14435, #26124 ),
 ( #16927, #9745 ),
 ( #24400, #19259 ),
 ( #3044, #5230 ),
 ( #12245, #14588 ),
 ( #12564, #2739 ),
 ( #538, #24090 ),
 ( #21444, #2429 ),
 ( #29089, #7574 ),
 ( #22057, #2893 ),
 ( #692, #10060 ),
 ( #28629, #4755 ),
 ( #4917, #28782 ),
 ( #26446, #17077 ),
 ( #24241, #19572 ),
 ( #3196, #13027 ),
 ( #22215, #22515 ),
 ( #1164, #12718 ),
 ( #25021, #13174 ),
 ( #6149, #19888 ),
 ( #20032, #29553 ),
 ( #17863, #10673 ),
 ( #851, #24877 ),
 ( #29875, #8041 ),
 ( #10837, #8187 ),
 ( #3513, #27380 ),
 ( #5847, #17693 ),
 ( #15655, #1014 ),
 ( #29242, #10210 ),
 ( #5687, #15504 ),
 ( #27210, #18017 ) ),
 .UNSPECIFIED., .F., .F., .F.,
 ( 4, 3, 3, 3, 3, 3, 3, 3, 3, 3, 4 ),
 ( 2, 2 ),
 ( 0.000000000000000000, 0.05425176834609633791, 0.1085332949128352958, 0.1623767749169382768, 0.2157504826133063158, 0.2688657508888171455, 0.3218907763505476360, 0.3749548578363336993, 0.4282048033836242107, 0.4818374082110501444, 0.4999999999131655715 ),
 ( 0.000000000000000000, 1.000000000000000000 ),
 .UNSPECIFIED. ) ;
#20094=CARTESIAN_POINT ( 'NONE',  ( 19.76051936388920893, 3.198927888044585721, 5.652196082364320695 ) ) ;
#20095=CARTESIAN_POINT ( 'NONE',  ( -15.21204208253569057, 13.01227270423824400, 18.36582235739946611 ) ) ;
#20097=CIRCLE ( 'NONE', #14113, 0.7499999999999997780 ) ;
#20098=CARTESIAN_POINT ( 'NONE',  ( -7.759781818727209846, -15.20954222608248863, 19.79423548914561692 ) ) ;
#20101=CARTESIAN_POINT ( 'NONE',  ( -9.372686588603338365, -14.20906563287599056, 6.385774490351135313 ) ) ;
#20102=CARTESIAN_POINT ( 'NONE',  ( -4.163336342344337027E-14, 1.387778780781445676E-14, 1.500000000000000000 ) ) ;
#20103=ORIENTED_EDGE ( 'NONE', *, *, #27340, .T. ) ;
#20108=VERTEX_POINT ( 'NONE', #16551 ) ;
#20110=CARTESIAN_POINT ( 'NONE',  ( 17.92140030663550831, -8.878400182913011918, 19.60917204426169036 ) ) ;
#20112=CARTESIAN_POINT ( 'NONE',  ( -5.292761969338719119, 19.30549167878804084, 5.940635272151477686 ) ) ;
#20115=CYLINDRICAL_SURFACE ( 'NONE', #17150, 0.7499999999999997780 ) ;
#20116=CARTESIAN_POINT ( 'NONE',  ( 6.067212148875111843, 19.05774739413747909, 6.033082186765050814 ) ) ;
#20118=CARTESIAN_POINT ( 'NONE',  ( -10.51100883930070040, -17.01524884273342764, 18.34798005863226678 ) ) ;
#20120=CARTESIAN_POINT ( 'NONE',  ( 16.80963242778063815, 2.754998275627142945, 7.557577766377196582 ) ) ;
#20121=ORIENTED_EDGE ( 'NONE', *, *, #30168, .F. ) ;
#20122=CARTESIAN_POINT ( 'NONE',  ( 12.38084545251366997, 11.71426794001388494, 5.651989602109218858 ) ) ;
#20124=VERTEX_POINT ( 'NONE', #9850 ) ;
#20130=CARTESIAN_POINT ( 'NONE',  ( 5.303644920943712648, 19.30240823413181062, 7.652108011868850035 ) ) ;
#20134=CARTESIAN_POINT ( 'NONE',  ( -5.524309650260714299, 7.706848733601010082, 1.500000000000001332 ) ) ;
#20135=FACE_OUTER_BOUND ( 'NONE', #6060, .T. ) ;
#20136=DIRECTION ( 'NONE',  ( -0.000000000000000000, -0.000000000000000000, 1.000000000000000000 ) ) ;
#20137=EDGE_LOOP ( 'NONE', ( #6765, #23334, #20159, #23052 ) ) ;
#20139=CARTESIAN_POINT ( 'NONE',  ( -15.45532977000708641, 12.72198496171736259, 18.35718225375110180 ) ) ;
#20140=CARTESIAN_POINT ( 'NONE',  ( 9.860909914091287476, -13.90333503830274609, 7.652108011868850923 ) ) ;
#20142=EDGE_LOOP ( 'NONE', ( #7067, #10612, #7115, #24640 ) ) ;
#20145=FACE_OUTER_BOUND ( 'NONE', #9946, .T. ) ;
#20146=CARTESIAN_POINT ( 'NONE',  ( -14.76380438154529173, 13.49194818783279004, 18.84056766331481825 ) ) ;
#20148=DIRECTION ( 'NONE',  ( -0.000000000000000000, -0.000000000000000000, 1.000000000000000000 ) ) ;
#20154=LINE ( 'NONE', #22182, #11973 ) ;
#20157=CARTESIAN_POINT ( 'NONE',  ( 5.130938270761610021, -7.974144905643801629, 13.00000000000000178 ) ) ;
#20159=ORIENTED_EDGE ( 'NONE', *, *, #17163, .F. ) ;
#20164=DIRECTION ( 'NONE',  ( 1.000000000000000000, 0.000000000000000000, 0.000000000000000000 ) ) ;
#20165=CARTESIAN_POINT ( 'NONE',  ( -11.03465445395215028, -16.68068344163646799, 5.849008070840543638 ) ) ;
#20166=CARTESIAN_POINT ( 'NONE',  ( 3.662523238938590442, -12.47340865698848056, 24.50000000000000000 ) ) ;
#20167=CARTESIAN_POINT ( 'NONE',  ( 0.7836603910024315667, -17.02734626465442602, 5.652196082364321583 ) ) ;
#20170=CARTESIAN_POINT ( 'NONE',  ( -14.97070905019798737, -8.177877011708877930, 7.559636331181775581 ) ) ;
#20172=CARTESIAN_POINT ( 'NONE',  ( 11.47892014274828298, -16.39977715623751564, 7.559636331181775581 ) ) ;
#20175=ORIENTED_EDGE ( 'NONE', *, *, #7084, .F. ) ;
#20179=DIRECTION ( 'NONE',  ( -0.000000000000000000, -0.000000000000000000, 1.000000000000000000 ) ) ;
#20180=CARTESIAN_POINT ( 'NONE',  ( -11.40980092660686829, 6.310027164379044429, 24.50000000000000000 ) ) ;
#20184=CARTESIAN_POINT ( 'NONE',  ( -11.35443157991640994, -16.48616348260577524, 6.420335371522007506 ) ) ;
#20185=ORIENTED_EDGE ( 'NONE', *, *, #1425, .T. ) ;
#20194=EDGE_CURVE ( 'NONE', #2008, #21638, #19193, .T. ) ;
#20196=LINE ( 'NONE', #17883, #8329 ) ;
#20202=CIRCLE ( 'NONE', #17224, 0.7500000000000006661 ) ;
#20204=LINE ( 'NONE', #22545, #4357 ) ;
#20209=CARTESIAN_POINT ( 'NONE',  ( -8.770223337697045096, -14.60814232176939953, 18.37259980046033903 ) ) ;
#20212=ORIENTED_EDGE ( 'NONE', *, *, #17222, .F. ) ;
#20215=CARTESIAN_POINT ( 'NONE',  ( -1.246245039005721811, -2.728895986063572643, 24.50000000000000000 ) ) ;
#20220=CARTESIAN_POINT ( 'NONE',  ( -4.622016212553093695, -12.19167610014704906, 1.500000000000001332 ) ) ;
#20221=B_SPLINE_CURVE_WITH_KNOTS ( 'NONE', 3,
 ( #22617, #5785, #13442, #3600, #27466, #6089, #20724, #25272, #22770, #1266, #30105, #8597, #18104, #10620, #11082, #1576, #20580, #12969 ),
 .UNSPECIFIED., .F., .F.,
 ( 4, 2, 2, 2, 2, 2, 2, 2, 4 ),
 ( 0.003174295595554306113, 0.003570702171545539743, 0.003967108747536773374, 0.004363515323528007438, 0.004759921899519240635, 0.005156328475510474699, 0.005552735051501708763, 0.005949141627492942827, 0.006345548203484176024 ),
 .UNSPECIFIED. ) ;
#20222=CARTESIAN_POINT ( 'NONE',  ( 9.007989464659727830, -14.44232047555457932, 19.21496526180055042 ) ) ;
#20226=LINE ( 'NONE', #17735, #811 ) ;
#20228=CARTESIAN_POINT ( 'NONE',  ( 16.74328841314637017, 3.194145055459935545, 7.652108011868850923 ) ) ;
#20231=CARTESIAN_POINT ( 'NONE',  ( -9.185733585337896301, 2.352830851074203533, 13.00000000000000178 ) ) ;
#20235=DIRECTION ( 'NONE',  ( -0.000000000000000000, -0.000000000000000000, 1.000000000000000000 ) ) ;
#20237=ORIENTED_EDGE ( 'NONE', *, *, #10926, .T. ) ;
#20239=CARTESIAN_POINT ( 'NONE',  ( -6.737892368765498574, 18.83108299337146718, 19.96797677718664232 ) ) ;
#20242=CARTESIAN_POINT ( 'NONE',  ( 19.57381806301095750, 4.191719245021451101, 6.782048567692550378 ) ) ;
#20248=CARTESIAN_POINT ( 'NONE',  ( -19.93127403599639536, 1.860458748833900833, 18.56793045041961321 ) ) ;
#20249=DIRECTION ( 'NONE',  ( 0.000000000000000000, 1.000000000000000000, 0.000000000000000000 ) ) ;
#20250=ORIENTED_EDGE ( 'NONE', *, *, #8613, .T. ) ;
#20253=CARTESIAN_POINT ( 'NONE',  ( 3.262081159835028110, 16.75658363658047278, 18.73314399819312115 ) ) ;
#20262=CARTESIAN_POINT ( 'NONE',  ( -4.661329110590012981, 16.37253524622245138, 7.080843742048788414 ) ) ;
#20263=ORIENTED_EDGE ( 'NONE', *, *, #24631, .F. ) ;
#20264=DIRECTION ( 'NONE',  ( -0.000000000000000000, -0.000000000000000000, 1.000000000000000000 ) ) ;
#20265=AXIS2_PLACEMENT_3D ( 'NONE', #17178, #5022, #12359 ) ;
#20266=CARTESIAN_POINT ( 'NONE',  ( -12.71197447203570263, 11.31946111510421105, 6.519181285484529909 ) ) ;
#20272=CARTESIAN_POINT ( 'NONE',  ( 19.81199842303381686, 2.865066961627992903, 5.701226463332907279 ) ) ;
#20273=VERTEX_POINT ( 'NONE', #26860 ) ;
#20275=CARTESIAN_POINT ( 'NONE',  ( 15.25015041412930827, 12.96756205105604920, 5.796888747622817029 ) ) ;
#20277=VERTEX_POINT ( 'NONE', #637 ) ;
#20278=CARTESIAN_POINT ( 'NONE',  ( 8.606594496258196614, 4.390207617113981442, 1.500000000000001332 ) ) ;
#20279=EDGE_CURVE ( 'NONE', #27751, #13589, #14284, .T. ) ;
#20283=ORIENTED_EDGE ( 'NONE', *, *, #20800, .F. ) ;
#20286=CARTESIAN_POINT ( 'NONE',  ( 3.064607854149375754, 16.80099270350295626, 6.782048567692550378 ) ) ;
#20288=CARTESIAN_POINT ( 'NONE',  ( -2.662523238938575343, -12.47340865698848056, 1.500000000000001332 ) ) ;
#20291=CARTESIAN_POINT ( 'NONE',  ( 10.51735345234056673, -17.03234025559531162, 18.63641924841378028 ) ) ;
#20292=CARTESIAN_POINT ( 'NONE',  ( 19.89739966441223018, 2.193321724558643382, 19.45164628100866722 ) ) ;
#20296=CARTESIAN_POINT ( 'NONE',  ( 15.48289691231203768, -7.082479268569366049, 6.018569869498933578 ) ) ;
#20297=CARTESIAN_POINT ( 'NONE',  ( -13.71804704112739870, 10.14464636835443301, 20.19593175699879595 ) ) ;
#20301=AXIS2_PLACEMENT_3D ( 'NONE', #13045, #22394, #27076 ) ;
#20303=CARTESIAN_POINT ( 'NONE',  ( 10.65056555575646158, -13.34799940469215329, 6.329955581934033404 ) ) ;
#20307=CARTESIAN_POINT ( 'NONE',  ( 0.000000000000000000, 0.000000000000000000, 21.50000000000000000 ) ) ;
#20308=CARTESIAN_POINT ( 'NONE',  ( 9.860909914091285700, -13.90333503830274253, 20.34789198813115263 ) ) ;
#20314=ADVANCED_FACE ( 'NONE', ( #26024 ), #9645, .T. ) ;
#20321=CARTESIAN_POINT ( 'NONE',  ( -6.778663211761418061, 6.630478080506979843, 21.50000000000000000 ) ) ;
#20332=CARTESIAN_POINT ( 'NONE',  ( -16.83567995169601161, 2.524450606648186213, 7.156916968540302904 ) ) ;
#20336=CARTESIAN_POINT ( 'NONE',  ( -4.953525029859956241, 16.29343450967639129, 5.848946451764560628 ) ) ;
#20337=CARTESIAN_POINT ( 'NONE',  ( 10.69412491129097909, -13.31565357151865570, 6.560937769032974209 ) ) ;
#20340=AXIS2_PLACEMENT_3D ( 'NONE', #29886, #8526, #8971 ) ;
#20341=ORIENTED_EDGE ( 'NONE', *, *, #10148, .T. ) ;
#20342=ORIENTED_EDGE ( 'NONE', *, *, #16050, .F. ) ;
#20346=FACE_OUTER_BOUND ( 'NONE', #10510, .T. ) ;
#20348=CARTESIAN_POINT ( 'NONE',  ( 3.790840891945185476, 16.62820496708805962, 5.653604225791662330 ) ) ;
#20351=CARTESIAN_POINT ( 'NONE',  ( -8.738547258790619665, -14.62818084867463853, 5.670038381137163519 ) ) ;
#20354=B_SPLINE_SURFACE_WITH_KNOTS ( 'NONE', 3, 1, ( 
 ( #1586, #3931 ),
 ( #16077, #6565 ),
 ( #27938, #25737 ),
 ( #13889, #4368 ),
 ( #13452, #30421 ),
 ( #9058, #27629 ),
 ( #18266, #25593 ),
 ( #11096, #8913 ),
 ( #20590, #1881 ),
 ( #27477, #22783 ),
 ( #6704, #4213 ),
 ( #18576, #23076 ),
 ( #30267, #15608 ),
 ( #8746, #13736 ),
 ( #22934, #11404 ),
 ( #1724, #23391 ),
 ( #20451, #30115 ),
 ( #27788, #2028 ),
 ( #20896, #6415 ),
 ( #3769, #15933 ),
 ( #28082, #25447 ),
 ( #16219, #18436 ),
 ( #29970, #11553 ),
 ( #21043, #30565 ),
 ( #17969, #25126 ),
 ( #18114, #4070 ),
 ( #1437, #13288 ),
 ( #10952, #8608 ),
 ( #11239, #6253 ),
 ( #13598, #15764 ),
 ( #25285, #16985 ) ),
 .UNSPECIFIED., .F., .F., .F.,
 ( 4, 3, 3, 3, 3, 3, 3, 3, 3, 3, 4 ),
 ( 2, 2 ),
 ( 0.4999999998345684982, 0.5360336730431939367, 0.5907651151589012883, 0.6456034593241830599, 0.6998270958050434309, 0.7529536536315937223, 0.8052385063053260073, 0.8575343587103997356, 0.9106564858195042023, 0.9648414833209685293, 1.000000006602610236 ),
 ( 0.000000000000000000, 1.000000000000000000 ),
 .UNSPECIFIED. ) ;
#20357=LINE ( 'NONE', #22674, #10851 ) ;
#20362=CARTESIAN_POINT ( 'NONE',  ( -10.45807895166738710, -17.06883091098137939, 5.652605728828375753 ) ) ;
#20366=CARTESIAN_POINT ( 'NONE',  ( 12.76513901715592958, 11.27219777357495900, 20.14907003336613300 ) ) ;
#20369=DIRECTION ( 'NONE',  ( 1.000000000000000000, 0.000000000000000000, 0.000000000000000000 ) ) ;
#20371=DIRECTION ( 'NONE',  ( 0.9594929736144992560, 0.2817325568414232317, 0.000000000000000000 ) ) ;
#20375=CARTESIAN_POINT ( 'NONE',  ( -8.550548372801090480, -14.74545326687210434, 20.34789198813115263 ) ) ;
#20382=FACE_OUTER_BOUND ( 'NONE', #25907, .T. ) ;
#20383=ORIENTED_EDGE ( 'NONE', *, *, #26164, .F. ) ;
#20387=CARTESIAN_POINT ( 'NONE',  ( 9.752055262432786975, -13.97602916343634583, 20.34789198813115974 ) ) ;
#20388=ADVANCED_FACE ( 'NONE', ( #28675 ), #3671, .T. ) ;
#20391=EDGE_CURVE ( 'NONE', #13705, #4512, #8230, .T. ) ;
#20392=CARTESIAN_POINT ( 'NONE',  ( -11.03614041005516277, -16.67970391259860108, 20.14992337338001960 ) ) ;
#20395=CARTESIAN_POINT ( 'NONE',  ( 15.53710936759972050, 12.59357901975564076, 6.518927109361845496 ) ) ;
#20396=DIRECTION ( 'NONE',  ( -0.1423148382732850048, -0.9898214418809327952, 0.000000000000000000 ) ) ;
#20397=ORIENTED_EDGE ( 'NONE', *, *, #7062, .T. ) ;
#20398=CARTESIAN_POINT ( 'NONE',  ( -4.604861147461548398, 16.38721654675212847, 19.60617949693493500 ) ) ;
#20400=CARTESIAN_POINT ( 'NONE',  ( -15.16517293421789070, -7.781889191988407894, 7.652108011868850923 ) ) ;
#20403=DIRECTION ( 'NONE',  ( 0.2817325568414296710, -0.9594929736144973687, 0.000000000000000000 ) ) ;
#20404=CARTESIAN_POINT ( 'NONE',  ( 16.61290147319823518, 3.916522693408249545, 5.951255046771932733 ) ) ;
#20406=CARTESIAN_POINT ( 'NONE',  ( 1.795304038745368480, -16.98367057141060599, 6.783738457429051572 ) ) ;
#20408=FACE_OUTER_BOUND ( 'NONE', #26238, .T. ) ;
#20411=VECTOR ( 'NONE', #10058, 1000.000000000000000 ) ;
#20412=CARTESIAN_POINT ( 'NONE',  ( 10.68026781623521515, -13.32599531033823759, 19.14333282897057842 ) ) ;
#20418=ADVANCED_FACE ( 'NONE', ( #22418 ), #20081, .F. ) ;
#20421=CARTESIAN_POINT ( 'NONE',  ( -5.031059497539948744, 16.27164807758200027, 5.796888747622817029 ) ) ;
#20423=DIRECTION ( 'NONE',  ( -1.000000000000000000, 0.000000000000000000, 0.000000000000000000 ) ) ;
#20424=CARTESIAN_POINT ( 'NONE',  ( -13.20835299067310409, 10.76336294910227664, 7.626437579292365321 ) ) ;
#20425=CARTESIAN_POINT ( 'NONE',  ( -7.730328572437709767, 4.608906612435681005, 21.50000000000000000 ) ) ;
#20430=CARTESIAN_POINT ( 'NONE',  ( 14.84329864647545172, 13.43104200419766059, 5.652605728828373977 ) ) ;
#20434=ADVANCED_FACE ( 'NONE', ( #25065 ), #8149, .T. ) ;
#20435=FACE_OUTER_BOUND ( 'NONE', #2734, .T. ) ;
#20437=EDGE_CURVE ( 'NONE', #18506, #160, #24248, .T. ) ;
#20438=ORIENTED_EDGE ( 'NONE', *, *, #18721, .T. ) ;
#20439=EDGE_CURVE ( 'NONE', #950, #30524, #20840, .T. ) ;
#20440=CARTESIAN_POINT ( 'NONE',  ( 4.523123428450326777, 19.49994255397358600, 6.041646659195333058 ) ) ;
#20441=CARTESIAN_POINT ( 'NONE',  ( 6.812559277181973627, -5.881244434206257310, 21.50000000000000000 ) ) ;
#20442=CARTESIAN_POINT ( 'NONE',  ( 13.00999358272542850, -0.8602714556717643291, 24.50000000000000000 ) ) ;
#20444=CARTESIAN_POINT ( 'NONE',  ( 9.096230214749073895, -14.38931669386024836, 18.90679857307105749 ) ) ;
#20446=VERTEX_POINT ( 'NONE', #8696 ) ;
#20448=CARTESIAN_POINT ( 'NONE',  ( 18.16954353748349860, -8.401983848419027012, 7.557577766377196582 ) ) ;
#20449=AXIS2_PLACEMENT_3D ( 'NONE', #26966, #27260, #24918 ) ;
#20451=CARTESIAN_POINT ( 'NONE',  ( 4.318335944327693632, 19.54627428603377126, 19.47783254395485031 ) ) ;
#20455=EDGE_CURVE ( 'NONE', #18622, #10066, #8428, .T. ) ;
#20458=CARTESIAN_POINT ( 'NONE',  ( 12.88533868980070096, 11.12831076047921286, 7.267659094423561505 ) ) ;
#20464=CARTESIAN_POINT ( 'NONE',  ( 2.959227181723801170, -8.499586724479446076, 21.50000000000000000 ) ) ;
#20467=ORIENTED_EDGE ( 'NONE', *, *, #29469, .T. ) ;
#20472=CARTESIAN_POINT ( 'NONE',  ( 1.438332125858173605, -8.884323311075778662, 21.50000000000000000 ) ) ;
#20474=CARTESIAN_POINT ( 'NONE',  ( -9.454746441592954298, 0.7220001660363462026, 13.00000000000000178 ) ) ;
#20480=CARTESIAN_POINT ( 'NONE',  ( 1.694955473231256393, -16.99033591619069483, 7.098451512883313441 ) ) ;
#20481=CARTESIAN_POINT ( 'NONE',  ( -16.89565484002363149, 2.154541803859437277, 7.526951045817045660 ) ) ;
#20483=EDGE_CURVE ( 'NONE', #15490, #28288, #11805, .T. ) ;
#20484=ADVANCED_FACE ( 'NONE', ( #28488 ), #1175, .T. ) ;
#20488=CARTESIAN_POINT ( 'NONE',  ( 9.454746441592959627, -0.7220001660362782570, 1.500000000000001332 ) ) ;
#20489=CIRCLE ( 'NONE', #8553, 0.7500000000000024425 ) ;
#20491=VERTEX_POINT ( 'NONE', #1174 ) ;
#20495=DIRECTION ( 'NONE',  ( 0.000000000000000000, 0.000000000000000000, -1.000000000000000000 ) ) ;
#20497=DIRECTION ( 'NONE',  ( 1.000000000000000000, 0.000000000000000000, 0.000000000000000000 ) ) ;
#20499=CARTESIAN_POINT ( 'NONE',  ( -8.744978663125429819, -14.62407600317563627, 7.632642797338977658 ) ) ;
#20500=ORIENTED_EDGE ( 'NONE', *, *, #39, .T. ) ;
#20503=CARTESIAN_POINT ( 'NONE',  ( 19.74328841314634886, 3.194145055459934213, 20.34789198813115263 ) ) ;
#20511=CARTESIAN_POINT ( 'NONE',  ( 12.00212711895368933, 12.12705342280389154, 20.24143955528809258 ) ) ;
#20513=CARTESIAN_POINT ( 'NONE',  ( 1.164358918501135598, -19.96629823696781614, 18.73377938172348323 ) ) ;
#20515=CYLINDRICAL_SURFACE ( 'NONE', #12764, 1.000000000000004441 ) ;
#20517=EDGE_CURVE ( 'NONE', #21638, #1882, #17239, .T. ) ;
#20518=DIRECTION ( 'NONE',  ( 0.000000000000000000, 0.000000000000000000, 1.000000000000000000 ) ) ;
#20520=CARTESIAN_POINT ( 'NONE',  ( -5.393256883115301825, -14.81828060999315433, 1.500000000000001332 ) ) ;
#20525=LINE ( 'NONE', #22701, #14933 ) ;
#20532=CARTESIAN_POINT ( 'NONE',  ( 9.755266891893601411, -13.97392213636465108, 18.34727598691067740 ) ) ;
#20534=ORIENTED_EDGE ( 'NONE', *, *, #26162, .T. ) ;
#20535=CARTESIAN_POINT ( 'NONE',  ( -10.73477556097085994, -16.87541441043898161, 18.37250658438899009 ) ) ;
#20545=CARTESIAN_POINT ( 'NONE',  ( -16.81483160676717503, 2.643882879105585726, 19.47784884541372108 ) ) ;
#20549=CARTESIAN_POINT ( 'NONE',  ( 16.73141127408300477, 3.267558643021993170, 7.652108011868850035 ) ) ;
#20550=CARTESIAN_POINT ( 'NONE',  ( -10.52692686119061882, -17.02631563033163076, 20.34789198813115263 ) ) ;
#20552=CARTESIAN_POINT ( 'NONE',  ( -9.288552932799431616, -14.26664216879983371, 6.143977687428008316 ) ) ;
#20554=ORIENTED_EDGE ( 'NONE', *, *, #6330, .F. ) ;
#20561=CARTESIAN_POINT ( 'NONE',  ( -15.73693831436012402, 12.34332084443491873, 5.853797745100182581 ) ) ;
#20562=AXIS2_PLACEMENT_3D ( 'NONE', #27338, #18124, #19995 ) ;
#20563=B_SPLINE_CURVE_WITH_KNOTS ( 'NONE', 3,
 ( #25077, #8562, #24607, #27582, #10729, #13396, #10428, #3876, #5740, #11045, #29302, #13085, #20239, #29763, #5595, #22574, #8405, #17450 ),
 .UNSPECIFIED., .F., .F.,
 ( 4, 2, 2, 2, 2, 2, 2, 2, 4 ),
 ( 0.000000000000000000, 0.0003967869494442892398, 0.0007935738988885784797, 0.001190360848332867611, 0.001587147797777156959, 0.001983934747221446308, 0.002380721696665735222, 0.002777508646110024570, 0.003174295595554313919 ),
 .UNSPECIFIED. ) ;
#20564=CARTESIAN_POINT ( 'NONE',  ( -5.090837523869514492, 19.35983187734362687, 7.080843742048788414 ) ) ;
#20566=CYLINDRICAL_SURFACE ( 'NONE', #2619, 9.482273699623480212 ) ;
#20567=CARTESIAN_POINT ( 'NONE',  ( 0.1262659238204208167, 8.999114229549594057, 1.500000000000001332 ) ) ;
#20569=DIRECTION ( 'NONE',  ( 1.000000000000000000, 0.000000000000000000, 0.000000000000000000 ) ) ;
#20572=ORIENTED_EDGE ( 'NONE', *, *, #11520, .T. ) ;
#20577=CARTESIAN_POINT ( 'NONE',  ( 3.436936369909017408, 16.71530215271316422, 7.441806358946449151 ) ) ;
#20580=CARTESIAN_POINT ( 'NONE',  ( 5.419676874198347427, 19.25213680916389691, 18.34726407865098707 ) ) ;
#20584=CARTESIAN_POINT ( 'NONE',  ( 16.87674189766844890, 2.217009531549523960, 19.56050940960062690 ) ) ;
#20588=CARTESIAN_POINT ( 'NONE',  ( 18.02181326450768140, -8.714141732420078057, 6.018569869498933578 ) ) ;
#20589=CARTESIAN_POINT ( 'NONE',  ( -15.35797660355606453, 12.83915183367558299, 5.652196082364323360 ) ) ;
#20590=CARTESIAN_POINT ( 'NONE',  ( 4.592382419210019329, 19.48389062382846504, 18.64703902303423178 ) ) ;
#20594=CARTESIAN_POINT ( 'NONE',  ( 10.69247012765649174, -13.31688477309528018, 6.588756557121050683 ) ) ;
#20595=B_SPLINE_SURFACE_WITH_KNOTS ( 'NONE', 3, 1, ( 
 ( #7404, #16913 ),
 ( #7557, #369 ),
 ( #11764, #12395 ),
 ( #2871, #2722 ),
 ( #9728, #17057 ),
 ( #23601, #23757 ),
 ( #28464, #4739 ),
 ( #21261, #26429 ),
 ( #21729, #2411 ),
 ( #26590, #24072 ),
 ( #5213, #24223 ),
 ( #29073, #5058 ),
 ( #21895, #14715 ),
 ( #30790, #7090 ),
 ( #28612, #7234 ),
 ( #524, #10047 ),
 ( #11937, #16450 ),
 ( #4591, #19240 ),
 ( #71, #14092 ),
 ( #16595, #16746 ),
 ( #14241, #9584 ),
 ( #26262, #4902 ),
 ( #14420, #23922 ),
 ( #2569, #12083 ),
 ( #28764, #3497 ),
 ( #5985, #25005 ),
 ( #29536, #22501 ),
 ( #679, #19870 ),
 ( #22652, #24859 ),
 ( #1145, #3645 ),
 ( #12551, #834 ) ),
 .UNSPECIFIED., .F., .F., .F.,
 ( 4, 3, 3, 3, 3, 3, 3, 3, 3, 3, 4 ),
 ( 2, 2 ),
 ( 0.4999999998345686647, 0.5360336730431939367, 0.5907651151589012883, 0.6456034593241830599, 0.6998270958050434309, 0.7529536536315937223, 0.8052385063053260073, 0.8575343587103997356, 0.9106564858195042023, 0.9648414833209685293, 1.000000006602610014 ),
 ( 0.000000000000000000, 1.000000000000000000 ),
 .UNSPECIFIED. ) ;
#20596=CARTESIAN_POINT ( 'NONE',  ( -4.581181804672374014, 16.39335237280001323, 19.22654678686458141 ) ) ;
#20597=CARTESIAN_POINT ( 'NONE',  ( -8.840471615930058036, 1.687027447297517080, 1.500000000000001332 ) ) ;
#20599=EDGE_CURVE ( 'NONE', #30087, #17934, #29247, .T. ) ;
#20600=FACE_OUTER_BOUND ( 'NONE', #6255, .T. ) ;
#20607=CARTESIAN_POINT ( 'NONE',  ( -19.87893182697125027, 2.354587536660440961, 7.643931100913408550 ) ) ;
#20610=ORIENTED_EDGE ( 'NONE', *, *, #23080, .T. ) ;
#20613=CARTESIAN_POINT ( 'NONE',  ( 9.590471615930072247, -1.687027447297460236, 1.500000000000001332 ) ) ;
#20614=CARTESIAN_POINT ( 'NONE',  ( -19.90131041440201187, 1.988107338454508932, 18.47531940416305929 ) ) ;
#20615=EDGE_LOOP ( 'NONE', ( #22000, #24525, #269, #7881 ) ) ;
#20618=DIRECTION ( 'NONE',  ( 0.000000000000000000, 1.000000000000000000, 0.000000000000000000 ) ) ;
#20619=EDGE_CURVE ( 'NONE', #13589, #22306, #15353, .T. ) ;
#20622=CARTESIAN_POINT ( 'NONE',  ( 4.622016212553096359, -12.19167610014704906, 1.500000000000001332 ) ) ;
#20625=CIRCLE ( 'NONE', #24584, 0.7500000000000006661 ) ;
#20627=CARTESIAN_POINT ( 'NONE',  ( 1.000541756189969433, -17.02230863066393596, 7.627891251804737927 ) ) ;
#20629=ORIENTED_EDGE ( 'NONE', *, *, #13760, .T. ) ;
#20630=EDGE_CURVE ( 'NONE', #3823, #24787, #14900, .T. ) ;
#20631=CYLINDRICAL_SURFACE ( 'NONE', #6873, 9.482273699623480212 ) ;
#20633=EDGE_CURVE ( 'NONE', #13391, #27228, #26924, .T. ) ;
#20634=CARTESIAN_POINT ( 'NONE',  ( -4.580173031741206380, 16.39361746661401043, 6.782064869129509788 ) ) ;
#20640=CARTESIAN_POINT ( 'NONE',  ( -0.5297379638125987444, -19.99304770284714650, 19.85261563089511228 ) ) ;
#20643=DIRECTION ( 'NONE',  ( 0.000000000000000000, 0.000000000000000000, 1.000000000000000000 ) ) ;
#20649=EDGE_CURVE ( 'NONE', #28858, #25523, #20913, .T. ) ;
#20654=CARTESIAN_POINT ( 'NONE',  ( 11.52514311384750911, -16.34582042812247238, 7.528076282304598799 ) ) ;
#20657=CARTESIAN_POINT ( 'NONE',  ( -8.481700458822091448, -14.78796854237962677, 5.652605728828375753 ) ) ;
#20659=ORIENTED_EDGE ( 'NONE', *, *, #983, .T. ) ;
#20661=CARTESIAN_POINT ( 'NONE',  ( 12.69001473637742983, 11.36098604102020460, 18.47056384035244037 ) ) ;
#20664=LINE ( 'NONE', #23605, #3318 ) ;
#20665=DIRECTION ( 'NONE',  ( -0.1423148382732850048, -0.9898214418809327952, 0.000000000000000000 ) ) ;
#20667=DIRECTION ( 'NONE',  ( 0.000000000000000000, 0.000000000000000000, 1.000000000000000000 ) ) ;
#20669=CARTESIAN_POINT ( 'NONE',  ( -15.35255149521179519, -7.379222211227441264, 20.25336174263950184 ) ) ;
#20678=CARTESIAN_POINT ( 'NONE',  ( 9.035144332690526525, -14.42607982873371952, 19.60617949693493856 ) ) ;
#20680=ORIENTED_EDGE ( 'NONE', *, *, #4963, .F. ) ;
#20681=CARTESIAN_POINT ( 'NONE',  ( -16.96078254943347829, 1.685604580053745361, 5.651989602109218858 ) ) ;
#20690=CARTESIAN_POINT ( 'NONE',  ( 5.687793815610356241, -6.974883619896809606, 21.50000000000000000 ) ) ;
#20694=CARTESIAN_POINT ( 'NONE',  ( -7.667077102831937552, 13.77986170986486592, 24.50000000000000000 ) ) ;
#20698=CARTESIAN_POINT ( 'NONE',  ( -13.89991139849285773, 7.447222512978775022, 24.50000000000000000 ) ) ;
#20699=CARTESIAN_POINT ( 'NONE',  ( -9.169883732660077058, -9.268939115642981008, 1.500000000000001332 ) ) ;
#20707=CARTESIAN_POINT ( 'NONE',  ( -5.905415913170756426, 19.12693415355692750, 5.653912893140659257 ) ) ;
#20710=VECTOR ( 'NONE', #24329, 1000.000000000000000 ) ;
#20713=ORIENTED_EDGE ( 'NONE', *, *, #7968, .T. ) ;
#20716=CARTESIAN_POINT ( 'NONE',  ( 5.524309650260767590, -7.706848733600972778, 21.50000000000000000 ) ) ;
#20719=CARTESIAN_POINT ( 'NONE',  ( 1.000000000000008438, 16.48749217771910125, 24.50000000000000000 ) ) ;
#20721=ORIENTED_EDGE ( 'NONE', *, *, #10693, .F. ) ;
#20723=CARTESIAN_POINT ( 'NONE',  ( -8.413215745754975217, 3.196529495465474380, 21.50000000000000000 ) ) ;
#20724=CARTESIAN_POINT ( 'NONE',  ( 6.140972302510984804, 19.03394436102036380, 19.85261563089512293 ) ) ;
#20727=CARTESIAN_POINT ( 'NONE',  ( 4.622016212553096359, -12.19167610014704906, 24.50000000000000000 ) ) ;
#20729=CARTESIAN_POINT ( 'NONE',  ( 16.76146518920503325, 3.081792779576177033, 20.34789198813115263 ) ) ;
#20730=EDGE_LOOP ( 'NONE', ( #18403, #7704, #11928, #25861 ) ) ;
#20732=CARTESIAN_POINT ( 'NONE',  ( 17.92455701194924700, -8.912206770388248600, 6.755862304746362845 ) ) ;
#20733=CARTESIAN_POINT ( 'NONE',  ( -15.93537878762121807, 12.11488692681952806, 6.233981582756856987 ) ) ;
#20734=CIRCLE ( 'NONE', #4799, 0.7500000000000015543 ) ;
#20736=VERTEX_POINT ( 'NONE', #9381 ) ;
#20741=CARTESIAN_POINT ( 'NONE',  ( -5.090837523869514492, 19.35983187734363042, 19.77662771831109367 ) ) ;
#20744=ADVANCED_FACE ( 'NONE', ( #18593 ), #30733, .F. ) ;
#20750=VECTOR ( 'NONE', #27441, 1000.000000000000227 ) ;
#20751=CARTESIAN_POINT ( 'NONE',  ( -17.04208893090348909, 0.9369385374313049519, 7.366751648393900176 ) ) ;
#20752=CARTESIAN_POINT ( 'NONE',  ( 14.32702845807336267, 13.95510847468388249, 18.73377938172349033 ) ) ;
#20753=CARTESIAN_POINT ( 'NONE',  ( 19.87632233081032496, 2.221350112303686508, 19.08232364404840453 ) ) ;
#20757=CARTESIAN_POINT ( 'NONE',  ( 15.94669506555478122, -6.049764716652520136, 5.704143890883081269 ) ) ;
#20762=CARTESIAN_POINT ( 'NONE',  ( -0.1550506074450035132, -19.99977091204053536, 7.526993102356323462 ) ) ;
#20767=DIRECTION ( 'NONE',  ( -0.000000000000000000, -0.000000000000000000, -1.000000000000000000 ) ) ;
#20770=CARTESIAN_POINT ( 'NONE',  ( 8.840471615930072247, -1.687027447297460236, 1.500000000000001332 ) ) ;
#20771=CARTESIAN_POINT ( 'NONE',  ( 1.111517487559786632, -17.01912455222412390, 7.603368798681074736 ) ) ;
#20772=CARTESIAN_POINT ( 'NONE',  ( -16.81483160676645383, 2.643882879109654915, 6.782064869129509788 ) ) ;
#20776=CARTESIAN_POINT ( 'NONE',  ( -13.37849590498012908, 10.56201291617988147, 7.652108011868850923 ) ) ;
#20777=ORIENTED_EDGE ( 'NONE', *, *, #30029, .T. ) ;
#20778=FACE_OUTER_BOUND ( 'NONE', #30704, .T. ) ;
#20779=CARTESIAN_POINT ( 'NONE',  ( -17.59781475975454157, -9.540531696329384914, 19.25672174529527325 ) ) ;
#20780=AXIS2_PLACEMENT_3D ( 'NONE', #12513, #24814, #29651 ) ;
#20781=VECTOR ( 'NONE', #28268, 1000.000000000000000 ) ;
#20784=VECTOR ( 'NONE', #14097, 1000.000000000000227 ) ;
#20786=DIRECTION ( 'NONE',  ( -0.000000000000000000, -0.000000000000000000, 1.000000000000000000 ) ) ;
#20792=CARTESIAN_POINT ( 'NONE',  ( 11.10715495309693601, -16.63223102436629830, 7.652108011868850035 ) ) ;
#20797=CYLINDRICAL_SURFACE ( 'NONE', #1991, 0.7499999999999988898 ) ;
#20800=EDGE_CURVE ( 'NONE', #13440, #1001, #30265, .T. ) ;
#20806=CARTESIAN_POINT ( 'NONE',  ( 7.724883619896791842, 5.687793815610376669, 1.500000000000001332 ) ) ;
#20814=EDGE_CURVE ( 'NONE', #1364, #21915, #29016, .T. ) ;
#20819=CARTESIAN_POINT ( 'NONE',  ( -15.55757656138296419, -6.908027829044470103, 19.66962785902261501 ) ) ;
#20820=CIRCLE ( 'NONE', #4886, 9.482273699623480212 ) ;
#20825=CARTESIAN_POINT ( 'NONE',  ( -15.55925901137641709, -6.904021205104065473, 19.66989035740801839 ) ) ;
#20827=ORIENTED_EDGE ( 'NONE', *, *, #5417, .T. ) ;
#20832=DIRECTION ( 'NONE',  ( -0.8412535328311810945, -0.5406408174555976665, 0.000000000000000000 ) ) ;
#20836=CARTESIAN_POINT ( 'NONE',  ( 17.94577521512061580, -8.869393445417760091, 19.66989035740801839 ) ) ;
#20838=DIRECTION ( 'NONE',  ( 1.000000000000000000, 0.000000000000000000, 0.000000000000000000 ) ) ;
#20839=ORIENTED_EDGE ( 'NONE', *, *, #29610, .T. ) ;
#20840=LINE ( 'NONE', #11498, #6813 ) ;
#20843=CARTESIAN_POINT ( 'NONE',  ( 15.53731853391908402, 12.59332096006128943, 6.781503518395071595 ) ) ;
#20845=VERTEX_POINT ( 'NONE', #14818 ) ;
#20848=ADVANCED_FACE ( 'NONE', ( #24165 ), #3408, .T. ) ;
#20852=CARTESIAN_POINT ( 'NONE',  ( 16.76419345870816002, 3.064929150530655733, 20.34789198813115974 ) ) ;
#20855=CARTESIAN_POINT ( 'NONE',  ( 0.2321890030833198282, -17.02978461145532307, 7.500898271101006820 ) ) ;
#20857=CYLINDRICAL_SURFACE ( 'NONE', #16736, 0.7500000000000006661 ) ;
#20858=CARTESIAN_POINT ( 'NONE',  ( -17.06629969734983021, 0.6399978984115078928, 19.47952243369110548 ) ) ;
#20859=CARTESIAN_POINT ( 'NONE',  ( -17.06456206750264215, 0.6636403356599821501, 19.58863275299554019 ) ) ;
#20861=ORIENTED_EDGE ( 'NONE', *, *, #27715, .F. ) ;
#20863=EDGE_CURVE ( 'NONE', #984, #5348, #4858, .T. ) ;
#20864=CARTESIAN_POINT ( 'NONE',  ( 9.860909911264737815, -13.90333503211346766, 20.34789198813115263 ) ) ;
#20868=ORIENTED_EDGE ( 'NONE', *, *, #5164, .F. ) ;
#20869=DIRECTION ( 'NONE',  ( 0.000000000000000000, 0.000000000000000000, -1.000000000000000000 ) ) ;
#20870=CARTESIAN_POINT ( 'NONE',  ( 7.706848733600955903, 5.524309650260792459, 13.00000000000000178 ) ) ;
#20878=CARTESIAN_POINT ( 'NONE',  ( 16.74864137134696662, 3.161078882829541747, 5.651989602109218858 ) ) ;
#20881=ORIENTED_EDGE ( 'NONE', *, *, #19318, .F. ) ;
#20885=ORIENTED_EDGE ( 'NONE', *, *, #25615, .T. ) ;
#20889=CARTESIAN_POINT ( 'NONE',  ( 9.195964344571798676, -14.32884674914071610, 18.71435384576123440 ) ) ;
#20892=CARTESIAN_POINT ( 'NONE',  ( -19.86072707285307715, 2.502642989097795478, 20.34789198813115263 ) ) ;
#20895=CARTESIAN_POINT ( 'NONE',  ( -15.94999985682713906, 12.09556989559485274, 6.995624166085161910 ) ) ;
#20896=CARTESIAN_POINT ( 'NONE',  ( 4.376647981176106761, 19.53331152111370272, 19.69140814234746273 ) ) ;
#20902=CARTESIAN_POINT ( 'NONE',  ( -5.325396069054046500, 16.18574704710536949, 20.32842677360128292 ) ) ;
#20904=AXIS2_PLACEMENT_3D ( 'NONE', #3014, #54, #11921 ) ;
#20905=CARTESIAN_POINT ( 'NONE',  ( 9.436481611552753890, 0.9307681286968855217, 21.50000000000000000 ) ) ;
#20909=CARTESIAN_POINT ( 'NONE',  ( 1.367923798957373593, -19.95316478012375683, 6.788986777570696241 ) ) ;
#20911=CARTESIAN_POINT ( 'NONE',  ( 19.87928744571102513, 2.194067154482766124, 19.47728749465736797 ) ) ;
#20913=LINE ( 'NONE', #9525, #17783 ) ;
#20915=CARTESIAN_POINT ( 'NONE',  ( 18.56338958360293745, -7.490577753534551242, 5.810767894563978686 ) ) ;
#20916=FACE_OUTER_BOUND ( 'NONE', #16479, .T. ) ;
#20922=CARTESIAN_POINT ( 'NONE',  ( 8.549050687778164459, 4.102102735472485939, 13.00000000000000178 ) ) ;
#20924=CARTESIAN_POINT ( 'NONE',  ( -16.96496224101209194, 1.652369717150044659, 7.652108011868850923 ) ) ;
#20927=DIRECTION ( 'NONE',  ( -0.000000000000000000, -0.000000000000000000, 1.000000000000000000 ) ) ;
#20929=DIRECTION ( 'NONE',  ( 1.000000000000000000, 0.000000000000000000, 0.000000000000000000 ) ) ;
#20930=CARTESIAN_POINT ( 'NONE',  ( 11.17648341053133798, -16.60731568869664443, 7.652108011868850035 ) ) ;
#20934=CYLINDRICAL_SURFACE ( 'NONE', #11981, 20.00000000000000000 ) ;
#20935=CARTESIAN_POINT ( 'NONE',  ( 16.17735844207722806, -3.336236224685152685, -0.6213203435596476032 ) ) ;
#20937=LINE ( 'NONE', #7214, #18081 ) ;
#20939=CIRCLE ( 'NONE', #20449, 9.482273699623480212 ) ;
#20943=CARTESIAN_POINT ( 'NONE',  ( 16.56213591300004850, 4.162091996074188671, 19.08844262864049313 ) ) ;
#20946=FACE_OUTER_BOUND ( 'NONE', #8700, .T. ) ;
#20952=EDGE_CURVE ( 'NONE', #12536, #29572, #12804, .T. ) ;
#20955=ADVANCED_FACE ( 'NONE', ( #15431 ), #6080, .F. ) ;
#20956=DIRECTION ( 'NONE',  ( -1.000000000000000000, 0.000000000000000000, 0.000000000000000000 ) ) ;
#20957=AXIS2_PLACEMENT_3D ( 'NONE', #6983, #4638, #14141 ) ;
#20960=CARTESIAN_POINT ( 'NONE',  ( -12.71180423606277365, 11.31964500333551271, 19.41069149716888020 ) ) ;
#20962=CARTESIAN_POINT ( 'NONE',  ( 3.190007960684840160, 16.77295862814622751, 19.85459532544248162 ) ) ;
#20965=CARTESIAN_POINT ( 'NONE',  ( -15.16517292768934055, -7.781889190071453299, 20.34789198813115263 ) ) ;
#20966=LINE ( 'NONE', #9282, #17091 ) ;
#20968=ORIENTED_EDGE ( 'NONE', *, *, #25839, .T. ) ;
#20969=LINE ( 'NONE', #28010, #16422 ) ;
#20972=CYLINDRICAL_SURFACE ( 'NONE', #24338, 1.000000000000010436 ) ;
#20975=CARTESIAN_POINT ( 'NONE',  ( -6.481689221575673621, 15.79948487156523207, 19.61324152429827450 ) ) ;
#20977=CARTESIAN_POINT ( 'NONE',  ( 6.225165711324285311, 19.02535939286849498, 6.974106381145714018 ) ) ;
#20980=CARTESIAN_POINT ( 'NONE',  ( -16.82311188420106518, 2.597149461308116081, 6.310736198168394928 ) ) ;
#20982=DIRECTION ( 'NONE',  ( 1.000000000000000000, 0.000000000000000000, 0.000000000000000000 ) ) ;
#20984=DIRECTION ( 'NONE',  ( -0.000000000000000000, -0.000000000000000000, 1.000000000000000000 ) ) ;
#20989=DIRECTION ( 'NONE',  ( 0.000000000000000000, 0.000000000000000000, 1.000000000000000000 ) ) ;
#20992=EDGE_CURVE ( 'NONE', #1147, #20089, #12959, .T. ) ;
#20993=DIRECTION ( 'NONE',  ( -0.000000000000000000, -0.000000000000000000, 1.000000000000000000 ) ) ;
#20995=CIRCLE ( 'NONE', #21489, 0.7499999999999988898 ) ;
#20997=CARTESIAN_POINT ( 'NONE',  ( 19.72466756933792453, 3.412884783584984927, 7.627891251804737927 ) ) ;
#20999=EDGE_CURVE ( 'NONE', #11391, #1364, #24272, .T. ) ;
#21000=DIRECTION ( 'NONE',  ( 1.000000000000000000, 0.000000000000000000, 0.000000000000000000 ) ) ;
#21001=CARTESIAN_POINT ( 'NONE',  ( 12.24063095261064404, 4.490763173670002217, 24.50000000000000000 ) ) ;
#21002=CARTESIAN_POINT ( 'NONE',  ( -19.96032475228487968, 1.513912977174403984, 19.58863275299554019 ) ) ;
#21006=CARTESIAN_POINT ( 'NONE',  ( -6.384540597206719958, 15.83495921350553459, 7.158811349119587497 ) ) ;
#21014=DIRECTION ( 'NONE',  ( 1.000000000000000000, 0.000000000000000000, 0.000000000000000000 ) ) ;
#21016=CARTESIAN_POINT ( 'NONE',  ( 12.43449883826692215, 11.65450130491726455, 20.34789198813115263 ) ) ;
#21018=ORIENTED_EDGE ( 'NONE', *, *, #5401, .T. ) ;
#21024=VERTEX_POINT ( 'NONE', #28206 ) ;
#21025=EDGE_CURVE ( 'NONE', #17954, #23193, #4509, .T. ) ;
#21030=DIRECTION ( 'NONE',  ( 0.000000000000000000, 0.000000000000000000, -1.000000000000000000 ) ) ;
#21031=CARTESIAN_POINT ( 'NONE',  ( 0.000000000000000000, 0.000000000000000000, 1.500000000000001332 ) ) ;
#21032=AXIS2_PLACEMENT_3D ( 'NONE', #20464, #15780, #29841 ) ;
#21034=CARTESIAN_POINT ( 'NONE',  ( -14.93131746134411308, -8.256826158467614363, 18.45571264222804331 ) ) ;
#21035=AXIS2_PLACEMENT_3D ( 'NONE', #23434, #28293, #9707 ) ;
#21038=CARTESIAN_POINT ( 'NONE',  ( 16.86769344895231271, 2.296683858978088466, 18.90679857307105749 ) ) ;
#21039=ORIENTED_EDGE ( 'NONE', *, *, #5986, .F. ) ;
#21040=CARTESIAN_POINT ( 'NONE',  ( -16.83986259902029659, 2.499865191129257092, 18.80699882434806369 ) ) ;
#21042=CARTESIAN_POINT ( 'NONE',  ( -15.49619650379777269, 12.67194488555738019, 20.32367522806703874 ) ) ;
#21043=CARTESIAN_POINT ( 'NONE',  ( 4.690664460087335286, 19.46058373524397922, 20.13759033520874908 ) ) ;
#21044=VERTEX_POINT ( 'NONE', #13577 ) ;
#21051=DIRECTION ( 'NONE',  ( 0.9594929736144992560, 0.2817325568414232317, 0.000000000000000000 ) ) ;
#21053=CARTESIAN_POINT ( 'NONE',  ( 0.4897477184365106040, -19.99444548460947146, 5.652912763329819512 ) ) ;
#21060=CARTESIAN_POINT ( 'NONE',  ( 16.11883921216213267, -5.620554474281632906, 6.041646659195333058 ) ) ;
#21070=CARTESIAN_POINT ( 'NONE',  ( -5.973959739936659297, 19.10558604466630683, 20.34789198813115263 ) ) ;
#21071=CARTESIAN_POINT ( 'NONE',  ( 7.562559277181973627, -5.881244434206257310, 1.500000000000001332 ) ) ;
#21073=CARTESIAN_POINT ( 'NONE',  ( 15.60593903839432706, -6.823719261784717993, 5.774779864094944593 ) ) ;
#21081=CIRCLE ( 'NONE', #24567, 0.7500000000000006661 ) ;
#21084=ORIENTED_EDGE ( 'NONE', *, *, #5777, .T. ) ;
#21085=DIRECTION ( 'NONE',  ( -0.000000000000000000, -0.000000000000000000, -1.000000000000000000 ) ) ;
#21088=CARTESIAN_POINT ( 'NONE',  ( -5.971396161871753705, 19.08775596758252391, 7.652108011868850035 ) ) ;
#21089=VERTEX_POINT ( 'NONE', #5439 ) ;
#21094=VERTEX_POINT ( 'NONE', #4802 ) ;
#21096=B_SPLINE_SURFACE_WITH_KNOTS ( 'NONE', 3, 1, ( 
 ( #22630, #8472 ),
 ( #1281, #11103 ),
 ( #17976, #20902 ),
 ( #15459, #4220 ),
 ( #8302, #18121 ),
 ( #27796, #6571 ),
 ( #10790, #17819 ),
 ( #27335, #27484 ),
 ( #25291, #25602 ),
 ( #6103, #15938 ),
 ( #20741, #25131 ),
 ( #22789, #16083 ),
 ( #5962, #3615 ),
 ( #3938, #10957 ),
 ( #13458, #22941 ),
 ( #29977, #20596 ),
 ( #1594, #30120 ),
 ( #8752, #4076 ),
 ( #13605, #1730 ),
 ( #11245, #8921 ),
 ( #18442, #24001 ),
 ( #2034, #12169 ),
 ( #19180, #25897 ),
 ( #2186, #11558 ),
 ( #13894, #4992 ),
 ( #23396, #16691 ),
 ( #30427, #28089 ),
 ( #9065, #30570 ),
 ( #7023, #14504 ),
 ( #26199, #9366 ),
 ( #16532, #11704 ) ),
 .UNSPECIFIED., .F., .F., .F.,
 ( 4, 3, 3, 3, 3, 3, 3, 3, 3, 3, 4 ),
 ( 2, 2 ),
 ( 0.000000000000000000, 0.05425176834609614362, 0.1085332949128348518, 0.1623767749169379715, 0.2157504826133058717, 0.2688657508888169789, 0.3218907763505471364, 0.3749548578363334772, 0.4282048033836237666, 0.4818374082110496448, 0.4999999999131651274 ),
 ( 0.000000000000000000, 1.000000000000000000 ),
 .UNSPECIFIED. ) ;
#21098=CARTESIAN_POINT ( 'NONE',  ( -0.3742200966386520222, -20.01457288233325116, 20.05479082170252525 ) ) ;
#21099=EDGE_CURVE ( 'NONE', #4518, #3697, #1671, .T. ) ;
#21101=CARTESIAN_POINT ( 'NONE',  ( -9.646222981487627024, -17.54010295177084089, 6.560937769032974209 ) ) ;
#21102=DIRECTION ( 'NONE',  ( -0.2817325568414296710, 0.9594929736144973687, -0.000000000000000000 ) ) ;
#21103=CARTESIAN_POINT ( 'NONE',  ( 1.733314906354235241, -16.98782497260185664, 19.69140814234746273 ) ) ;
#21105=CARTESIAN_POINT ( 'NONE',  ( 18.67144399175156977, -7.167977615171047923, 7.161525567826885208 ) ) ;
#21106=CARTESIAN_POINT ( 'NONE',  ( 16.56617216130305437, 4.143135851887535637, 6.329955581934031628 ) ) ;
#21109=ORIENTED_EDGE ( 'NONE', *, *, #5951, .F. ) ;
#21111=CARTESIAN_POINT ( 'NONE',  ( -15.57492749417079736, -6.866608492821396403, 19.47784884541372463 ) ) ;
#21112=CARTESIAN_POINT ( 'NONE',  ( -13.38160118231794371, 10.55829203257429860, 18.34798005863078885 ) ) ;
#21114=CARTESIAN_POINT ( 'NONE',  ( 3.089102459976073689, 16.79563822436285747, 19.61324152429827095 ) ) ;
#21115=CARTESIAN_POINT ( 'NONE',  ( -18.44536497093016436, -7.731176935556636209, 19.08232364404839743 ) ) ;
#21119=VERTEX_POINT ( 'NONE', #16668 ) ;
#21120=LINE ( 'NONE', #16005, #9972 ) ;
#21121=VECTOR ( 'NONE', #24747, 1000.000000000000000 ) ;
#21123=CYLINDRICAL_SURFACE ( 'NONE', #6431, 0.7500000000000024425 ) ;
#21125=CARTESIAN_POINT ( 'NONE',  ( 15.63062718528784956, -6.770321384568312340, 20.25336174263950184 ) ) ;
#21126=CARTESIAN_POINT ( 'NONE',  ( 4.930301257365633738, 16.29355789806661647, 7.080843742048788414 ) ) ;
#21128=ORIENTED_EDGE ( 'NONE', *, *, #7912, .F. ) ;
#21129=CARTESIAN_POINT ( 'NONE',  ( 4.373786442354534287, 16.46525014965065026, 20.29090034784956131 ) ) ;
#21130=DIRECTION ( 'NONE',  ( 0.1423148382732889461, 0.9898214418809321291, 0.000000000000000000 ) ) ;
#21136=CARTESIAN_POINT ( 'NONE',  ( -4.340342926365016396, -8.430595340551244377, 21.50000000000000000 ) ) ;
#21137=CARTESIAN_POINT ( 'NONE',  ( -15.17333614897415828, 13.03014763290140721, 7.626647697317578078 ) ) ;
#21139=CARTESIAN_POINT ( 'NONE',  ( -15.30782679199506546, -7.476958555467158263, 7.595116371587256054 ) ) ;
#21141=CARTESIAN_POINT ( 'NONE',  ( 16.81773250897601812, 2.696729702855533262, 18.47056384035244037 ) ) ;
#21142=CYLINDRICAL_SURFACE ( 'NONE', #6262, 9.482273699623480212 ) ;
#21146=EDGE_CURVE ( 'NONE', #22916, #24186, #7341, .T. ) ;
#21148=LINE ( 'NONE', #30668, #7016 ) ;
#21150=ORIENTED_EDGE ( 'NONE', *, *, #1930, .T. ) ;
#21151=CARTESIAN_POINT ( 'NONE',  ( 10.04466414020356524, -13.77914355952371928, 20.32367522806703874 ) ) ;
#21153=ORIENTED_EDGE ( 'NONE', *, *, #7895, .F. ) ;
#21154=VERTEX_POINT ( 'NONE', #21335 ) ;
#21156=CARTESIAN_POINT ( 'NONE',  ( 18.33599632111990019, -7.986941774664177096, 7.652108011868850035 ) ) ;
#21159=AXIS2_PLACEMENT_3D ( 'NONE', #7503, #28709, #24007 ) ;
#21162=ADVANCED_FACE ( 'NONE', ( #2786 ), #9649, .T. ) ;
#21163=DIRECTION ( 'NONE',  ( 0.000000000000000000, 0.000000000000000000, -1.000000000000000000 ) ) ;
#21165=ORIENTED_EDGE ( 'NONE', *, *, #1487, .F. ) ;
#21170=CIRCLE ( 'NONE', #29728, 0.7500000000000006661 ) ;
#21172=EDGE_CURVE ( 'NONE', #11969, #7300, #13339, .T. ) ;
#21175=CARTESIAN_POINT ( 'NONE',  ( -17.92585835919031823, -8.870080556897411483, 5.679672709359372185 ) ) ;
#21176=AXIS2_PLACEMENT_3D ( 'NONE', #21917, #12574, #17405 ) ;
#21177=EDGE_CURVE ( 'NONE', #1188, #22820, #15555, .T. ) ;
#21180=CARTESIAN_POINT ( 'NONE',  ( 19.88003893156456670, 2.345734461008496474, 18.80699882434806369 ) ) ;
#21182=FACE_OUTER_BOUND ( 'NONE', #9241, .T. ) ;
#21184=VECTOR ( 'NONE', #8269, 1000.000000000000000 ) ;
#21195=CARTESIAN_POINT ( 'NONE',  ( -5.380257496407077511, 19.26296000801971786, 5.849008070840540974 ) ) ;
#21197=EDGE_CURVE ( 'NONE', #6692, #2256, #22719, .T. ) ;
#21198=CARTESIAN_POINT ( 'NONE',  ( -17.04337418722500530, 0.9225192032720770374, 5.951255046771932733 ) ) ;
#21200=EDGE_CURVE ( 'NONE', #21892, #15430, #24600, .T. ) ;
#21202=ORIENTED_EDGE ( 'NONE', *, *, #15723, .T. ) ;
#21206=CARTESIAN_POINT ( 'NONE',  ( 15.81416324982726884, -6.360572704771158214, 5.652196082364320695 ) ) ;
#21212=ADVANCED_FACE ( 'NONE', ( #15082 ), #13231, .F. ) ;
#21214=CARTESIAN_POINT ( 'NONE',  ( 10.08428597779237457, -13.75408489919876587, 18.34938820207545263 ) ) ;
#21215=CARTESIAN_POINT ( 'NONE',  ( -18.40637697828373476, -7.823545570387639536, 7.156831654632813233 ) ) ;
#21216=CARTESIAN_POINT ( 'NONE',  ( -5.755751318732965416, 16.05090033862148502, 20.32367522806703874 ) ) ;
#21217=VECTOR ( 'NONE', #14918, 1000.000000000000000 ) ;
#21219=CYLINDRICAL_SURFACE ( 'NONE', #21338, 9.482273699623480212 ) ;
#21223=CARTESIAN_POINT ( 'NONE',  ( 15.39831020855742594, -7.255125275872136292, 6.385774490351132648 ) ) ;
#21228=VECTOR ( 'NONE', #19694, 1000.000000000000000 ) ;
#21229=CARTESIAN_POINT ( 'NONE',  ( -14.97070905019798026, -8.177877011708881483, 20.25542030744407640 ) ) ;
#21230=LINE ( 'NONE', #2686, #18708 ) ;
#21231=EDGE_CURVE ( 'NONE', #2392, #5492, #17296, .T. ) ;
#21233=CIRCLE ( 'NONE', #30700, 20.00000000000000000 ) ;
#21235=EDGE_LOOP ( 'NONE', ( #28577, #3194, #4479, #11540 ) ) ;
#21236=CARTESIAN_POINT ( 'NONE',  ( 1.750000000000008660, 16.48749217771910125, 24.50000000000000000 ) ) ;
#21237=CYLINDRICAL_SURFACE ( 'NONE', #26102, 0.7500000000000006661 ) ;
#21244=DIRECTION ( 'NONE',  ( -1.000000000000000000, 0.000000000000000000, 0.000000000000000000 ) ) ;
#21246=VECTOR ( 'NONE', #15233, 1000.000000000000000 ) ;
#21247=EDGE_LOOP ( 'NONE', ( #10140, #6963, #3272, #21018 ) ) ;
#21250=VERTEX_POINT ( 'NONE', #6202 ) ;
#21252=CARTESIAN_POINT ( 'NONE',  ( 0.5572578986459487682, -17.03042415120789954, 18.36582235739946611 ) ) ;
#21254=CARTESIAN_POINT ( 'NONE',  ( -9.668922248712510381, -17.52764785324846741, 6.892848776733236704 ) ) ;
#21256=CARTESIAN_POINT ( 'NONE',  ( 4.985742441158911298, 16.27537970825794389, 19.60617949693493500 ) ) ;
#21257=CARTESIAN_POINT ( 'NONE',  ( 0.8531715179115267889, -17.02613171184587770, 20.34789198813115263 ) ) ;
#21261=CARTESIAN_POINT ( 'NONE',  ( 14.45824965121216366, 13.84471048730597786, 18.56793045041961321 ) ) ;
#21262=DIRECTION ( 'NONE',  ( 1.000000000000000000, 0.000000000000000000, 0.000000000000000000 ) ) ;
#21274=CARTESIAN_POINT ( 'NONE',  ( -18.45502384974596310, -7.754294478968729365, 19.66989035740801839 ) ) ;
#21277=EDGE_CURVE ( 'NONE', #15068, #25416, #29790, .T. ) ;
#21278=VERTEX_POINT ( 'NONE', #29298 ) ;
#21279=ORIENTED_EDGE ( 'NONE', *, *, #8765, .T. ) ;
#21281=ADVANCED_FACE ( 'NONE', ( #3558 ), #8401, .F. ) ;
#21282=DIRECTION ( 'NONE',  ( -0.000000000000000000, -0.000000000000000000, 1.000000000000000000 ) ) ;
#21284=LINE ( 'NONE', #15855, #30333 ) ;
#21289=CARTESIAN_POINT ( 'NONE',  ( 17.99082164042340537, -8.777603813954270251, 19.87181966307587544 ) ) ;
#21290=CARTESIAN_POINT ( 'NONE',  ( 5.721595087358980258, 19.18273663903466542, 5.749228751562096562 ) ) ;
#21292=EDGE_LOOP ( 'NONE', ( #20121, #24622, #13395, #1027 ) ) ;
#21293=CARTESIAN_POINT ( 'NONE',  ( 5.524396280439210827, 19.24072699314231727, 20.32842677360128292 ) ) ;
#21294=VECTOR ( 'NONE', #28397, 1000.000000000000000 ) ;
#21297=DIRECTION ( 'NONE',  ( 1.000000000000000000, 0.000000000000000000, 0.000000000000000000 ) ) ;
#21299=VERTEX_POINT ( 'NONE', #10422 ) ;
#21303=AXIS2_PLACEMENT_3D ( 'NONE', #8557, #22570, #24921 ) ;
#21306=CARTESIAN_POINT ( 'NONE',  ( -18.45239215198388294, -7.760673075470066351, 6.310736198168394928 ) ) ;
#21312=CARTESIAN_POINT ( 'NONE',  ( -17.00407983531364309, 1.321870115990432248, 20.29915277494337644 ) ) ;
#21315=AXIS2_PLACEMENT_3D ( 'NONE', #150, #4374, #4682 ) ;
#21317=CARTESIAN_POINT ( 'NONE',  ( 11.63559590357233553, -16.28893981701509830, 20.13759033520874908 ) ) ;
#21320=ORIENTED_EDGE ( 'NONE', *, *, #96, .T. ) ;
#21323=ADVANCED_FACE ( 'NONE', ( #27428 ), #17594, .F. ) ;
#21326=CARTESIAN_POINT ( 'NONE',  ( 12.71820101047898532, 11.32761398983758383, 20.19668224736330941 ) ) ;
#21328=ORIENTED_EDGE ( 'NONE', *, *, #14707, .T. ) ;
#21329=B_SPLINE_CURVE_WITH_KNOTS ( 'NONE', 3,
 ( #1550, #27754, #3895, #22902, #20561, #9326, #19150, #2005, #19001, #12135, #28512, #23815, #6676, #11817, #28195, #26163, #23508, #4499 ),
 .UNSPECIFIED., .F., .F.,
 ( 4, 2, 2, 2, 2, 2, 2, 2, 4 ),
 ( 0.000000000000000000, 0.0003967869494442920588, 0.0007935738988885811902, 0.001190360848332870213, 0.001587147797777159128, 0.001983934747221448476, 0.002380721696665736957, 0.002777508646110026305, 0.003174295595554314786 ),
 .UNSPECIFIED. ) ;
#21330=CARTESIAN_POINT ( 'NONE',  ( 15.94669506555476701, -6.049764716652515695, 18.39992786714538298 ) ) ;
#21332=CARTESIAN_POINT ( 'NONE',  ( 16.55580462840119438, 4.191719245021452878, 19.47783254395485031 ) ) ;
#21333=CARTESIAN_POINT ( 'NONE',  ( -8.884323311075783991, -1.438332125858144295, 1.500000000000001332 ) ) ;
#21335=CARTESIAN_POINT ( 'NONE',  ( 6.437793815610357129, -6.974883619896809606, 1.500000000000001332 ) ) ;
#21338=AXIS2_PLACEMENT_3D ( 'NONE', #24025, #2526, #23717 ) ;
#21343=CARTESIAN_POINT ( 'NONE',  ( -0.1790877314264358866, -17.02136788083136310, 19.66962785902261501 ) ) ;
#21344=CARTESIAN_POINT ( 'NONE',  ( 1.208994807697890916, -19.98122169387826830, 7.196036389296800451 ) ) ;
#21347=CARTESIAN_POINT ( 'NONE',  ( 19.85228648261877282, 2.570616772381428383, 18.55820869691756769 ) ) ;
#21349=ORIENTED_EDGE ( 'NONE', *, *, #985, .F. ) ;
#21351=CARTESIAN_POINT ( 'NONE',  ( 9.402326492558371385, -14.20083561530969973, 7.500898271101006820 ) ) ;
#21354=CARTESIAN_POINT ( 'NONE',  ( -13.83017030316319840, 10.00185174541443978, 7.366751648393900176 ) ) ;
#21355=CARTESIAN_POINT ( 'NONE',  ( -19.91398265452221850, -1.852915226174651986, 1.500000000000001332 ) ) ;
#21356=EDGE_CURVE ( 'NONE', #23071, #24333, #11643, .T. ) ;
#21366=CIRCLE ( 'NONE', #7424, 1.000000000000010436 ) ;
#21373=EDGE_CURVE ( 'NONE', #5348, #30675, #11357, .T. ) ;
#21379=CARTESIAN_POINT ( 'NONE',  ( 16.02447511960551552, -5.858916503155154665, 5.810767894563978686 ) ) ;
#21384=CARTESIAN_POINT ( 'NONE',  ( 10.69237140622465887, -13.31695822555149178, 19.47952243369110548 ) ) ;
#21385=CARTESIAN_POINT ( 'NONE',  ( -18.10021843967230737, -8.508777197197414210, 7.652108011868850923 ) ) ;
#21389=ORIENTED_EDGE ( 'NONE', *, *, #30393, .T. ) ;
#21395=ORIENTED_EDGE ( 'NONE', *, *, #29042, .F. ) ;
#21400=CARTESIAN_POINT ( 'NONE',  ( 4.537114060968175266, 16.41705816690543784, 7.526951045817044772 ) ) ;
#21407=FACE_OUTER_BOUND ( 'NONE', #7603, .T. ) ;
#21409=CARTESIAN_POINT ( 'NONE',  ( -13.99459037269021344, 9.787106705890307623, 6.917457548096559883 ) ) ;
#21410=VERTEX_POINT ( 'NONE', #25536 ) ;
#21417=EDGE_LOOP ( 'NONE', ( #7954, #24780, #3515, #3585 ) ) ;
#21419=CARTESIAN_POINT ( 'NONE',  ( -0.4401303402703798384, -20.01320326077420830, 18.71435384576123440 ) ) ;
#21421=CARTESIAN_POINT ( 'NONE',  ( -9.648244442396759268, -17.53899143774386005, 6.672349528511551497 ) ) ;
#21423=CARTESIAN_POINT ( 'NONE',  ( 4.049916833591939103, 16.55712665779026693, 20.34789198813115263 ) ) ;
#21424=CARTESIAN_POINT ( 'NONE',  ( 0.6820093937066836753, -20.00641896168560052, 20.29915277494337644 ) ) ;
#21426=AXIS2_PLACEMENT_3D ( 'NONE', #19533, #4718, #26408 ) ;
#21427=CARTESIAN_POINT ( 'NONE',  ( 18.33599632111990019, -7.986941774664177096, 7.652108011868850035 ) ) ;
#21428=CARTESIAN_POINT ( 'NONE',  ( -4.622016212553093695, -12.19167610014704906, 1.500000000000001332 ) ) ;
#21429=CARTESIAN_POINT ( 'NONE',  ( 1.368946144808714793, -19.95309466511746166, 19.21940439362674624 ) ) ;
#21432=B_SPLINE_CURVE_WITH_KNOTS ( 'NONE', 3,
 ( #24981, #12684, #8156, #17659, #27177, #29839, #5808, #15000, #3008, #24363, #13142, #10328, #22634, #17349, #17981, #27490, #12526, #12987, #15305, #19843 ),
 .UNSPECIFIED., .F., .F.,
 ( 4, 2, 2, 2, 2, 2, 2, 2, 2, 4 ),
 ( 0.000000000000000000, 0.06249999999999968081, 0.1249999999999993616, 0.1874999999999990286, 0.2187499999999989453, 0.2499999999999988343, 0.3124999999999991118, 0.3749999999999992784, 0.4374999999999995559, 0.4999999999999997780 ),
 .UNSPECIFIED. ) ;
#21434=CARTESIAN_POINT ( 'NONE',  ( -14.70205207497230582, -8.690259054815006934, 6.560937769032974209 ) ) ;
#21444=CARTESIAN_POINT ( 'NONE',  ( -14.88094288956370548, 13.38957456607570506, 7.359006845440219102 ) ) ;
#21448=DIRECTION ( 'NONE',  ( 1.000000000000000000, 0.000000000000000000, 0.000000000000000000 ) ) ;
#21449=CARTESIAN_POINT ( 'NONE',  ( 5.730668117466259481, 19.18033075515274888, 7.557577766377196582 ) ) ;
#21451=CARTESIAN_POINT ( 'NONE',  ( 5.913643690471324987, 19.12442985200254597, 20.12545155307891065 ) ) ;
#21457=VECTOR ( 'NONE', #19232, 1000.000000000000000 ) ;
#21462=CARTESIAN_POINT ( 'NONE',  ( -15.43012792948217538, -7.204331193346492412, 7.429667576816606278 ) ) ;
#21463=DIRECTION ( 'NONE',  ( 1.000000000000000000, 0.000000000000000000, 0.000000000000000000 ) ) ;
#21465=CARTESIAN_POINT ( 'NONE',  ( 0.3440795696225480427, -17.03036400190297783, 5.749228751562096562 ) ) ;
#21467=DIRECTION ( 'NONE',  ( -0.000000000000000000, -0.000000000000000000, 1.000000000000000000 ) ) ;
#21468=CARTESIAN_POINT ( 'NONE',  ( -17.06646200723452722, 0.6378183210065171416, 19.25672174529527325 ) ) ;
#21472=CARTESIAN_POINT ( 'NONE',  ( 1.195154792889395967, 9.406652940105990623, 1.500000000000001332 ) ) ;
#21475=CARTESIAN_POINT ( 'NONE',  ( 4.512576344050351018, 19.48449473338812510, 19.96797677718664232 ) ) ;
#21478=ORIENTED_EDGE ( 'NONE', *, *, #16438, .T. ) ;
#21481=CARTESIAN_POINT ( 'NONE',  ( -8.647361814388510481, -14.68561526379591164, 7.652108011868850035 ) ) ;
#21483=CARTESIAN_POINT ( 'NONE',  ( 18.41347767057966678, -7.852385608265396222, 18.35718225375110180 ) ) ;
#21484=CARTESIAN_POINT ( 'NONE',  ( -15.97539537256530195, 12.03273630363204205, 19.48477075383299706 ) ) ;
#21487=CARTESIAN_POINT ( 'NONE',  ( 15.39831020856429866, -7.255125275858175904, 19.08155846658118904 ) ) ;
#21488=ORIENTED_EDGE ( 'NONE', *, *, #24067, .T. ) ;
#21489=AXIS2_PLACEMENT_3D ( 'NONE', #14170, #7009, #16519 ) ;
#21495=CARTESIAN_POINT ( 'NONE',  ( -8.079801766074020009, -15.02755831366980566, 18.50655187082627862 ) ) ;
#21500=CARTESIAN_POINT ( 'NONE',  ( -16.81500952837178531, 2.642855143025228504, 19.22654678686458141 ) ) ;
#21502=DIRECTION ( 'NONE',  ( 0.000000000000000000, 0.000000000000000000, 1.000000000000000000 ) ) ;
#21507=VECTOR ( 'NONE', #28578, 1000.000000000000000 ) ;
#21509=CARTESIAN_POINT ( 'NONE',  ( 6.187077094091595342, 11.47693674426096599, 24.50000000000000000 ) ) ;
#21510=CARTESIAN_POINT ( 'NONE',  ( -15.49859937938256138, -7.047316568033163087, 7.267659094423556176 ) ) ;
#21513=ORIENTED_EDGE ( 'NONE', *, *, #9431, .F. ) ;
#21515=LINE ( 'NONE', #9521, #20710 ) ;
#21517=EDGE_CURVE ( 'NONE', #10764, #1242, #13543, .T. ) ;
#21520=CARTESIAN_POINT ( 'NONE',  ( 12.91703683527121704, 11.08965543756653460, 6.111214848085761986 ) ) ;
#21521=EDGE_LOOP ( 'NONE', ( #14968, #21395, #28423, #18972 ) ) ;
#21522=CARTESIAN_POINT ( 'NONE',  ( -4.163336342344337027E-14, 1.387778780781445676E-14, 24.50000000000000000 ) ) ;
#21528=CIRCLE ( 'NONE', #8110, 9.482273699623480212 ) ;
#21531=EDGE_CURVE ( 'NONE', #24029, #1292, #6655, .T. ) ;
#21537=ORIENTED_EDGE ( 'NONE', *, *, #3065, .F. ) ;
#21539=ADVANCED_FACE ( 'NONE', ( #14599 ), #19276, .F. ) ;
#21547=CARTESIAN_POINT ( 'NONE',  ( 4.894722408976176276, 16.30505022501959900, 7.156916968540298463 ) ) ;
#21550=CARTESIAN_POINT ( 'NONE',  ( -11.82521593960875528, 5.400395169024524655, 24.50000000000000000 ) ) ;
#21551=CIRCLE ( 'NONE', #14090, 1.000000000000008660 ) ;
#21558=CARTESIAN_POINT ( 'NONE',  ( 15.41296542101254552, 5.939519782021115191, 24.50000000000000000 ) ) ;
#21562=AXIS2_PLACEMENT_3D ( 'NONE', #18020, #27531, #23738 ) ;
#21563=ORIENTED_EDGE ( 'NONE', *, *, #13948, .T. ) ;
#21569=CARTESIAN_POINT ( 'NONE',  ( 0.3440795696225442679, -17.03036400190298139, 18.44501272782439827 ) ) ;
#21571=CARTESIAN_POINT ( 'NONE',  ( -9.661386603328285361, -17.53179420831165558, 6.447548852708279377 ) ) ;
#21573=CARTESIAN_POINT ( 'NONE',  ( 5.016036949087476771, 16.26541432804313914, 19.41069149716887310 ) ) ;
#21574=CARTESIAN_POINT ( 'NONE',  ( 0.9359619706472936951, -17.02419289499718147, 18.35718225375110180 ) ) ;
#21575=EDGE_LOOP ( 'NONE', ( #277, #23370, #8666, #9354, #21279, #312, #9329, #22928, #1093, #22157, #10089, #23281, #21583, #5269, #19884, #6546, #30838, #11682, #29957, #9205, #9305, #11053, #9893, #11537, #1211, #7491, #12724, #14927, #9783, #11977, #9708, #5478, #12380, #5433, #10887, #8366, #11406, #1935, #10331, #28833, #5161, #9471, #8501, #24801, #28787, #17509, #6731, #30195, #10334, #19195, #6928, #12066, #6100, #21978, #10880, #24848, #27461, #23192, #17200, #9495, #24862, #2289, #14267, #12098, #11665, #20342, #3731, #16821, #5703, #25719, #18152, #10215, #2077, #27853, #23077, #6240, #11760 ) ) ;
#21577=CARTESIAN_POINT ( 'NONE',  ( 18.53505294460179798, -7.514422089582853737, 5.779535427900761135 ) ) ;
#21580=CARTESIAN_POINT ( 'NONE',  ( 1.236176367852860780, -19.96182836857062171, 19.85730954408918336 ) ) ;
#21583=ORIENTED_EDGE ( 'NONE', *, *, #1556, .T. ) ;
#21584=B_SPLINE_CURVE_WITH_KNOTS ( 'NONE', 3,
 ( #14185, #25454, #23087, #1732, #16085, #25604, #4221, #5463, #24477, #2501, #14964, #12170, #21668, #151, #9988, #760 ),
 .UNSPECIFIED., .F., .F.,
 ( 4, 2, 2, 2, 2, 2, 2, 4 ),
 ( 0.4999999999999994449, 0.6249999999999996669, 0.6874999999999997780, 0.7187499999999995559, 0.7499999999999994449, 0.8124999999999995559, 0.8749999999999997780, 1.000000000000000000 ),
 .UNSPECIFIED. ) ;
#21588=CARTESIAN_POINT ( 'NONE',  ( -6.878634932266923130, 18.79866186728735400, 6.995624166085161910 ) ) ;
#21589=DIRECTION ( 'NONE',  ( 1.000000000000000000, 0.000000000000000000, 0.000000000000000000 ) ) ;
#21596=CARTESIAN_POINT ( 'NONE',  ( -5.846240454020372290, 19.12690956503887918, 20.34789198813115618 ) ) ;
#21598=CARTESIAN_POINT ( 'NONE',  ( 11.53007546964076191, -16.34234030559854034, 18.47531940416306639 ) ) ;
#21599=ORIENTED_EDGE ( 'NONE', *, *, #11278, .F. ) ;
#21601=CARTESIAN_POINT ( 'NONE',  ( 15.59193442375634753, -6.853442328767824776, 18.49267272388512140 ) ) ;
#21602=CARTESIAN_POINT ( 'NONE',  ( 4.806943871629680842, 16.33324523791883109, 6.018569869498933578 ) ) ;
#21608=EDGE_CURVE ( 'NONE', #29972, #20277, #7122, .T. ) ;
#21609=CARTESIAN_POINT ( 'NONE',  ( 12.35846532919129004, 11.73919094318043932, 7.652108011868850035 ) ) ;
#21613=VERTEX_POINT ( 'NONE', #26297 ) ;
#21617=CARTESIAN_POINT ( 'NONE',  ( -5.815855718377446415, -16.25752007041490188, 24.50000000000000000 ) ) ;
#21619=CARTESIAN_POINT ( 'NONE',  ( -18.24831633358132521, -8.229495485092101603, 7.557577766377196582 ) ) ;
#21620=CYLINDRICAL_SURFACE ( 'NONE', #14845, 0.7500000000000006661 ) ;
#21621=CARTESIAN_POINT ( 'NONE',  ( 7.869584159753955532, 10.39565510934977333, 1.500000000000001332 ) ) ;
#21623=CARTESIAN_POINT ( 'NONE',  ( -0.3606176111512335858, -20.01462698034515597, 5.940635272151477686 ) ) ;
#21625=CARTESIAN_POINT ( 'NONE',  ( -13.83213539500865785, 7.758783772730382111, 1.500000000000000000 ) ) ;
#21631=DIRECTION ( 'NONE',  ( -0.9594929736144975907, 0.2817325568414293380, 0.000000000000000000 ) ) ;
#21633=ORIENTED_EDGE ( 'NONE', *, *, #4183, .F. ) ;
#21634=CARTESIAN_POINT ( 'NONE',  ( 4.690519134554619107, 19.44242338873975484, 18.54958172136248251 ) ) ;
#21638=VERTEX_POINT ( 'NONE', #550 ) ;
#21639=EDGE_CURVE ( 'NONE', #24660, #4417, #15317, .T. ) ;
#21642=ORIENTED_EDGE ( 'NONE', *, *, #7314, .T. ) ;
#21643=CARTESIAN_POINT ( 'NONE',  ( 18.67779315278252739, -7.200759110456479206, 19.89182036555910571 ) ) ;
#21644=CARTESIAN_POINT ( 'NONE',  ( 16.56580381663017576, 4.144794415032112767, 19.03762469184452755 ) ) ;
#21647=CARTESIAN_POINT ( 'NONE',  ( 15.40878509682498709, -7.233835690006360508, 19.66962785902261146 ) ) ;
#21648=VECTOR ( 'NONE', #21914, 1000.000000000000000 ) ;
#21652=CARTESIAN_POINT ( 'NONE',  ( -12.81275022540756581, 11.20978530020977182, 19.87181966307587544 ) ) ;
#21653=CARTESIAN_POINT ( 'NONE',  ( -9.895604986052601859, -17.40083251127919794, 18.64703902303423178 ) ) ;
#21657=ORIENTED_EDGE ( 'NONE', *, *, #366, .T. ) ;
#21658=CARTESIAN_POINT ( 'NONE',  ( 9.579384792474776589, -14.08793303971873101, 7.595116371587256054 ) ) ;
#21661=LINE ( 'NONE', #4984, #5842 ) ;
#21666=LINE ( 'NONE', #149, #21294 ) ;
#21667=CARTESIAN_POINT ( 'NONE',  ( -5.754904482333548899, 19.17304367822654854, 7.632642797338977658 ) ) ;
#21668=CARTESIAN_POINT ( 'NONE',  ( 11.80522207451355143, 12.33118449395948169, 7.269896094239230777 ) ) ;
#21669=ADVANCED_FACE ( 'NONE', ( #25997 ), #23629, .F. ) ;
#21674=DIRECTION ( 'NONE',  ( 0.000000000000000000, 0.000000000000000000, 1.000000000000000000 ) ) ;
#21675=EDGE_LOOP ( 'NONE', ( #12042, #28637, #18861, #15002 ) ) ;
#21678=DIRECTION ( 'NONE',  ( -0.000000000000000000, -0.000000000000000000, -1.000000000000000000 ) ) ;
#21679=CARTESIAN_POINT ( 'NONE',  ( 16.59792644102986614, 3.991267607033987197, 19.96568007040468729 ) ) ;
#21686=CARTESIAN_POINT ( 'NONE',  ( -18.25569084301828582, -8.169747224523369766, 5.775318986477950389 ) ) ;
#21689=FACE_OUTER_BOUND ( 'NONE', #16259, .T. ) ;
#21697=CARTESIAN_POINT ( 'NONE',  ( -17.86647173498021957, -9.028149653223259463, 20.25542030744407640 ) ) ;
#21698=LINE ( 'NONE', #26401, #5267 ) ;
#21705=CARTESIAN_POINT ( 'NONE',  ( 19.59831178344207814, 3.989367808977725804, 7.272192800924339728 ) ) ;
#21709=EDGE_LOOP ( 'NONE', ( #13841, #9524, #29988, #22407 ) ) ;
#21711=CARTESIAN_POINT ( 'NONE',  ( -18.58529988941444699, 7.388276390372320535, 1.500000000000001332 ) ) ;
#21713=VERTEX_POINT ( 'NONE', #22677 ) ;
#21719=CARTESIAN_POINT ( 'NONE',  ( -0.2311899301088675418, -17.01971842090038223, 19.45164628100866722 ) ) ;
#21722=CARTESIAN_POINT ( 'NONE',  ( -7.673856334772120924, -15.25703464229374617, 6.782048567692550378 ) ) ;
#21724=CARTESIAN_POINT ( 'NONE',  ( 1.780236034000290957, -16.98472935612791801, 19.14333282897057842 ) ) ;
#21729=CARTESIAN_POINT ( 'NONE',  ( 14.39714448835433025, 13.90806243540158071, 18.64703902303423178 ) ) ;
#21730=DIRECTION ( 'NONE',  ( 0.000000000000000000, 0.000000000000000000, -1.000000000000000000 ) ) ;
#21735=CARTESIAN_POINT ( 'NONE',  ( -15.16307466679259264, -7.786257835066841437, 5.652196082364323360 ) ) ;
#21736=CARTESIAN_POINT ( 'NONE',  ( -6.051176437752240567, 19.08139585423913331, 5.652605728828373977 ) ) ;
#21737=DIRECTION ( 'NONE',  ( 0.000000000000000000, 0.000000000000000000, 1.000000000000000000 ) ) ;
#21741=CARTESIAN_POINT ( 'NONE',  ( -15.21221250122201596, -7.682808169219079275, 18.35377592296120497 ) ) ;
#21744=EDGE_LOOP ( 'NONE', ( #12744, #982, #3999, #27713 ) ) ;
#21749=LINE ( 'NONE', #5075, #23337 ) ;
#21750=EDGE_CURVE ( 'NONE', #18090, #24218, #14907, .T. ) ;
#21752=EDGE_LOOP ( 'NONE', ( #9599, #27104, #8640, #29169 ) ) ;
#21755=CARTESIAN_POINT ( 'NONE',  ( 5.298970182598332634, 19.30368537022594211, 5.652196082367002106 ) ) ;
#21759=CARTESIAN_POINT ( 'NONE',  ( 6.247918173525853547, 19.01788707503811438, 19.56050940960062690 ) ) ;
#21762=VECTOR ( 'NONE', #28280, 1000.000000000000000 ) ;
#21763=EDGE_CURVE ( 'NONE', #9004, #7775, #17703, .T. ) ;
#21773=CARTESIAN_POINT ( 'NONE',  ( -18.47553274370955734, -7.705290464775616854, 6.641371103590088865 ) ) ;
#21774=CARTESIAN_POINT ( 'NONE',  ( 14.70074466696774174, 13.56107787884953986, 5.679672709359371297 ) ) ;
#21776=CARTESIAN_POINT ( 'NONE',  ( -0.6524377400371697000, -20.00727110999512348, 6.530762810602277924 ) ) ;
#21778=DIRECTION ( 'NONE',  ( 1.000000000000000000, 0.000000000000000000, 0.000000000000000000 ) ) ;
#21784=EDGE_CURVE ( 'NONE', #10643, #15912, #22227, .T. ) ;
#21786=FACE_BOUND ( 'NONE', #25539, .T. ) ;
#21787=CARTESIAN_POINT ( 'NONE',  ( 4.805983152666244429, 19.41435796516022450, 7.528076282304598799 ) ) ;
#21792=AXIS2_PLACEMENT_3D ( 'NONE', #13985, #20984, #21297 ) ;
#21796=ORIENTED_EDGE ( 'NONE', *, *, #13249, .F. ) ;
#21798=CARTESIAN_POINT ( 'NONE',  ( -9.396043825398766813, -14.19290753657280035, 6.755862304746362845 ) ) ;
#21799=EDGE_CURVE ( 'NONE', #27449, #26398, #15360, .T. ) ;
#21800=CARTESIAN_POINT ( 'NONE',  ( 16.08779849516155025, -5.700297231796346509, 20.06253562465620632 ) ) ;
#21801=CARTESIAN_POINT ( 'NONE',  ( -15.95879822657219194, 12.05485308878816220, 19.61564845152808090 ) ) ;
#21802=AXIS2_PLACEMENT_3D ( 'NONE', #735, #10253, #19767 ) ;
#21803=CARTESIAN_POINT ( 'NONE',  ( -4.163336342344337027E-14, 1.387778780781445676E-14, 1.500000000000000000 ) ) ;
#21806=CARTESIAN_POINT ( 'NONE',  ( 15.55762523216159821, -6.926306048554701889, 18.54473042795395088 ) ) ;
#21808=EDGE_CURVE ( 'NONE', #18935, #27782, #15527, .T. ) ;
#21810=CARTESIAN_POINT ( 'NONE',  ( -6.914714884271994322, 18.78545221144173638, 19.58863275299554019 ) ) ;
#21811=CARTESIAN_POINT ( 'NONE',  ( -13.16038179581985723, 10.81844819380990330, 20.29090034784956131 ) ) ;
#21815=FACE_OUTER_BOUND ( 'NONE', #8928, .T. ) ;
#21818=LINE ( 'NONE', #5450, #18367 ) ;
#21820=CARTESIAN_POINT ( 'NONE',  ( 10.75049709165479861, -16.88611404641621405, 5.749228751562096562 ) ) ;
#21823=CARTESIAN_POINT ( 'NONE',  ( -15.49619650379776559, 12.67194488555737131, 7.627891251804737927 ) ) ;
#21827=DIRECTION ( 'NONE',  ( 1.000000000000000000, 0.000000000000000000, 0.000000000000000000 ) ) ;
#21828=CARTESIAN_POINT ( 'NONE',  ( 13.00999358272542850, -0.8602714556717643291, 1.500000000000001332 ) ) ;
#21832=CARTESIAN_POINT ( 'NONE',  ( -16.90598708042468701, 2.083096162940503593, 18.44501272782439827 ) ) ;
#21834=CIRCLE ( 'NONE', #23329, 0.7500000000000006661 ) ;
#21842=CARTESIAN_POINT ( 'NONE',  ( 15.55631266752686770, 12.59833113950373651, 6.641371103590088865 ) ) ;
#21844=CARTESIAN_POINT ( 'NONE',  ( 16.18939002998178722, -5.436351910499668705, 6.447548852708279377 ) ) ;
#21845=CARTESIAN_POINT ( 'NONE',  ( 16.55530288949897155, 4.194058762902726833, 19.47952243369110548 ) ) ;
#21849=CARTESIAN_POINT ( 'NONE',  ( 1.000000000000008438, 16.48749217771910125, 1.500000000000000000 ) ) ;
#21853=ADVANCED_FACE ( 'NONE', ( #23444 ), #11605, .F. ) ;
#21855=FACE_OUTER_BOUND ( 'NONE', #17546, .T. ) ;
#21857=CYLINDRICAL_SURFACE ( 'NONE', #8899, 0.7500000000000006661 ) ;
#21860=AXIS2_PLACEMENT_3D ( 'NONE', #11172, #18353, #6489 ) ;
#21865=CARTESIAN_POINT ( 'NONE',  ( -18.02885658979140970, -8.699255478180123902, 20.34789198813115263 ) ) ;
#21867=CARTESIAN_POINT ( 'NONE',  ( -14.69412328735587003, 13.56780452301002704, 19.60917204426170457 ) ) ;
#21868=CARTESIAN_POINT ( 'NONE',  ( 5.016036949087496311, 16.26541432804313203, 6.714907520933423690 ) ) ;
#21885=ORIENTED_EDGE ( 'NONE', *, *, #2165, .F. ) ;
#21888=DIRECTION ( 'NONE',  ( -1.000000000000000000, 0.000000000000000000, 0.000000000000000000 ) ) ;
#21889=CARTESIAN_POINT ( 'NONE',  ( 5.009972004270265344, 16.26741710164193222, 19.47784884541372108 ) ) ;
#21892=VERTEX_POINT ( 'NONE', #1645 ) ;
#21895=CARTESIAN_POINT ( 'NONE',  ( 14.23411040819767059, 14.07463391211592274, 19.03762469184452755 ) ) ;
#21900=CARTESIAN_POINT ( 'NONE',  ( -17.99270058295303443, -8.773758909272052264, 5.661398277488802755 ) ) ;
#21901=CARTESIAN_POINT ( 'NONE',  ( -6.505190245242042479, 15.79074656234091556, 6.782048567692550378 ) ) ;
#21903=CARTESIAN_POINT ( 'NONE',  ( -15.49172192819003335, -7.063155179282991192, 18.71435384576123440 ) ) ;
#21904=DIRECTION ( 'NONE',  ( 1.000000000000000000, 0.000000000000000000, 0.000000000000000000 ) ) ;
#21912=CIRCLE ( 'NONE', #28913, 0.7500000000000006661 ) ;
#21913=FACE_OUTER_BOUND ( 'NONE', #19408, .T. ) ;
#21914=DIRECTION ( 'NONE',  ( 0.6548607339452890974, 0.7557495743542548272, 0.000000000000000000 ) ) ;
#21915=VERTEX_POINT ( 'NONE', #11158 ) ;
#21917=CARTESIAN_POINT ( 'NONE',  ( 8.884323311075775109, 1.438332125858202692, 1.500000000000001332 ) ) ;
#21919=CARTESIAN_POINT ( 'NONE',  ( -7.717362503654372041, -15.23305454438880702, 19.02573955821369367 ) ) ;
#21933=CARTESIAN_POINT ( 'NONE',  ( -5.881244434206279514, -6.812559277181949646, 21.50000000000000000 ) ) ;
#21937=ADVANCED_FACE ( 'NONE', ( #13658 ), #15668, .F. ) ;
#21944=DIRECTION ( 'NONE',  ( 0.2817325568414296710, 0.9594929736144973687, -0.000000000000000000 ) ) ;
#21947=CARTESIAN_POINT ( 'NONE',  ( 15.52282850165806138, 12.63957212366657501, 19.66989035740801839 ) ) ;
#21950=CARTESIAN_POINT ( 'NONE',  ( 2.878478920843521749, -0.8451976705243363641, 24.50000000000000000 ) ) ;
#21951=CARTESIAN_POINT ( 'NONE',  ( 19.64806919293055287, 3.830191698062870742, 18.56793045041961321 ) ) ;
#21952=AXIS2_PLACEMENT_3D ( 'NONE', #9814, #19327, #1235 ) ;
#21955=CARTESIAN_POINT ( 'NONE',  ( 0.000000000000000000, 0.000000000000000000, 21.50000000000000000 ) ) ;
#21958=EDGE_CURVE ( 'NONE', #16110, #30524, #5051, .T. ) ;
#21959=ADVANCED_FACE ( 'NONE', ( #23915 ), #24559, .T. ) ;
#21960=EDGE_CURVE ( 'NONE', #15068, #23022, #10650, .T. ) ;
#21964=CARTESIAN_POINT ( 'NONE',  ( -6.723597995833587859, 18.85470073956823711, 19.97651184436794125 ) ) ;
#21965=CARTESIAN_POINT ( 'NONE',  ( -12.81506474335657408, 11.20733750501348425, 18.80699882434806369 ) ) ;
#21970=FACE_OUTER_BOUND ( 'NONE', #21292, .T. ) ;
#21973=CARTESIAN_POINT ( 'NONE',  ( 9.096230214749077447, -14.38931669386025192, 6.211014596808754007 ) ) ;
#21976=CARTESIAN_POINT ( 'NONE',  ( 9.640932123708072510, -14.04859418185266584, 7.626437579292365321 ) ) ;
#21978=ORIENTED_EDGE ( 'NONE', *, *, #2285, .F. ) ;
#21981=CARTESIAN_POINT ( 'NONE',  ( 18.53278507915171147, -7.520016387818814430, 20.22386025856690495 ) ) ;
#21982=CARTESIAN_POINT ( 'NONE',  ( 8.499586724479435418, 2.959227181723830036, 21.50000000000000000 ) ) ;
#21984=CARTESIAN_POINT ( 'NONE',  ( 6.262045289545330462, 18.99438835075423881, 6.518927109361845496 ) ) ;
#21987=VECTOR ( 'NONE', #11974, 1000.000000000000000 ) ;
#21988=CARTESIAN_POINT ( 'NONE',  ( -6.974883619896829146, -5.687793815610328707, 21.50000000000000000 ) ) ;
#21989=DIRECTION ( 'NONE',  ( 1.000000000000000000, 0.000000000000000000, 0.000000000000000000 ) ) ;
#21990=CARTESIAN_POINT ( 'NONE',  ( 19.82764810689592849, 2.754998275627142945, 7.557577766377196582 ) ) ;
#21992=CARTESIAN_POINT ( 'NONE',  ( 12.88134121443597380, 11.13293444107316787, 7.272049892295485485 ) ) ;
#21995=CARTESIAN_POINT ( 'NONE',  ( 18.48179574117062529, -7.690589227441819276, 7.603368798681074736 ) ) ;
#21997=CARTESIAN_POINT ( 'NONE',  ( 16.55667234709053659, 4.187688857952014843, 19.21769074125272425 ) ) ;
#21998=VECTOR ( 'NONE', #4286, 1000.000000000000000 ) ;
#22000=ORIENTED_EDGE ( 'NONE', *, *, #23269, .F. ) ;
#22001=CARTESIAN_POINT ( 'NONE',  ( -11.82521593960875528, 5.400395169024524655, 1.500000000000001332 ) ) ;
#22003=CARTESIAN_POINT ( 'NONE',  ( 4.668110441710642711, -19.44758969394385062, 1.500000000000001332 ) ) ;
#22007=AXIS2_PLACEMENT_3D ( 'NONE', #13775, #11443, #20929 ) ;
#22009=CARTESIAN_POINT ( 'NONE',  ( -13.38159811071079552, 10.55828946507379307, 18.34798005862662507 ) ) ;
#22011=ORIENTED_EDGE ( 'NONE', *, *, #29576, .T. ) ;
#22016=AXIS2_PLACEMENT_3D ( 'NONE', #5091, #14276, #16783 ) ;
#22018=DIRECTION ( 'NONE',  ( -0.9898214418809326842, -0.1423148382732852824, 0.000000000000000000 ) ) ;
#22022=ORIENTED_EDGE ( 'NONE', *, *, #15441, .F. ) ;
#22026=DIRECTION ( 'NONE',  ( -0.000000000000000000, -0.000000000000000000, 1.000000000000000000 ) ) ;
#22027=ORIENTED_EDGE ( 'NONE', *, *, #16675, .T. ) ;
#22028=ORIENTED_EDGE ( 'NONE', *, *, #14891, .T. ) ;
#22029=DIRECTION ( 'NONE',  ( 0.000000000000000000, 0.000000000000000000, 1.000000000000000000 ) ) ;
#22035=DIRECTION ( 'NONE',  ( 0.000000000000000000, 0.000000000000000000, 1.000000000000000000 ) ) ;
#22040=CARTESIAN_POINT ( 'NONE',  ( -11.25470158702820456, -16.53282404628957991, 7.156831654632821227 ) ) ;
#22042=FACE_OUTER_BOUND ( 'NONE', #2112, .T. ) ;
#22046=CARTESIAN_POINT ( 'NONE',  ( -17.64660589602034690, -9.450098986197513540, 7.098451512883313441 ) ) ;
#22047=CARTESIAN_POINT ( 'NONE',  ( -5.764374838704561910, 16.04809504443726098, 5.678370764302467677 ) ) ;
#22050=CARTESIAN_POINT ( 'NONE',  ( -15.56928374346769495, -6.880100827600170277, 19.11611934778430921 ) ) ;
#22056=DIRECTION ( 'NONE',  ( -0.000000000000000000, -0.000000000000000000, 1.000000000000000000 ) ) ;
#22057=CARTESIAN_POINT ( 'NONE',  ( -14.78913018809137370, 13.49064936509565982, 7.176035686813569292 ) ) ;
#22059=ORIENTED_EDGE ( 'NONE', *, *, #11159, .F. ) ;
#22064=ORIENTED_EDGE ( 'NONE', *, *, #27567, .T. ) ;
#22065=CARTESIAN_POINT ( 'NONE',  ( 4.564720541824407896, 16.40857754966928184, 18.49267272388512140 ) ) ;
#22067=CARTESIAN_POINT ( 'NONE',  ( 0.000000000000000000, 0.000000000000000000, 1.500000000000001332 ) ) ;
#22075=ORIENTED_EDGE ( 'NONE', *, *, #24594, .F. ) ;
#22076=DIRECTION ( 'NONE',  ( -0.000000000000000000, -0.000000000000000000, 1.000000000000000000 ) ) ;
#22077=CARTESIAN_POINT ( 'NONE',  ( 14.73074142449663881, 5.627958522269737252, 24.50000000000000000 ) ) ;
#22085=CARTESIAN_POINT ( 'NONE',  ( 0.000000000000000000, 0.000000000000000000, 1.500000000000001332 ) ) ;
#22087=CARTESIAN_POINT ( 'NONE',  ( -19.84344116185557283, 2.497567387674354489, 7.652108011868850035 ) ) ;
#22088=ORIENTED_EDGE ( 'NONE', *, *, #17973, .F. ) ;
#22089=ORIENTED_EDGE ( 'NONE', *, *, #4571, .F. ) ;
#22092=CARTESIAN_POINT ( 'NONE',  ( -1.438332125858111432, 8.884323311075791096, 21.50000000000000000 ) ) ;
#22097=CARTESIAN_POINT ( 'NONE',  ( 12.57902516942791493, 11.48976026227457936, 18.39701043959520987 ) ) ;
#22098=B_SPLINE_CURVE_WITH_KNOTS ( 'NONE', 3,
 ( #8764, #10971, #27350, #12997, #17834, #1459, #18289, #8488, #22641, #27647, #13473, #13307, #5975, #22805, #17990, #6437, #22954, #11118 ),
 .UNSPECIFIED., .F., .F.,
 ( 4, 2, 2, 2, 2, 2, 2, 2, 4 ),
 ( 0.003174295595554288765, 0.003570702171545512855, 0.003967108747536736944, 0.004363515323527961468, 0.004759921899519185123, 0.005156328475510408779, 0.005552735051501633302, 0.005949141627492857826, 0.006345548203484081481 ),
 .UNSPECIFIED. ) ;
#22100=ORIENTED_EDGE ( 'NONE', *, *, #24030, .T. ) ;
#22102=CARTESIAN_POINT ( 'NONE',  ( 18.43859109590531276, -7.792859017390148857, 20.32367522806703874 ) ) ;
#22103=CARTESIAN_POINT ( 'NONE',  ( 18.28487737789067324, -8.104377114558880990, 5.651480102388687143 ) ) ;
#22106=CARTESIAN_POINT ( 'NONE',  ( -4.699300155657183176, 16.36248368692915989, 18.83976166372256245 ) ) ;
#22108=B_SPLINE_CURVE_WITH_KNOTS ( 'NONE', 3,
 ( #19104, #28620, #7244, #10121, #29899, #5292, #29318, #9983, #3114, #26661, #30041, #5456, #14958, #24317, #3693, #25364, #12483, #3997 ),
 .UNSPECIFIED., .F., .F.,
 ( 4, 2, 2, 2, 2, 2, 2, 2, 4 ),
 ( 0.003174295595554316521, 0.003570702171545547983, 0.003967108747536779445, 0.004363515323528011775, 0.004759921899519242369, 0.005156328475510474699, 0.005552735051501706161, 0.005949141627492937623, 0.006345548203484169085 ),
 .UNSPECIFIED. ) ;
#22110=ORIENTED_EDGE ( 'NONE', *, *, #29608, .T. ) ;
#22112=CIRCLE ( 'NONE', #12675, 0.7499999999999997780 ) ;
#22114=CARTESIAN_POINT ( 'NONE',  ( 16.66634534075878094, 3.639270104310704745, 5.749491821935610147 ) ) ;
#22115=CARTESIAN_POINT ( 'NONE',  ( -14.68399241520484111, 13.60504237629023194, 19.33715507985239412 ) ) ;
#22120=ORIENTED_EDGE ( 'NONE', *, *, #6157, .T. ) ;
#22121=CARTESIAN_POINT ( 'NONE',  ( -19.91230480659700319, 2.053870633397346435, 5.749491821935610147 ) ) ;
#22132=DIRECTION ( 'NONE',  ( 1.000000000000000000, 0.000000000000000000, 0.000000000000000000 ) ) ;
#22133=ORIENTED_EDGE ( 'NONE', *, *, #13572, .F. ) ;
#22135=CARTESIAN_POINT ( 'NONE',  ( 6.812559277181973627, -5.881244434206257310, 1.500000000000001332 ) ) ;
#22143=CARTESIAN_POINT ( 'NONE',  ( 16.87846183053957461, 2.201534687727673578, 6.530762810602277924 ) ) ;
#22145=ORIENTED_EDGE ( 'NONE', *, *, #7857, .T. ) ;
#22146=CARTESIAN_POINT ( 'NONE',  ( 14.97341519046260494, 13.28616376876794547, 7.652108011868850035 ) ) ;
#22147=EDGE_LOOP ( 'NONE', ( #23720, #12845, #27617, #15574 ) ) ;
#22155=EDGE_CURVE ( 'NONE', #194, #13705, #27832, .T. ) ;
#22157=ORIENTED_EDGE ( 'NONE', *, *, #19319, .F. ) ;
#22161=CARTESIAN_POINT ( 'NONE',  ( 10.33891776879019808, -17.14136798460503996, 19.77662771831109367 ) ) ;
#22162=DIRECTION ( 'NONE',  ( 1.000000000000000000, 0.000000000000000000, 0.000000000000000000 ) ) ;
#22163=ORIENTED_EDGE ( 'NONE', *, *, #15083, .T. ) ;
#22165=CARTESIAN_POINT ( 'NONE',  ( -13.52555592105307980, 10.38406032642568455, 18.37415474056476938 ) ) ;
#22169=EDGE_CURVE ( 'NONE', #19541, #8561, #5480, .T. ) ;
#22173=CARTESIAN_POINT ( 'NONE',  ( 8.606594496258196614, 4.390207617113981442, 21.50000000000000000 ) ) ;
#22178=CARTESIAN_POINT ( 'NONE',  ( 19.63396244889325715, 3.810028285208273857, 5.853797745100183469 ) ) ;
#22179=VERTEX_POINT ( 'NONE', #318 ) ;
#22181=CARTESIAN_POINT ( 'NONE',  ( -4.163336342344337027E-14, 1.387778780781445676E-14, 1.500000000000000000 ) ) ;
#22182=CARTESIAN_POINT ( 'NONE',  ( 9.436481611552752113, 0.9307681286968852996, 13.00000000000000178 ) ) ;
#22183=ORIENTED_EDGE ( 'NONE', *, *, #7231, .T. ) ;
#22185=ORIENTED_EDGE ( 'NONE', *, *, #14908, .F. ) ;
#22188=VERTEX_POINT ( 'NONE', #16283 ) ;
#22195=ORIENTED_EDGE ( 'NONE', *, *, #14950, .F. ) ;
#22196=LINE ( 'NONE', #832, #8410 ) ;
#22202=EDGE_CURVE ( 'NONE', #4883, #5400, #15341, .T. ) ;
#22203=CARTESIAN_POINT ( 'NONE',  ( -9.085694127122227570, -14.40282604532831812, 20.12545155307891065 ) ) ;
#22205=CARTESIAN_POINT ( 'NONE',  ( -6.495433978329088198, 18.93455902173411687, 5.810767894563978686 ) ) ;
#22207=CARTESIAN_POINT ( 'NONE',  ( 11.24508296785401917, -16.56092475412858533, 5.661398277488802755 ) ) ;
#22211=ORIENTED_EDGE ( 'NONE', *, *, #20437, .T. ) ;
#22214=CARTESIAN_POINT ( 'NONE',  ( -8.099370871114970782, -15.01721251069485596, 7.545655578832109356 ) ) ;
#22215=CARTESIAN_POINT ( 'NONE',  ( -14.70245401545669139, 13.58508552794529223, 6.420335371522007506 ) ) ;
#22227=LINE ( 'NONE', #5547, #24316 ) ;
#22229=CIRCLE ( 'NONE', #810, 1.000000000000009548 ) ;
#22230=DIRECTION ( 'NONE',  ( 1.000000000000000000, 0.000000000000000000, 0.000000000000000000 ) ) ;
#22233=DIRECTION ( 'NONE',  ( 0.1423148382732889183, 0.9898214418809321291, 0.000000000000000000 ) ) ;
#22236=CARTESIAN_POINT ( 'NONE',  ( 13.01350570279883634, 10.97146294988705506, 19.41069149716887310 ) ) ;
#22237=DIRECTION ( 'NONE',  ( 0.000000000000000000, 0.000000000000000000, 1.000000000000000000 ) ) ;
#22244=DIRECTION ( 'NONE',  ( 0.000000000000000000, 0.000000000000000000, -1.000000000000000000 ) ) ;
#22246=DIRECTION ( 'NONE',  ( -1.000000000000000000, 0.000000000000000000, 0.000000000000000000 ) ) ;
#22247=DIRECTION ( 'NONE',  ( 0.000000000000000000, 0.000000000000000000, 1.000000000000000000 ) ) ;
#22249=VERTEX_POINT ( 'NONE', #29645 ) ;
#22250=CIRCLE ( 'NONE', #15775, 9.482273699623480212 ) ;
#22257=CARTESIAN_POINT ( 'NONE',  ( 12.77210943289887801, 11.26383436979580566, 18.55820869691756769 ) ) ;
#22258=VERTEX_POINT ( 'NONE', #10614 ) ;
#22259=CARTESIAN_POINT ( 'NONE',  ( -16.81771903218351838, 2.627522578025005107, 6.864725433338323413 ) ) ;
#22260=CARTESIAN_POINT ( 'NONE',  ( 19.65054205152828004, 3.817440173033144202, 20.13759033520874908 ) ) ;
#22263=CARTESIAN_POINT ( 'NONE',  ( -4.580173031745207624, 16.39361746661297659, 19.47784884541372818 ) ) ;
#22265=CARTESIAN_POINT ( 'NONE',  ( -16.89565484000427986, 2.154541803992424231, 20.22273502201483453 ) ) ;
#22269=CARTESIAN_POINT ( 'NONE',  ( 16.55580462840120504, 4.191719245021451101, 6.782048567692550378 ) ) ;
#22272=CARTESIAN_POINT ( 'NONE',  ( 0.7788148816922453310, -17.02744011591805062, 7.652108011868850923 ) ) ;
#22274=CARTESIAN_POINT ( 'NONE',  ( 8.743977807160074889, 3.668292057956028973, 1.500000000000001332 ) ) ;
#22279=CARTESIAN_POINT ( 'NONE',  ( 10.28124378133233741, -17.17592898829030901, 6.864725433338323413 ) ) ;
#22282=AXIS2_PLACEMENT_3D ( 'NONE', #2180, #21502, #12320 ) ;
#22287=CARTESIAN_POINT ( 'NONE',  ( 18.64396409872438198, -7.239577540284320989, 19.96797677718664232 ) ) ;
#22295=B_SPLINE_CURVE_WITH_KNOTS ( 'NONE', 3,
 ( #25887, #4978, #30558, #28218, #6698, #25730, #19023, #26187, #2487, #11690, #139, #19168, #16678, #7010, #9658, #30702 ),
 .UNSPECIFIED., .F., .F.,
 ( 4, 2, 2, 2, 2, 2, 2, 4 ),
 ( 0.4999999999999998890, 0.6250000000000012212, 0.6875000000000019984, 0.7187500000000022204, 0.7500000000000026645, 0.8125000000000017764, 0.8750000000000007772, 1.000000000000000000 ),
 .UNSPECIFIED. ) ;
#22296=AXIS2_PLACEMENT_3D ( 'NONE', #18637, #15988, #6768 ) ;
#22297=DIRECTION ( 'NONE',  ( 1.000000000000000000, 0.000000000000000000, 0.000000000000000000 ) ) ;
#22299=CARTESIAN_POINT ( 'NONE',  ( 19.89647750965486495, 2.201534687727673578, 6.530762810602277924 ) ) ;
#22301=CARTESIAN_POINT ( 'NONE',  ( 12.82328378257164836, 11.20259424400691195, 5.940635272151477686 ) ) ;
#22302=ORIENTED_EDGE ( 'NONE', *, *, #10961, .T. ) ;
#22306=VERTEX_POINT ( 'NONE', #15274 ) ;
#22313=VECTOR ( 'NONE', #14125, 1000.000000000000000 ) ;
#22315=CIRCLE ( 'NONE', #10861, 0.7500000000000006661 ) ;
#22317=CARTESIAN_POINT ( 'NONE',  ( 10.30179067644846747, -17.16362715220463642, 19.66989035740801839 ) ) ;
#22319=CARTESIAN_POINT ( 'NONE',  ( 10.42970548045642332, -17.06546344489796851, 18.72886616302736940 ) ) ;
#22320=ORIENTED_EDGE ( 'NONE', *, *, #24823, .T. ) ;
#22324=CARTESIAN_POINT ( 'NONE',  ( -15.76141475779637879, 12.34077778289585048, 18.56793045041961321 ) ) ;
#22327=ORIENTED_EDGE ( 'NONE', *, *, #16853, .F. ) ;
#22329=EDGE_CURVE ( 'NONE', #2507, #24787, #11910, .T. ) ;
#22330=B_SPLINE_SURFACE_WITH_KNOTS ( 'NONE', 3, 1, ( 
 ( #9608, #30499 ),
 ( #25838, #14264 ),
 ( #2116, #28166 ),
 ( #14441, #25988 ),
 ( #21449, #6795 ),
 ( #11494, #1973 ),
 ( #23622, #16771 ),
 ( #4472, #23943 ),
 ( #2589, #12106 ),
 ( #2265, #11634 ),
 ( #13980, #21126 ),
 ( #20977, #30646 ),
 ( #23784, #9292 ),
 ( #4615, #9752 ),
 ( #4759, #18660 ),
 ( #18817, #26129 ),
 ( #28336, #6961 ),
 ( #16622, #14116 ),
 ( #91, #26287 ),
 ( #16471, #19117 ),
 ( #4924, #21602 ),
 ( #240, #28635 ),
 ( #25679, #30813 ),
 ( #7259, #11785 ),
 ( #21290, #9460 ),
 ( #18975, #19266 ),
 ( #28485, #6647 ),
 ( #7114, #16164 ),
 ( #4300, #13830 ),
 ( #27066, #2899 ),
 ( #21755, #697 ) ),
 .UNSPECIFIED., .F., .F., .F.,
 ( 4, 3, 3, 3, 3, 3, 3, 3, 3, 3, 4 ),
 ( 2, 2 ),
 ( 0.000000000000000000, 0.05425176834609633791, 0.1085332949128352958, 0.1623767749169382768, 0.2157504826133063158, 0.2688657508888171455, 0.3218907763505476360, 0.3749548578363336993, 0.4282048033836242107, 0.4818374082110501444, 0.4999999999131655715 ),
 ( 0.000000000000000000, 1.000000000000000000 ),
 .UNSPECIFIED. ) ;
#22341=AXIS2_PLACEMENT_3D ( 'NONE', #28142, #16285, #25179 ) ;
#22343=ORIENTED_EDGE ( 'NONE', *, *, #12223, .F. ) ;
#22345=DIRECTION ( 'NONE',  ( 0.000000000000000000, 0.000000000000000000, 1.000000000000000000 ) ) ;
#22348=CARTESIAN_POINT ( 'NONE',  ( -2.703030265324078307, -12.75514121382991384, 24.50000000000000000 ) ) ;
#22355=CARTESIAN_POINT ( 'NONE',  ( 9.185733585337910512, -2.352830851074146246, 21.50000000000000000 ) ) ;
#22359=DIRECTION ( 'NONE',  ( 0.000000000000000000, 0.000000000000000000, 1.000000000000000000 ) ) ;
#22360=DIRECTION ( 'NONE',  ( 1.000000000000000000, 0.000000000000000000, 0.000000000000000000 ) ) ;
#22363=EDGE_LOOP ( 'NONE', ( #15395, #29480, #4114, #20383 ) ) ;
#22364=ADVANCED_FACE ( 'NONE', ( #29127 ), #7458, .F. ) ;
#22365=AXIS2_PLACEMENT_3D ( 'NONE', #11179, #20832, #25980 ) ;
#22366=CARTESIAN_POINT ( 'NONE',  ( -11.33306590618138543, -16.50086680533498296, 19.66989035740801839 ) ) ;
#22367=DIRECTION ( 'NONE',  ( 0.000000000000000000, 0.000000000000000000, -1.000000000000000000 ) ) ;
#22369=CARTESIAN_POINT ( 'NONE',  ( 10.67336573878037775, -13.33112751634290127, 6.892848776733236704 ) ) ;
#22372=AXIS2_PLACEMENT_3D ( 'NONE', #14069, #1923, #1772 ) ;
#22379=CARTESIAN_POINT ( 'NONE',  ( -0.1984805017666675109, -17.02075843868213667, 6.910395520694541993 ) ) ;
#22381=CARTESIAN_POINT ( 'NONE',  ( -7.974144905643821168, -5.130938270761582487, 13.00000000000000178 ) ) ;
#22383=DIRECTION ( 'NONE',  ( 1.000000000000000000, 0.000000000000000000, 0.000000000000000000 ) ) ;
#22394=DIRECTION ( 'NONE',  ( 0.000000000000000000, 0.000000000000000000, 1.000000000000000000 ) ) ;
#22395=CARTESIAN_POINT ( 'NONE',  ( -19.80925230797852876, 2.758332870380178825, 20.32243167357988511 ) ) ;
#22398=CARTESIAN_POINT ( 'NONE',  ( -5.687793815610304726, 6.974883619896852238, 1.500000000000001332 ) ) ;
#22399=DIRECTION ( 'NONE',  ( 0.000000000000000000, 0.000000000000000000, 1.000000000000000000 ) ) ;
#22400=FACE_OUTER_BOUND ( 'NONE', #8381, .T. ) ;
#22403=ORIENTED_EDGE ( 'NONE', *, *, #6894, .T. ) ;
#22407=ORIENTED_EDGE ( 'NONE', *, *, #13184, .T. ) ;
#22409=CARTESIAN_POINT ( 'NONE',  ( -11.40980092660686829, 6.310027164379044429, 1.500000000000001332 ) ) ;
#22414=LINE ( 'NONE', #1057, #28116 ) ;
#22416=ORIENTED_EDGE ( 'NONE', *, *, #11336, .F. ) ;
#22418=FACE_OUTER_BOUND ( 'NONE', #5917, .T. ) ;
#22419=CARTESIAN_POINT ( 'NONE',  ( 19.76130184095197961, 3.194145055459935101, 20.34789198813115263 ) ) ;
#22422=DIRECTION ( 'NONE',  ( 0.000000000000000000, 0.000000000000000000, -1.000000000000000000 ) ) ;
#22425=VERTEX_POINT ( 'NONE', #11027 ) ;
#22428=CARTESIAN_POINT ( 'NONE',  ( 19.63091490780798409, 3.916522693408249545, 5.951255046771932733 ) ) ;
#22435=CARTESIAN_POINT ( 'NONE',  ( 9.138492726993304061, -14.36378254522092135, 6.111214848085761986 ) ) ;
#22436=CARTESIAN_POINT ( 'NONE',  ( 11.56680498864186291, -16.33760111733343123, 18.50655187082627862 ) ) ;
#22441=LINE ( 'NONE', #10127, #19094 ) ;
#22442=CARTESIAN_POINT ( 'NONE',  ( -5.978582851986702806, 19.10413308555694911, 5.652196082367002106 ) ) ;
#22448=LINE ( 'NONE', #13264, #21184 ) ;
#22450=CARTESIAN_POINT ( 'NONE',  ( 19.89475757678375345, 2.217009531549524848, 6.864725433338323413 ) ) ;
#22452=DIRECTION ( 'NONE',  ( 1.000000000000000000, 0.000000000000000000, 0.000000000000000000 ) ) ;
#22453=ORIENTED_EDGE ( 'NONE', *, *, #6134, .T. ) ;
#22454=CARTESIAN_POINT ( 'NONE',  ( -13.71336669116180929, 10.15199454966009718, 18.45571264222803975 ) ) ;
#22460=CARTESIAN_POINT ( 'NONE',  ( 14.73074142449663881, 5.627958522269738140, 1.500000000000001332 ) ) ;
#22465=ORIENTED_EDGE ( 'NONE', *, *, #20633, .F. ) ;
#22467=CARTESIAN_POINT ( 'NONE',  ( -15.69442553397267304, 12.42550873695622826, 20.19593175699879595 ) ) ;
#22468=CARTESIAN_POINT ( 'NONE',  ( 1.000000000000008438, 17.23749217771910480, 24.50000000000000000 ) ) ;
#22469=DIRECTION ( 'NONE',  ( 0.000000000000000000, 0.000000000000000000, 1.000000000000000000 ) ) ;
#22470=ORIENTED_EDGE ( 'NONE', *, *, #19009, .F. ) ;
#22483=CARTESIAN_POINT ( 'NONE',  ( -1.000000000000008438, 13.00000000000001421, 1.500000000000001332 ) ) ;
#22489=CARTESIAN_POINT ( 'NONE',  ( 12.24063095261064404, 4.490763173670002217, 24.50000000000000000 ) ) ;
#22490=ORIENTED_EDGE ( 'NONE', *, *, #11319, .T. ) ;
#22493=CIRCLE ( 'NONE', #29485, 0.7500000000000006661 ) ;
#22498=ADVANCED_FACE ( 'NONE', ( #20382 ), #3545, .F. ) ;
#22500=DIRECTION ( 'NONE',  ( -0.000000000000000000, -0.000000000000000000, 1.000000000000000000 ) ) ;
#22501=CARTESIAN_POINT ( 'NONE',  ( 12.13430697852916929, 11.98518526348621016, 20.29915277494337644 ) ) ;
#22506=CARTESIAN_POINT ( 'NONE',  ( -4.604861147465549642, 16.38721654675108752, 6.910395520694541993 ) ) ;
#22507=CARTESIAN_POINT ( 'NONE',  ( 11.71757112412214141, -16.22992597261980308, 5.951255046771932733 ) ) ;
#22510=VERTEX_POINT ( 'NONE', #15384 ) ;
#22515=CARTESIAN_POINT ( 'NONE',  ( -12.72607405277288350, 11.30422146305940245, 6.420335371522007506 ) ) ;
#22517=DIRECTION ( 'NONE',  ( -0.000000000000000000, -0.000000000000000000, 1.000000000000000000 ) ) ;
#22518=VECTOR ( 'NONE', #10986, 1000.000000000000000 ) ;
#22520=CARTESIAN_POINT ( 'NONE',  ( 3.794966104506363180, 16.62713903699921048, 7.652108011868852699 ) ) ;
#22523=CARTESIAN_POINT ( 'NONE',  ( -8.925879454855033757, -14.50801274514188677, 7.557577766377196582 ) ) ;
#22525=CARTESIAN_POINT ( 'NONE',  ( 5.721595087358985587, 19.18273663903466897, 18.44501272782439827 ) ) ;
#22526=EDGE_CURVE ( 'NONE', #26251, #17832, #9412, .T. ) ;
#22529=ORIENTED_EDGE ( 'NONE', *, *, #24076, .F. ) ;
#22531=CARTESIAN_POINT ( 'NONE',  ( 11.93826604606910990, -16.04611492155651575, 6.788986777570701570 ) ) ;
#22533=CARTESIAN_POINT ( 'NONE',  ( -1.000000000000008438, 13.00000000000001421, 1.500000000000001332 ) ) ;
#22539=AXIS2_PLACEMENT_3D ( 'NONE', #28133, #16428, #2071 ) ;
#22542=CIRCLE ( 'NONE', #29528, 1.000000000000007772 ) ;
#22545=CARTESIAN_POINT ( 'NONE',  ( -19.91398265452221850, -1.852915226174652208, 24.50000000000000000 ) ) ;
#22546=DIRECTION ( 'NONE',  ( 1.000000000000000000, 0.000000000000000000, 0.000000000000000000 ) ) ;
#22547=CARTESIAN_POINT ( 'NONE',  ( -20.00000000000004263, 1.387778780781445676E-14, 24.50000000000000000 ) ) ;
#22553=DIRECTION ( 'NONE',  ( -0.000000000000000000, -0.000000000000000000, 1.000000000000000000 ) ) ;
#22559=PLANE ( 'NONE',  #23835 ) ;
#22561=DIRECTION ( 'NONE',  ( 1.000000000000000000, 0.000000000000000000, 0.000000000000000000 ) ) ;
#22564=AXIS2_PLACEMENT_3D ( 'NONE', #2066, #26084, #16725 ) ;
#22565=CARTESIAN_POINT ( 'NONE',  ( -19.84651427434117821, 2.615565199888951309, 7.652108011868850035 ) ) ;
#22566=CARTESIAN_POINT ( 'NONE',  ( 16.66826434373539811, 3.628879393376897244, 20.25542030744407640 ) ) ;
#22567=CARTESIAN_POINT ( 'NONE',  ( 15.21635490854752781, 12.97988522761634478, 7.526993102356318133 ) ) ;
#22569=ORIENTED_EDGE ( 'NONE', *, *, #2266, .T. ) ;
#22570=DIRECTION ( 'NONE',  ( -0.000000000000000000, -0.000000000000000000, 1.000000000000000000 ) ) ;
#22574=CARTESIAN_POINT ( 'NONE',  ( -6.222613296526853688, 19.00773140132666938, 20.32200205377525393 ) ) ;
#22577=CARTESIAN_POINT ( 'NONE',  ( 9.248129367672065726, 2.094186647214772989, 13.00000000000000178 ) ) ;
#22579=CARTESIAN_POINT ( 'NONE',  ( 1.767905995587313761, -16.98559759804296476, 6.917457548096558995 ) ) ;
#22581=CIRCLE ( 'NONE', #30075, 9.482273699623480212 ) ;
#22582=CARTESIAN_POINT ( 'NONE',  ( -8.978548835163147501, -14.47379921348856868, 7.526951045817043884 ) ) ;
#22583=DIRECTION ( 'NONE',  ( -0.000000000000000000, -0.000000000000000000, 1.000000000000000000 ) ) ;
#22587=LINE ( 'NONE', #17929, #20750 ) ;
#22588=ADVANCED_FACE ( 'NONE', ( #25831 ), #20972, .F. ) ;
#22594=DIRECTION ( 'NONE',  ( 1.000000000000000000, 0.000000000000000000, 0.000000000000000000 ) ) ;
#22595=CARTESIAN_POINT ( 'NONE',  ( -4.863253556059218496, 16.31819504766686890, 5.940635272151477686 ) ) ;
#22596=ORIENTED_EDGE ( 'NONE', *, *, #13608, .T. ) ;
#22598=CARTESIAN_POINT ( 'NONE',  ( -3.000000000000041744, 1.387778780781445676E-14, 24.50000000000000000 ) ) ;
#22599=CARTESIAN_POINT ( 'NONE',  ( -9.436481611552759219, -0.9307681286968260137, 1.500000000000001332 ) ) ;
#22603=CARTESIAN_POINT ( 'NONE',  ( 16.82202058066697248, 2.664153601443037367, 5.796888747622817029 ) ) ;
#22609=CARTESIAN_POINT ( 'NONE',  ( -13.88572908629245184, 9.930151408457417617, 19.96568007040468729 ) ) ;
#22613=VERTEX_POINT ( 'NONE', #8837 ) ;
#22614=VECTOR ( 'NONE', #4881, 1000.000000000000000 ) ;
#22615=CARTESIAN_POINT ( 'NONE',  ( 3.062389757841103677, 16.80148204205677587, 6.672349528511551497 ) ) ;
#22617=CARTESIAN_POINT ( 'NONE',  ( 5.296161872597624942, 19.28602264385379428, 20.34789198813115263 ) ) ;
#22618=DIRECTION ( 'NONE',  ( -1.000000000000000000, 0.000000000000000000, 0.000000000000000000 ) ) ;
#22620=CARTESIAN_POINT ( 'NONE',  ( 19.88037316481945282, 2.342382300094908665, 19.87181966307587544 ) ) ;
#22621=EDGE_LOOP ( 'NONE', ( #18397, #11980, #10680, #23393 ) ) ;
#22623=CARTESIAN_POINT ( 'NONE',  ( 15.40995608898785107, -7.231564984717128830, 6.310736198168394928 ) ) ;
#22624=CARTESIAN_POINT ( 'NONE',  ( -13.95900029477595439, 9.834024558217739909, 18.92976555901915603 ) ) ;
#22626=ORIENTED_EDGE ( 'NONE', *, *, #9142, .T. ) ;
#22630=CARTESIAN_POINT ( 'NONE',  ( -5.973960059363100150, 19.10558826632600216, 20.34789198813115263 ) ) ;
#22632=CYLINDRICAL_SURFACE ( 'NONE', #20562, 1.000000000000008660 ) ;
#22634=CARTESIAN_POINT ( 'NONE',  ( 16.87629972246965337, 2.221555249129149257, 6.385774490351134425 ) ) ;
#22638=DIRECTION ( 'NONE',  ( -0.000000000000000000, -0.000000000000000000, 1.000000000000000000 ) ) ;
#22641=CARTESIAN_POINT ( 'NONE',  ( -19.69217677393684696, 3.495450461901487671, 6.781503518395076036 ) ) ;
#22642=DIRECTION ( 'NONE',  ( 0.000000000000000000, 0.000000000000000000, 1.000000000000000000 ) ) ;
#22644=CARTESIAN_POINT ( 'NONE',  ( -0.6299556268942230197, -19.99014111075367595, 6.386539667786101937 ) ) ;
#22645=VECTOR ( 'NONE', #15156, 1000.000000000000000 ) ;
#22649=CARTESIAN_POINT ( 'NONE',  ( -5.621668343899183462, 16.09410144477764604, 18.34838970509067479 ) ) ;
#22650=CARTESIAN_POINT ( 'NONE',  ( -11.64054540341807353, 16.26338533980437262, 1.500000000000001332 ) ) ;
#22651=DIRECTION ( 'NONE',  ( 0.000000000000000000, 0.000000000000000000, 1.000000000000000000 ) ) ;
#22652=CARTESIAN_POINT ( 'NONE',  ( 14.79741041486972897, 13.48156734445488070, 20.33971507717571114 ) ) ;
#22653=DIRECTION ( 'NONE',  ( 0.000000000000000000, 0.000000000000000000, 1.000000000000000000 ) ) ;
#22656=CARTESIAN_POINT ( 'NONE',  ( -9.269489102446176076, -14.27959628656685886, 18.80699882434806369 ) ) ;
#22658=LINE ( 'NONE', #30453, #15037 ) ;
#22659=CARTESIAN_POINT ( 'NONE',  ( 11.87672590887049573, -16.11366389249059594, 6.233981582756856987 ) ) ;
#22663=ORIENTED_EDGE ( 'NONE', *, *, #12020, .T. ) ;
#22672=CARTESIAN_POINT ( 'NONE',  ( -8.917851762035224894, -14.51287734179233802, 5.749228751562096562 ) ) ;
#22674=CARTESIAN_POINT ( 'NONE',  ( -13.00999358272542494, -0.8602714556717691030, 1.500000000000001332 ) ) ;
#22677=CARTESIAN_POINT ( 'NONE',  ( -4.622016212553093695, -12.19167610014704906, 24.50000000000000000 ) ) ;
#22681=ORIENTED_EDGE ( 'NONE', *, *, #4314, .T. ) ;
#22690=CARTESIAN_POINT ( 'NONE',  ( -16.99844672487172659, 1.385815296940135388, 5.653604225791664994 ) ) ;
#22692=DIRECTION ( 'NONE',  ( 0.000000000000000000, 0.000000000000000000, 1.000000000000000000 ) ) ;
#22694=DIRECTION ( 'NONE',  ( -0.000000000000000000, -0.000000000000000000, -1.000000000000000000 ) ) ;
#22695=ADVANCED_FACE ( 'NONE', ( #1664 ), #21123, .F. ) ;
#22696=CARTESIAN_POINT ( 'NONE',  ( 9.007774317138279585, -14.44244895400450801, 6.714907520933423690 ) ) ;
#22697=CARTESIAN_POINT ( 'NONE',  ( 5.296161872597630271, 19.28602264385381204, 7.652108011868850035 ) ) ;
#22699=ORIENTED_EDGE ( 'NONE', *, *, #28347, .F. ) ;
#22701=CARTESIAN_POINT ( 'NONE',  ( -13.00999358272542494, -0.8602714556717691030, 1.500000000000001332 ) ) ;
#22703=ADVANCED_FACE ( 'NONE', ( #25527 ), #6341, .F. ) ;
#22709=AXIS2_PLACEMENT_3D ( 'NONE', #22085, #14462, #10086 ) ;
#22710=EDGE_CURVE ( 'NONE', #1147, #23584, #21284, .T. ) ;
#22713=CARTESIAN_POINT ( 'NONE',  ( -19.75759631649036407, 3.218781778493905676, 7.359006845440219102 ) ) ;
#22714=CARTESIAN_POINT ( 'NONE',  ( 16.65022252850693363, 3.724077645907920342, 20.19593175699879595 ) ) ;
#22715=CIRCLE ( 'NONE', #18741, 0.7499999999999997780 ) ;
#22718=ORIENTED_EDGE ( 'NONE', *, *, #24457, .T. ) ;
#22719=LINE ( 'NONE', #3717, #8371 ) ;
#22723=AXIS2_PLACEMENT_3D ( 'NONE', #18443, #11246, #6422 ) ;
#22727=CARTESIAN_POINT ( 'NONE',  ( 2.703030265324084080, -12.75514121382991384, 1.500000000000001332 ) ) ;
#22728=CARTESIAN_POINT ( 'NONE',  ( 16.59873159789849595, 3.986191100139169663, 6.041646659195333058 ) ) ;
#22729=CARTESIAN_POINT ( 'NONE',  ( -15.33339156390900193, 12.86857621502489657, 18.34777357837152323 ) ) ;
#22731=CARTESIAN_POINT ( 'NONE',  ( -10.39981488257415698, -17.10438141112845400, 20.33971507717571114 ) ) ;
#22734=CARTESIAN_POINT ( 'NONE',  ( -9.225205623801109311, -14.30976465324222957, 6.031926333436658183 ) ) ;
#22737=EDGE_CURVE ( 'NONE', #7773, #6035, #21749, .T. ) ;
#22744=CARTESIAN_POINT ( 'NONE',  ( 11.40980092660686118, 6.310027164379057751, 1.500000000000001332 ) ) ;
#22746=CARTESIAN_POINT ( 'NONE',  ( -5.460567910819449366, 19.25894470870317221, 5.796888747622817029 ) ) ;
#22749=VECTOR ( 'NONE', #28151, 1000.000000000000000 ) ;
#22750=CARTESIAN_POINT ( 'NONE',  ( -15.26435939152463384, 8.070345032481604619, 1.500000000000000000 ) ) ;
#22751=VECTOR ( 'NONE', #19284, 1000.000000000000000 ) ;
#22755=CARTESIAN_POINT ( 'NONE',  ( 12.35522127307955920, 11.74279147895036068, 5.652196082364320695 ) ) ;
#22757=EDGE_LOOP ( 'NONE', ( #1324, #6441, #4370, #10076 ) ) ;
#22758=CIRCLE ( 'NONE', #24251, 0.7500000000000004441 ) ;
#22759=CARTESIAN_POINT ( 'NONE',  ( 15.18428249823343457, 13.04421712177833470, 5.749228751562096562 ) ) ;
#22766=ORIENTED_EDGE ( 'NONE', *, *, #14529, .T. ) ;
#22767=CARTESIAN_POINT ( 'NONE',  ( 3.623302445573600039, 16.66947753447049863, 7.559636331181775581 ) ) ;
#22770=CARTESIAN_POINT ( 'NONE',  ( 6.262360769054551746, 18.99428434097456631, 19.47728749465737863 ) ) ;
#22771=VECTOR ( 'NONE', #9088, 1000.000000000000000 ) ;
#22773=CIRCLE ( 'NONE', #9330, 1.000000000000010436 ) ;
#22775=CARTESIAN_POINT ( 'NONE',  ( 10.75049709165479683, -16.88611404641621405, 18.44501272782439827 ) ) ;
#22776=CARTESIAN_POINT ( 'NONE',  ( 16.86235748570415183, 2.342382300094908665, 19.87181966307587544 ) ) ;
#22779=CARTESIAN_POINT ( 'NONE',  ( -19.74495986540963699, 3.294819794740639463, 19.96783386855779341 ) ) ;
#22780=CARTESIAN_POINT ( 'NONE',  ( 18.35115206909799923, -7.996681782469499566, 7.652108011868850035 ) ) ;
#22782=FACE_OUTER_BOUND ( 'NONE', #12114, .T. ) ;
#22783=CARTESIAN_POINT ( 'NONE',  ( 3.269395338272003126, 16.75466097144276034, 18.73743063545763121 ) ) ;
#22786=CIRCLE ( 'NONE', #1381, 0.7500000000000006661 ) ;
#22789=CARTESIAN_POINT ( 'NONE',  ( -5.048943207435891978, 19.37072948160042429, 19.66989035740801839 ) ) ;
#22799=EDGE_LOOP ( 'NONE', ( #24582, #5504, #2802, #1866 ) ) ;
#22802=CARTESIAN_POINT ( 'NONE',  ( 5.881244434206234217, 6.812559277181991391, 1.500000000000001332 ) ) ;
#22805=CARTESIAN_POINT ( 'NONE',  ( -19.75724448635271457, 3.108068420208399907, 5.849008070840541862 ) ) ;
#22809=ORIENTED_EDGE ( 'NONE', *, *, #1089, .T. ) ;
#22816=DIRECTION ( 'NONE',  ( 0.000000000000000000, 0.000000000000000000, -1.000000000000000000 ) ) ;
#22820=VERTEX_POINT ( 'NONE', #5384 ) ;
#22822=AXIS2_PLACEMENT_3D ( 'NONE', #24967, #25440, #15928 ) ;
#22824=CARTESIAN_POINT ( 'NONE',  ( -6.055745631507628346, 15.95075576291064756, 7.500147780736496017 ) ) ;
#22834=DIRECTION ( 'NONE',  ( -0.9096319953545185522, 0.4154150130018859355, 0.000000000000000000 ) ) ;
#22836=CARTESIAN_POINT ( 'NONE',  ( -2.555255504830902691, 9.131494062835640690, 21.50000000000000000 ) ) ;
#22838=CARTESIAN_POINT ( 'NONE',  ( -8.546421330728135146, -14.74799399454104432, 5.652196082367002994 ) ) ;
#22843=CARTESIAN_POINT ( 'NONE',  ( -8.325649706210086265, -14.88445757357571786, 20.34789198813115618 ) ) ;
#22845=CARTESIAN_POINT ( 'NONE',  ( 19.59736455876166517, 3.994007928088045389, 18.73377938172348678 ) ) ;
#22852=CARTESIAN_POINT ( 'NONE',  ( 16.59792644105115755, 3.991267606926847122, 7.269896094239229889 ) ) ;
#22853=CARTESIAN_POINT ( 'NONE',  ( 0.6218383925729463746, -19.99069893758406735, 18.37545668562167478 ) ) ;
#22855=CARTESIAN_POINT ( 'NONE',  ( -17.02473723649752557, 1.129071356226221345, 7.545655578832111132 ) ) ;
#22858=CARTESIAN_POINT ( 'NONE',  ( -15.16307827826492627, -7.786259562520722710, 5.652196082368482699 ) ) ;
#22861=DIRECTION ( 'NONE',  ( 0.000000000000000000, 0.000000000000000000, 1.000000000000000000 ) ) ;
#22869=CIRCLE ( 'NONE', #9433, 1.000000000000000888 ) ;
#22875=CARTESIAN_POINT ( 'NONE',  ( -16.92089108241427198, 1.982400079378045410, 5.701226463332907279 ) ) ;
#22876=FACE_OUTER_BOUND ( 'NONE', #26204, .T. ) ;
#22877=CARTESIAN_POINT ( 'NONE',  ( -11.82521593960875528, 5.400395169024524655, 1.500000000000001332 ) ) ;
#22882=ADVANCED_FACE ( 'NONE', ( #26603 ), #20093, .T. ) ;
#22883=CARTESIAN_POINT ( 'NONE',  ( 0.3567147238643512130, -19.99681861211370659, 5.652196082369963293 ) ) ;
#22884=CARTESIAN_POINT ( 'NONE',  ( -16.94912694327470959, 1.778434105053336545, 18.34727598691068096 ) ) ;
#22886=DIRECTION ( 'NONE',  ( 1.000000000000000000, 0.000000000000000000, 0.000000000000000000 ) ) ;
#22887=CARTESIAN_POINT ( 'NONE',  ( -5.352643706120517209, -7.827050521741861999, 1.500000000000001332 ) ) ;
#22889=ADVANCED_FACE ( 'NONE', ( #1318 ), #15347, .F. ) ;
#22893=CARTESIAN_POINT ( 'NONE',  ( -19.94516883457951550, 1.701953382846944196, 18.73743063545763121 ) ) ;
#22902=CARTESIAN_POINT ( 'NONE',  ( -15.66719571743413475, 12.43196305300237903, 5.779535427900761135 ) ) ;
#22903=CARTESIAN_POINT ( 'NONE',  ( -4.775770841707820402, 16.34206821731734038, 7.272049892295485485 ) ) ;
#22906=CARTESIAN_POINT ( 'NONE',  ( -13.21131958021091179, 10.75991052173262474, 5.676815824193226945 ) ) ;
#22909=ORIENTED_EDGE ( 'NONE', *, *, #3618, .F. ) ;
#22911=EDGE_CURVE ( 'NONE', #29885, #18473, #21432, .T. ) ;
#22912=CARTESIAN_POINT ( 'NONE',  ( 15.41296542101254552, 5.939519782021115191, 1.500000000000000000 ) ) ;
#22916=VERTEX_POINT ( 'NONE', #7836 ) ;
#22923=ADVANCED_FACE ( 'NONE', ( #24513 ), #13899, .T. ) ;
#22925=CARTESIAN_POINT ( 'NONE',  ( 3.424309912165884207, 16.71834993634870159, 5.872146474157316831 ) ) ;
#22928=ORIENTED_EDGE ( 'NONE', *, *, #16048, .F. ) ;
#22929=CARTESIAN_POINT ( 'NONE',  ( 19.89647750965486495, 2.201534687727671802, 19.22654678686458141 ) ) ;
#22932=CARTESIAN_POINT ( 'NONE',  ( 17.93426220341855526, -8.892634148397206673, 6.420335371522007506 ) ) ;
#22933=CARTESIAN_POINT ( 'NONE',  ( -13.66451197432776432, 10.21236830578559562, 5.749491821935610147 ) ) ;
#22934=CARTESIAN_POINT ( 'NONE',  ( 4.313865120791887442, 19.54726060313607050, 19.25672174529527325 ) ) ;
#22936=EDGE_LOOP ( 'NONE', ( #26031, #10085, #8722, #24042 ) ) ;
#22940=CARTESIAN_POINT ( 'NONE',  ( 15.05429537369196069, 13.16750578773771352, 18.37250658438899009 ) ) ;
#22941=CARTESIAN_POINT ( 'NONE',  ( -4.568010850242215426, 16.39675899511904689, 19.33715507985239412 ) ) ;
#22942=DIRECTION ( 'NONE',  ( 0.000000000000000000, 0.000000000000000000, 1.000000000000000000 ) ) ;
#22943=CYLINDRICAL_SURFACE ( 'NONE', #14095, 20.00000000000000355 ) ;
#22951=FACE_OUTER_BOUND ( 'NONE', #24009, .T. ) ;
#22954=CARTESIAN_POINT ( 'NONE',  ( -19.82747825358060467, 2.624647641736344461, 5.651480102388687143 ) ) ;
#22957=ORIENTED_EDGE ( 'NONE', *, *, #3164, .F. ) ;
#22958=CARTESIAN_POINT ( 'NONE',  ( 0.2207535014603130841, -19.99921160563567923, 7.652108011868850923 ) ) ;
#22961=CARTESIAN_POINT ( 'NONE',  ( 0.000000000000000000, 0.000000000000000000, 21.50000000000000000 ) ) ;
#22962=CARTESIAN_POINT ( 'NONE',  ( -6.193882932557621679, 19.03538945389874470, 18.37415474056476938 ) ) ;
#22964=CARTESIAN_POINT ( 'NONE',  ( 1.638502901550993540, -16.99392728441680234, 7.196036389296800451 ) ) ;
#22969=CARTESIAN_POINT ( 'NONE',  ( -5.544451646083596863, 16.11829163520482311, 7.652108011868850035 ) ) ;
#22974=CARTESIAN_POINT ( 'NONE',  ( -5.604556300746500241, -15.53790034020399169, 1.500000000000000000 ) ) ;
#22976=DIRECTION ( 'NONE',  ( -0.000000000000000000, -0.000000000000000000, 1.000000000000000000 ) ) ;
#22980=CARTESIAN_POINT ( 'NONE',  ( 8.499586724479435418, 2.959227181723830036, 1.500000000000001332 ) ) ;
#22984=FACE_OUTER_BOUND ( 'NONE', #5031, .T. ) ;
#22991=CARTESIAN_POINT ( 'NONE',  ( -8.546421331151641709, -14.74799399427946689, 5.652196082364321583 ) ) ;
#22996=CARTESIAN_POINT ( 'NONE',  ( 7.730328572437743517, -4.608906612435629491, 21.50000000000000000 ) ) ;
#23000=CARTESIAN_POINT ( 'NONE',  ( -15.49859937932966680, -7.047316568154765370, 19.96344307082652847 ) ) ;
#23015=CARTESIAN_POINT ( 'NONE',  ( 9.860909914091285700, -13.90333503830274253, 20.34789198813115263 ) ) ;
#23016=EDGE_LOOP ( 'NONE', ( #11609, #6025, #20049, #1216 ) ) ;
#23017=ORIENTED_EDGE ( 'NONE', *, *, #10693, .T. ) ;
#23018=CARTESIAN_POINT ( 'NONE',  ( -16.96555893295483841, 1.647560171216676750, 5.652196082367002106 ) ) ;
#23022=VERTEX_POINT ( 'NONE', #18446 ) ;
#23027=CARTESIAN_POINT ( 'NONE',  ( -14.71622834325375351, -8.664216105401095547, 6.917457548096559883 ) ) ;
#23028=DIRECTION ( 'NONE',  ( 1.000000000000000000, 0.000000000000000000, 0.000000000000000000 ) ) ;
#23035=CARTESIAN_POINT ( 'NONE',  ( -19.95549607358725908, 1.576375212833064143, 18.92976555901915603 ) ) ;
#23040=ORIENTED_EDGE ( 'NONE', *, *, #30760, .F. ) ;
#23042=VECTOR ( 'NONE', #29926, 1000.000000000000000 ) ;
#23043=CARTESIAN_POINT ( 'NONE',  ( 10.89102995336899937, -16.77499580993352524, 5.676722608126683944 ) ) ;
#23044=EDGE_CURVE ( 'NONE', #4677, #25657, #19380, .T. ) ;
#23048=CARTESIAN_POINT ( 'NONE',  ( 5.738360882149951436, 7.548823014270661602, 1.500000000000001332 ) ) ;
#23052=ORIENTED_EDGE ( 'NONE', *, *, #29404, .F. ) ;
#23058=DIRECTION ( 'NONE',  ( 1.000000000000000000, 0.000000000000000000, 0.000000000000000000 ) ) ;
#23061=CARTESIAN_POINT ( 'NONE',  ( -18.06093776605887058, -8.632162463936113639, 7.652108011868850035 ) ) ;
#23062=VECTOR ( 'NONE', #28399, 1000.000000000000000 ) ;
#23064=DIRECTION ( 'NONE',  ( -0.000000000000000000, -0.000000000000000000, 1.000000000000000000 ) ) ;
#23066=EDGE_CURVE ( 'NONE', #20277, #160, #13902, .T. ) ;
#23071=VERTEX_POINT ( 'NONE', #27949 ) ;
#23074=CARTESIAN_POINT ( 'NONE',  ( 15.47797589786117634, -7.092492006142043337, 7.272049892295485485 ) ) ;
#23075=CARTESIAN_POINT ( 'NONE',  ( -13.92530307126622269, 9.878387810998201957, 6.131018562779544823 ) ) ;
#23076=CARTESIAN_POINT ( 'NONE',  ( 3.146565092309292933, 16.78275473100423554, 18.92976555901915603 ) ) ;
#23077=ORIENTED_EDGE ( 'NONE', *, *, #14740, .T. ) ;
#23080=EDGE_CURVE ( 'NONE', #681, #14465, #7297, .T. ) ;
#23083=B_SPLINE_SURFACE_WITH_KNOTS ( 'NONE', 3, 1, ( 
 ( #23610, #20965 ),
 ( #6637, #9448 ),
 ( #25669, #13818 ),
 ( #2253, #6950 ),
 ( #27866, #20669 ),
 ( #30191, #28324 ),
 ( #6784, #11773 ),
 ( #23320, #25521 ),
 ( #16307, #11482 ),
 ( #13674, #23158 ),
 ( #30489, #11328 ),
 ( #21274, #20825 ),
 ( #8989, #18504 ),
 ( #28006, #18650 ),
 ( #4458, #13966 ),
 ( #23464, #11625 ),
 ( #24233, #22050 ),
 ( #19712, #19566 ),
 ( #9739, #26747 ),
 ( #531, #19415 ),
 ( #225, #21903 ),
 ( #29083, #16921 ),
 ( #7877, #17384 ),
 ( #26436, #2578 ),
 ( #7724, #14250 ),
 ( #12238, #17223 ),
 ( #2885, #14582 ),
 ( #19105, #21741 ),
 ( #24084, #9595 ),
 ( #19251, #28774 ),
 ( #17071, #23769 ) ),
 .UNSPECIFIED., .F., .F., .F.,
 ( 4, 3, 3, 3, 3, 3, 3, 3, 3, 3, 4 ),
 ( 2, 2 ),
 ( 0.000000000000000000, 0.05425176834609614362, 0.1085332949128348518, 0.1623767749169379715, 0.2157504826133058717, 0.2688657508888169789, 0.3218907763505471364, 0.3749548578363334772, 0.4282048033836237666, 0.4818374082110496448, 0.4999999999131651274 ),
 ( 0.000000000000000000, 1.000000000000000000 ),
 .UNSPECIFIED. ) ;
#23085=LINE ( 'NONE', #3723, #21246 ) ;
#23087=CARTESIAN_POINT ( 'NONE',  ( 12.00027744587103840, 12.12900492888020665, 5.759928666072752890 ) ) ;
#23089=AXIS2_PLACEMENT_3D ( 'NONE', #13065, #29907, #8689 ) ;
#23094=CARTESIAN_POINT ( 'NONE',  ( 1.236176367852860336, -19.96182836857062171, 7.161525567826881655 ) ) ;
#23095=EDGE_CURVE ( 'NONE', #14352, #12655, #4996, .T. ) ;
#23097=DIRECTION ( 'NONE',  ( 1.000000000000000000, 0.000000000000000000, 0.000000000000000000 ) ) ;
#23100=CARTESIAN_POINT ( 'NONE',  ( -4.163336342344337027E-14, 1.387778780781445676E-14, 24.50000000000000000 ) ) ;
#23102=DIRECTION ( 'NONE',  ( -0.000000000000000000, -0.000000000000000000, 1.000000000000000000 ) ) ;
#23105=CARTESIAN_POINT ( 'NONE',  ( 0.3518703668723787148, -19.99690444156084723, 7.652108011868850035 ) ) ;
#23110=DIRECTION ( 'NONE',  ( 0.000000000000000000, 0.000000000000000000, 1.000000000000000000 ) ) ;
#23111=CARTESIAN_POINT ( 'NONE',  ( 1.342146863054722639, -19.97260970722469509, 6.892848776733236704 ) ) ;
#23114=ORIENTED_EDGE ( 'NONE', *, *, #17973, .T. ) ;
#23118=CYLINDRICAL_SURFACE ( 'NONE', #30216, 9.482273699623480212 ) ;
#23120=VERTEX_POINT ( 'NONE', #13108 ) ;
#23122=CARTESIAN_POINT ( 'NONE',  ( -17.73231296732453188, -9.288543855440106967, 18.64703902303423178 ) ) ;
#23124=EDGE_CURVE ( 'NONE', #24186, #466, #5766, .T. ) ;
#23125=( NAMED_UNIT ( * ) PLANE_ANGLE_UNIT ( ) SI_UNIT ( $, .RADIAN. ) );
#23127=EDGE_LOOP ( 'NONE', ( #6741, #20467, #28867, #13127 ) ) ;
#23128=CARTESIAN_POINT ( 'NONE',  ( 7.562559277181973627, -5.881244434206257310, 1.500000000000001332 ) ) ;
#23142=EDGE_CURVE ( 'NONE', #18090, #7470, #24357, .T. ) ;
#23143=CARTESIAN_POINT ( 'NONE',  ( -10.32985675426555616, -17.14655349859504341, 5.678370764302467677 ) ) ;
#23146=DIRECTION ( 'NONE',  ( 0.000000000000000000, 0.000000000000000000, 1.000000000000000000 ) ) ;
#23147=VERTEX_POINT ( 'NONE', #8267 ) ;
#23148=DIRECTION ( 'NONE',  ( 0.7557495743542582689, -0.6548607339452849896, 0.000000000000000000 ) ) ;
#23149=CARTESIAN_POINT ( 'NONE',  ( 16.55530288949897866, 4.194058762902721504, 6.783738457429058677 ) ) ;
#23153=CARTESIAN_POINT ( 'NONE',  ( -12.84881549446081017, 11.17046077483154853, 19.96344307082653202 ) ) ;
#23156=CARTESIAN_POINT ( 'NONE',  ( 3.188743458504121442, 16.77324615162856958, 18.84329447212444464 ) ) ;
#23158=CARTESIAN_POINT ( 'NONE',  ( -15.51938817160314876, -6.998174447281577670, 19.87181966307587544 ) ) ;
#23163=DIRECTION ( 'NONE',  ( 1.000000000000000000, 0.000000000000000000, 0.000000000000000000 ) ) ;
#23166=CARTESIAN_POINT ( 'NONE',  ( -6.312773474853920597, 15.86096687809345696, 19.96568007040468729 ) ) ;
#23168=ORIENTED_EDGE ( 'NONE', *, *, #18702, .T. ) ;
#23170=CARTESIAN_POINT ( 'NONE',  ( -10.82521593960875528, 5.400395169024524655, 1.500000000000001332 ) ) ;
#23173=DIRECTION ( 'NONE',  ( 1.000000000000000000, 0.000000000000000000, 0.000000000000000000 ) ) ;
#23176=CARTESIAN_POINT ( 'NONE',  ( -15.16307827826492627, -7.786259562520722710, 5.652196082368482699 ) ) ;
#23178=EDGE_CURVE ( 'NONE', #3110, #2473, #2975, .T. ) ;
#23179=EDGE_LOOP ( 'NONE', ( #25430, #28968, #5198, #14080 ) ) ;
#23184=CARTESIAN_POINT ( 'NONE',  ( 19.74942470869275368, 3.267558643021993170, 7.652108011868850035 ) ) ;
#23186=DIRECTION ( 'NONE',  ( 1.000000000000000000, 0.000000000000000000, 0.000000000000000000 ) ) ;
#23187=CARTESIAN_POINT ( 'NONE',  ( -17.05026832885478072, 0.8441673869077329639, 18.73314399819311760 ) ) ;
#23188=CARTESIAN_POINT ( 'NONE',  ( 3.196529495465388226, 8.413215745755008967, 1.500000000000001332 ) ) ;
#23190=CARTESIAN_POINT ( 'NONE',  ( 9.984725267469515941, -13.82013960671582531, 20.33971507717571114 ) ) ;
#23191=DIRECTION ( 'NONE',  ( -0.000000000000000000, -0.000000000000000000, 1.000000000000000000 ) ) ;
#23192=ORIENTED_EDGE ( 'NONE', *, *, #8469, .F. ) ;
#23193=VERTEX_POINT ( 'NONE', #15424 ) ;
#23196=DIRECTION ( 'NONE',  ( -0.000000000000000000, -0.000000000000000000, 1.000000000000000000 ) ) ;
#23200=CARTESIAN_POINT ( 'NONE',  ( -12.97606618380807220, 11.02883152178847936, 5.848946451764558851 ) ) ;
#23202=B_SPLINE_CURVE_WITH_KNOTS ( 'NONE', 3,
 ( #1279, #8750, #15612, #4373, #9062, #20303, #16081, #23232, #20594, #11409, #15770, #30425, #1886, #3936, #13456, #25451 ),
 .UNSPECIFIED., .F., .F.,
 ( 4, 2, 2, 2, 2, 2, 2, 4 ),
 ( 0.4999999999999997224, 0.6249999999999995559, 0.6874999999999995559, 0.7187499999999995559, 0.7499999999999995559, 0.8124999999999995559, 0.8749999999999997780, 1.000000000000000000 ),
 .UNSPECIFIED. ) ;
#23206=ORIENTED_EDGE ( 'NONE', *, *, #10926, .F. ) ;
#23211=ORIENTED_EDGE ( 'NONE', *, *, #19086, .T. ) ;
#23214=EDGE_CURVE ( 'NONE', #27034, #26243, #24361, .T. ) ;
#23216=LINE ( 'NONE', #16673, #10096 ) ;
#23218=AXIS2_PLACEMENT_3D ( 'NONE', #28598, #4579, #16735 ) ;
#23220=CARTESIAN_POINT ( 'NONE',  ( 9.411519254647286559, -14.19511874370440907, 18.49267272388512140 ) ) ;
#23221=CARTESIAN_POINT ( 'NONE',  ( 16.87696675355429576, 2.215034284604904702, 19.11611934778430921 ) ) ;
#23223=CARTESIAN_POINT ( 'NONE',  ( -19.75759631649036763, 3.218781778493906121, 20.05479082170252525 ) ) ;
#23224=CARTESIAN_POINT ( 'NONE',  ( 15.59193442375635819, -6.853442328767825664, 5.796888747622817029 ) ) ;
#23225=CARTESIAN_POINT ( 'NONE',  ( -15.98876933090331498, 12.04425525511917527, 6.560937769032974209 ) ) ;
#23227=CARTESIAN_POINT ( 'NONE',  ( 1.000000000000008438, 15.73749217771910125, 24.50000000000000000 ) ) ;
#23230=VERTEX_POINT ( 'NONE', #26995 ) ;
#23232=CARTESIAN_POINT ( 'NONE',  ( 10.68714603012076303, -13.32085008213842769, 6.521906765011492801 ) ) ;
#23233=CARTESIAN_POINT ( 'NONE',  ( 12.98116905408885557, 11.01127998641985428, 6.973843882838225205 ) ) ;
#23242=CARTESIAN_POINT ( 'NONE',  ( -19.95735252415838445, 1.552219945263930700, 6.995624166085161910 ) ) ;
#23244=CARTESIAN_POINT ( 'NONE',  ( -6.630478080506954974, -6.778663211761442930, 1.500000000000001332 ) ) ;
#23251=DIRECTION ( 'NONE',  ( -0.4154150130018840481, 0.9096319953545194403, 0.000000000000000000 ) ) ;
#23252=AXIS2_PLACEMENT_3D ( 'NONE', #23848, #16842, #7017 ) ;
#23254=VERTEX_POINT ( 'NONE', #22599 ) ;
#23255=CARTESIAN_POINT ( 'NONE',  ( -0.2664633505551967652, -19.99844781589863274, 7.454139397117730326 ) ) ;
#23256=EDGE_CURVE ( 'NONE', #8747, #8832, #19494, .T. ) ;
#23258=EDGE_CURVE ( 'NONE', #14232, #5725, #25256, .T. ) ;
#23264=CARTESIAN_POINT ( 'NONE',  ( -18.04365185506138047, -8.627086862512674870, 20.34789198813115263 ) ) ;
#23266=EDGE_CURVE ( 'NONE', #15211, #21613, #9038, .T. ) ;
#23269=EDGE_CURVE ( 'NONE', #20491, #12536, #22869, .T. ) ;
#23275=CARTESIAN_POINT ( 'NONE',  ( -17.66624025659153574, -9.413543259203217772, 18.82680253904184298 ) ) ;
#23280=VECTOR ( 'NONE', #17569, 1000.000000000000000 ) ;
#23281=ORIENTED_EDGE ( 'NONE', *, *, #10695, .F. ) ;
#23283=CARTESIAN_POINT ( 'NONE',  ( 11.40980092660686118, 6.310027164379057751, 24.50000000000000000 ) ) ;
#23287=DIRECTION ( 'NONE',  ( 0.000000000000000000, 0.000000000000000000, 1.000000000000000000 ) ) ;
#23289=DIRECTION ( 'NONE',  ( 1.000000000000000000, 0.000000000000000000, 0.000000000000000000 ) ) ;
#23290=DIRECTION ( 'NONE',  ( 1.000000000000000000, 0.000000000000000000, 0.000000000000000000 ) ) ;
#23292=EDGE_CURVE ( 'NONE', #19042, #17054, #19898, .T. ) ;
#23305=VECTOR ( 'NONE', #20249, 1000.000000000000000 ) ;
#23306=ORIENTED_EDGE ( 'NONE', *, *, #1089, .F. ) ;
#23309=CARTESIAN_POINT ( 'NONE',  ( 16.65321191609847418, 3.713086718183620683, 7.545655578832111132 ) ) ;
#23310=CARTESIAN_POINT ( 'NONE',  ( -10.47960520055065636, -7.757439966934454034, 1.500000000000001332 ) ) ;
#23311=CARTESIAN_POINT ( 'NONE',  ( -13.33237335330699125, 10.61702797731129877, 18.34969686940296185 ) ) ;
#23315=CARTESIAN_POINT ( 'NONE',  ( -14.44122519041009234, -13.83658248990211348, 24.50000000000000000 ) ) ;
#23320=CARTESIAN_POINT ( 'NONE',  ( -18.36135251343598185, -7.973951480934446501, 20.05479082170252525 ) ) ;
#23322=ORIENTED_EDGE ( 'NONE', *, *, #29812, .T. ) ;
#23324=LINE ( 'NONE', #11487, #2000 ) ;
#23329=AXIS2_PLACEMENT_3D ( 'NONE', #16449, #30477, #30337 ) ;
#23331=CARTESIAN_POINT ( 'NONE',  ( 18.09058649146511044, -8.570415951004784816, 18.55820869691756769 ) ) ;
#23334=ORIENTED_EDGE ( 'NONE', *, *, #127, .F. ) ;
#23335=DIRECTION ( 'NONE',  ( -0.000000000000000000, -0.000000000000000000, 1.000000000000000000 ) ) ;
#23337=VECTOR ( 'NONE', #86, 1000.000000000000000 ) ;
#23340=CARTESIAN_POINT ( 'NONE',  ( -8.549050687778191104, -4.102102735472429096, 21.50000000000000000 ) ) ;
#23345=ORIENTED_EDGE ( 'NONE', *, *, #18174, .T. ) ;
#23350=PRODUCT_DEFINITION_SHAPE ( 'NONE', 'NONE',  #12777 ) ;
#23354=DIRECTION ( 'NONE',  ( 0.000000000000000000, 0.000000000000000000, 1.000000000000000000 ) ) ;
#23355=CARTESIAN_POINT ( 'NONE',  ( -16.99143801116384722, 1.432169416036907617, 20.32367522806703874 ) ) ;
#23356=CARTESIAN_POINT ( 'NONE',  ( -12.54846374865995706, -9.550116103605043705, 24.50000000000000000 ) ) ;
#23358=CARTESIAN_POINT ( 'NONE',  ( 4.622016212553096359, -12.19167610014704906, 1.500000000000001332 ) ) ;
#23367=VECTOR ( 'NONE', #30605, 1000.000000000000000 ) ;
#23368=CARTESIAN_POINT ( 'NONE',  ( -12.79825419737478676, 11.22575876280636642, 7.156916968540300239 ) ) ;
#23370=ORIENTED_EDGE ( 'NONE', *, *, #20075, .F. ) ;
#23379=AXIS2_PLACEMENT_3D ( 'NONE', #9874, #22026, #9563 ) ;
#23385=DIRECTION ( 'NONE',  ( 0.000000000000000000, 0.000000000000000000, 1.000000000000000000 ) ) ;
#23386=CARTESIAN_POINT ( 'NONE',  ( -6.187077094091591789, 11.47693674426096955, 1.500000000000001332 ) ) ;
#23388=CARTESIAN_POINT ( 'NONE',  ( 10.65605551513794502, -16.94611923951457655, 7.500898271101006820 ) ) ;
#23391=CARTESIAN_POINT ( 'NONE',  ( 3.062389757841097904, 16.80148204205676876, 19.36813350477385143 ) ) ;
#23393=ORIENTED_EDGE ( 'NONE', *, *, #10139, .F. ) ;
#23396=CARTESIAN_POINT ( 'NONE',  ( -5.655446062488476144, 19.20259930434394846, 18.39701043959520987 ) ) ;
#23402=ORIENTED_EDGE ( 'NONE', *, *, #8248, .F. ) ;
#23404=CARTESIAN_POINT ( 'NONE',  ( -19.86072491926578110, 2.502642356747510899, 7.652108011868850035 ) ) ;
#23406=CARTESIAN_POINT ( 'NONE',  ( 19.78395057425408865, 2.934310293824241356, 20.32243167357989577 ) ) ;
#23414=LINE ( 'NONE', #25075, #16822 ) ;
#23417=CARTESIAN_POINT ( 'NONE',  ( -6.460166075217649961, 15.80732207284229673, 19.03762469184452755 ) ) ;
#23418=LINE ( 'NONE', #2674, #24289 ) ;
#23421=CARTESIAN_POINT ( 'NONE',  ( 5.296161872597624942, 19.28602264385379428, 20.34789198813115263 ) ) ;
#23424=ORIENTED_EDGE ( 'NONE', *, *, #18763, .F. ) ;
#23428=ADVANCED_FACE ( 'NONE', ( #9794 ), #10898, .T. ) ;
#23434=CARTESIAN_POINT ( 'NONE',  ( -12.24063095261064227, 4.490763173670005770, 1.500000000000001332 ) ) ;
#23438=VERTEX_POINT ( 'NONE', #11000 ) ;
#23439=PLANE ( 'NONE',  #230 ) ;
#23440=CARTESIAN_POINT ( 'NONE',  ( 0.000000000000000000, 0.000000000000000000, 1.500000000000001332 ) ) ;
#23443=ORIENTED_EDGE ( 'NONE', *, *, #23256, .T. ) ;
#23444=FACE_OUTER_BOUND ( 'NONE', #30615, .T. ) ;
#23446=CARTESIAN_POINT ( 'NONE',  ( -7.759781818727213398, -15.20954222608249395, 7.098451512883313441 ) ) ;
#23448=CARTESIAN_POINT ( 'NONE',  ( 1.512395753140455934, -17.00118538373298804, 18.64703902303423178 ) ) ;
#23456=VECTOR ( 'NONE', #18225, 1000.000000000000000 ) ;
#23458=CARTESIAN_POINT ( 'NONE',  ( -12.97413174816959724, 11.03100730464097090, 20.14907003336613300 ) ) ;
#23462=ADVANCED_FACE ( 'NONE', ( #16432 ), #20797, .F. ) ;
#23463=ADVANCED_FACE ( 'NONE', ( #16131 ), #25947, .F. ) ;
#23464=CARTESIAN_POINT ( 'NONE',  ( -18.47028637364417136, -7.717842544976234009, 19.22654678686458141 ) ) ;
#23467=VERTEX_POINT ( 'NONE', #13941 ) ;
#23469=CARTESIAN_POINT ( 'NONE',  ( -7.786278744133511509, -15.19480685133639497, 7.158811349119585721 ) ) ;
#23474=CARTESIAN_POINT ( 'NONE',  ( -6.501324370946574227, 15.79217903278910740, 19.21769074125272780 ) ) ;
#23479=CARTESIAN_POINT ( 'NONE',  ( -10.62668044795003297, -16.94375577056504412, 20.34789198813115618 ) ) ;
#23481=CIRCLE ( 'NONE', #17530, 0.7500000000000002220 ) ;
#23482=LINE ( 'NONE', #9464, #6378 ) ;
#23484=ORIENTED_EDGE ( 'NONE', *, *, #17497, .F. ) ;
#23487=CARTESIAN_POINT ( 'NONE',  ( -15.05112753843571483, -8.020416455010169088, 7.652108011868853588 ) ) ;
#23489=ORIENTED_EDGE ( 'NONE', *, *, #7314, .F. ) ;
#23491=LINE ( 'NONE', #11650, #19257 ) ;
#23496=DIRECTION ( 'NONE',  ( 1.000000000000000000, 0.000000000000000000, 0.000000000000000000 ) ) ;
#23497=CARTESIAN_POINT ( 'NONE',  ( -19.91121867491064279, 2.064381093144386004, 20.25542030744407640 ) ) ;
#23498=DIRECTION ( 'NONE',  ( 1.000000000000000000, 0.000000000000000000, 0.000000000000000000 ) ) ;
#23500=ADVANCED_FACE ( 'NONE', ( #22984, #18938, #11599 ), #2230, .T. ) ;
#23501=EDGE_CURVE ( 'NONE', #23911, #6597, #9259, .T. ) ;
#23502=CARTESIAN_POINT ( 'NONE',  ( 10.50949999207124286, -13.45141484214874517, 19.97651184436794125 ) ) ;
#23505=ORIENTED_EDGE ( 'NONE', *, *, #26972, .T. ) ;
#23507=ORIENTED_EDGE ( 'NONE', *, *, #28866, .F. ) ;
#23508=CARTESIAN_POINT ( 'NONE',  ( -15.42727847259665452, 12.72856271945105888, 7.652108011868850923 ) ) ;
#23518=DIRECTION ( 'NONE',  ( -0.000000000000000000, -0.000000000000000000, 1.000000000000000000 ) ) ;
#23521=ORIENTED_EDGE ( 'NONE', *, *, #9078, .T. ) ;
#23527=CARTESIAN_POINT ( 'NONE',  ( -14.93254240682317047, -8.254432589069386594, 20.24143955528809613 ) ) ;
#23528=CIRCLE ( 'NONE', #9101, 0.7499999999999997780 ) ;
#23533=CARTESIAN_POINT ( 'NONE',  ( -16.96078254943347829, 1.685604580053747803, 18.34777357837152323 ) ) ;
#23534=CARTESIAN_POINT ( 'NONE',  ( 18.33777834721833955, -8.027392848387997049, 5.651989602109219746 ) ) ;
#23535=CARTESIAN_POINT ( 'NONE',  ( -13.47385700491362215, 10.44730466805193103, 7.643931100913408550 ) ) ;
#23536=DIRECTION ( 'NONE',  ( -0.000000000000000000, -0.000000000000000000, 1.000000000000000000 ) ) ;
#23539=LINE ( 'NONE', #2183, #24765 ) ;
#23540=CARTESIAN_POINT ( 'NONE',  ( -19.84404562991029763, 2.492760124447686465, 5.652196082369965069 ) ) ;
#23546=CARTESIAN_POINT ( 'NONE',  ( -19.96222469201676475, 1.488090962520939531, 6.560937769032974209 ) ) ;
#23547=CARTESIAN_POINT ( 'NONE',  ( 14.53509801925589784, 13.73847344395387005, 18.47531940416306284 ) ) ;
#23549=ORIENTED_EDGE ( 'NONE', *, *, #17100, .T. ) ;
#23555=CARTESIAN_POINT ( 'NONE',  ( 8.499586724479435418, 2.959227181723830036, 1.500000000000001332 ) ) ;
#23561=CARTESIAN_POINT ( 'NONE',  ( -6.403603917672689327, 18.96607824920917906, 18.44527579819791185 ) ) ;
#23562=EDGE_CURVE ( 'NONE', #25305, #24319, #4266, .T. ) ;
#23563=CARTESIAN_POINT ( 'NONE',  ( 11.64054540341803978, 16.26338533980433709, 24.50000000000000000 ) ) ;
#23567=CARTESIAN_POINT ( 'NONE',  ( 15.81416692036122917, -6.360574302898113430, 5.652196082368483587 ) ) ;
#23573=AXIS2_PLACEMENT_3D ( 'NONE', #29786, #16044, #30395 ) ;
#23574=CARTESIAN_POINT ( 'NONE',  ( -14.70423443302405708, -8.686234331489295357, 19.47783254395485031 ) ) ;
#23580=CARTESIAN_POINT ( 'NONE',  ( -4.163336342344337027E-14, 1.387778780781445676E-14, 24.50000000000000000 ) ) ;
#23584=VERTEX_POINT ( 'NONE', #30167 ) ;
#23591=PRODUCT ( 'Rotor', 'Rotor', '', ( #15039 ) ) ;
#23593=CARTESIAN_POINT ( 'NONE',  ( -0.6524377400371712543, -20.00727110999511993, 19.22654678686458141 ) ) ;
#23595=CARTESIAN_POINT ( 'NONE',  ( -9.736160311572508164, -17.49040459468424658, 7.098451512883313441 ) ) ;
#23596=CARTESIAN_POINT ( 'NONE',  ( 8.413215745754998309, -3.196529495465417980, 1.500000000000001332 ) ) ;
#23597=CARTESIAN_POINT ( 'NONE',  ( 0.4236634240584221112, -20.01342612130735787, 20.34789198813115263 ) ) ;
#23598=ORIENTED_EDGE ( 'NONE', *, *, #11452, .T. ) ;
#23600=CARTESIAN_POINT ( 'NONE',  ( -13.00999358272542494, -0.8602714556717691030, 1.500000000000001332 ) ) ;
#23601=CARTESIAN_POINT ( 'NONE',  ( 14.59199839715918046, 13.70371665158259944, 18.44527579819791185 ) ) ;
#23605=CARTESIAN_POINT ( 'NONE',  ( -15.34307810681595896, 12.82926163924266660, 7.652108011868850035 ) ) ;
#23606=DIRECTION ( 'NONE',  ( 1.000000000000000000, 0.000000000000000000, 0.000000000000000000 ) ) ;
#23608=DIRECTION ( 'NONE',  ( 1.000000000000000000, 0.000000000000000000, 0.000000000000000000 ) ) ;
#23609=CARTESIAN_POINT ( 'NONE',  ( 9.163215745754998309, -3.196529495465417980, 1.500000000000001332 ) ) ;
#23610=CARTESIAN_POINT ( 'NONE',  ( -18.06093776605888479, -8.632162463936117192, 20.34789198813115263 ) ) ;
#23612=ORIENTED_EDGE ( 'NONE', *, *, #4209, .T. ) ;
#23615=AXIS2_PLACEMENT_3D ( 'NONE', #20567, #8724, #18239 ) ;
#23618=DIRECTION ( 'NONE',  ( 1.000000000000000000, 0.000000000000000000, 0.000000000000000000 ) ) ;
#23621=CARTESIAN_POINT ( 'NONE',  ( 17.93426220341855171, -8.892634148397208449, 19.11611934778430921 ) ) ;
#23622=CARTESIAN_POINT ( 'NONE',  ( 5.913643690471324987, 19.12442985200254597, 7.429667576816606278 ) ) ;
#23623=ORIENTED_EDGE ( 'NONE', *, *, #25043, .F. ) ;
#23625=CARTESIAN_POINT ( 'NONE',  ( 14.79741041486972541, 13.48156734445487714, 7.643931100913408550 ) ) ;
#23629=PLANE ( 'NONE',  #10859 ) ;
#23630=EDGE_CURVE ( 'NONE', #6239, #26662, #25800, .T. ) ;
#23635=CARTESIAN_POINT ( 'NONE',  ( -15.53738272950673682, -6.955830428693971612, 6.211014596808754007 ) ) ;
#23639=EDGE_CURVE ( 'NONE', #8694, #24029, #16931, .T. ) ;
#23642=CARTESIAN_POINT ( 'NONE',  ( 5.524309650260767590, -7.706848733600972778, 13.00000000000000178 ) ) ;
#23643=CARTESIAN_POINT ( 'NONE',  ( -17.03429152191316831, 1.023117790763816037, 20.13759033520874908 ) ) ;
#23644=DIRECTION ( 'NONE',  ( 0.1423148382732746797, -0.9898214418809342385, 0.000000000000000000 ) ) ;
#23646=ADVANCED_FACE ( 'NONE', ( #14555 ), #26245, .F. ) ;
#23647=CARTESIAN_POINT ( 'NONE',  ( 11.39002951368468430, -16.46174851469274003, 20.29915277494337644 ) ) ;
#23649=ADVANCED_FACE ( 'NONE', ( #7698 ), #5347, .F. ) ;
#23654=ORIENTED_EDGE ( 'NONE', *, *, #30356, .F. ) ;
#23659=ORIENTED_EDGE ( 'NONE', *, *, #3451, .F. ) ;
#23660=CARTESIAN_POINT ( 'NONE',  ( 18.72527277698615222, -7.076062192109020543, 19.58863275299554019 ) ) ;
#23661=CARTESIAN_POINT ( 'NONE',  ( 16.55532831589957254, 4.193940174973931789, 19.36813350477385143 ) ) ;
#23663=VERTEX_POINT ( 'NONE', #21711 ) ;
#23664=CARTESIAN_POINT ( 'NONE',  ( 12.37236664230077743, -12.04390635323149716, -0.6213203435596476032 ) ) ;
#23665=ADVANCED_FACE ( 'NONE', ( #19222 ), #10177, .F. ) ;
#23679=EDGE_CURVE ( 'NONE', #115, #25416, #23907, .T. ) ;
#23680=CARTESIAN_POINT ( 'NONE',  ( -19.80175191879421703, 2.933369436805208785, 18.44501272782439827 ) ) ;
#23682=CARTESIAN_POINT ( 'NONE',  ( -4.163336342344337027E-14, 1.387778780781445676E-14, 24.50000000000000000 ) ) ;
#23683=FACE_OUTER_BOUND ( 'NONE', #25098, .T. ) ;
#23688=DIRECTION ( 'NONE',  ( 1.000000000000000000, 0.000000000000000000, 0.000000000000000000 ) ) ;
#23690=LINE ( 'NONE', #27946, #18615 ) ;
#23694=EDGE_CURVE ( 'NONE', #25239, #28858, #16948, .T. ) ;
#23695=ORIENTED_EDGE ( 'NONE', *, *, #28242, .T. ) ;
#23696=ADVANCED_FACE ( 'NONE', ( #351 ), #24370, .F. ) ;
#23706=CIRCLE ( 'NONE', #10273, 20.00000000000000000 ) ;
#23707=CARTESIAN_POINT ( 'NONE',  ( 11.10715495309693601, -16.63223102436629830, 20.34789198813115263 ) ) ;
#23712=CARTESIAN_POINT ( 'NONE',  ( 10.65056555576078701, -13.34799940468896473, 19.02573955821369367 ) ) ;
#23713=B_SPLINE_CURVE_WITH_KNOTS ( 'NONE', 3,
 ( #8976, #30034, #1650, #8819, #13666, #21106, #9271, #18344, #11317, #23149, #1797, #27855, #22852, #23309, #30625, #6939 ),
 .UNSPECIFIED., .F., .F.,
 ( 4, 2, 2, 2, 2, 2, 2, 4 ),
 ( 0.4999999999999997780, 0.6249999999999998890, 0.6875000000000000000, 0.7187500000000000000, 0.7499999999999998890, 0.8124999999999997780, 0.8749999999999997780, 1.000000000000000000 ),
 .UNSPECIFIED. ) ;
#23717=DIRECTION ( 'NONE',  ( 1.000000000000000000, 0.000000000000000000, 0.000000000000000000 ) ) ;
#23719=CARTESIAN_POINT ( 'NONE',  ( 11.10715495309693424, -16.63223102436629475, 20.34789198813115263 ) ) ;
#23720=ORIENTED_EDGE ( 'NONE', *, *, #990, .T. ) ;
#23730=CARTESIAN_POINT ( 'NONE',  ( -4.163336342344337027E-14, 1.387778780781445676E-14, 1.500000000000000000 ) ) ;
#23733=VERTEX_POINT ( 'NONE', #7070 ) ;
#23738=DIRECTION ( 'NONE',  ( 1.000000000000000000, 0.000000000000000000, 0.000000000000000000 ) ) ;
#23746=AXIS2_PLACEMENT_3D ( 'NONE', #2268, #242, #6964 ) ;
#23749=CARTESIAN_POINT ( 'NONE',  ( 0.4421796641654207050, -17.03052986487778497, 20.29090034784956131 ) ) ;
#23751=CARTESIAN_POINT ( 'NONE',  ( -7.995704773938818732, -15.07639970738306801, 5.872146474157316831 ) ) ;
#23755=CARTESIAN_POINT ( 'NONE',  ( 18.53278507915170437, -7.520016387818809100, 7.528076282304597022 ) ) ;
#23757=CARTESIAN_POINT ( 'NONE',  ( 12.05308393316171234, 12.07205540120322595, 18.44527579819791185 ) ) ;
#23761=AXIS2_PLACEMENT_3D ( 'NONE', #10946, #27931, #1580 ) ;
#23764=CARTESIAN_POINT ( 'NONE',  ( -18.05883735157481951, -8.636530476581215865, 5.652196082364323360 ) ) ;
#23765=CARTESIAN_POINT ( 'NONE',  ( -13.20835299076127711, 10.76336294900085733, 20.32222155561919053 ) ) ;
#23766=CARTESIAN_POINT ( 'NONE',  ( -19.84404562991029763, 2.492760124447686465, 5.652196082369965069 ) ) ;
#23768=VECTOR ( 'NONE', #12509, 1000.000000000000114 ) ;
#23769=CARTESIAN_POINT ( 'NONE',  ( -15.16307466657772807, -7.786257835515859149, 18.34798005862930381 ) ) ;
#23772=ORIENTED_EDGE ( 'NONE', *, *, #18240, .F. ) ;
#23775=DIRECTION ( 'NONE',  ( -0.000000000000000000, -0.000000000000000000, -1.000000000000000000 ) ) ;
#23778=CARTESIAN_POINT ( 'NONE',  ( 0.000000000000000000, 0.000000000000000000, 1.500000000000001332 ) ) ;
#23779=VERTEX_POINT ( 'NONE', #26569 ) ;
#23782=CARTESIAN_POINT ( 'NONE',  ( 18.25868057198135830, -8.206406842115287148, 20.32842677360128292 ) ) ;
#23784=CARTESIAN_POINT ( 'NONE',  ( 6.247918173525850882, 19.01788707503811438, 6.864725433338323413 ) ) ;
#23787=CARTESIAN_POINT ( 'NONE',  ( 6.124711512895119725, 19.05797279266333888, 18.80699882434806369 ) ) ;
#23789=CARTESIAN_POINT ( 'NONE',  ( 11.77016209912416578, 12.36695356451125782, 7.196036389296800451 ) ) ;
#23793=EDGE_LOOP ( 'NONE', ( #13311, #11486, #11799, #28258 ) ) ;
#23797=AXIS2_PLACEMENT_3D ( 'NONE', #27109, #17914, #24755 ) ;
#23799=CARTESIAN_POINT ( 'NONE',  ( -18.47348503376728601, -7.710222065540590641, 6.755862304746362845 ) ) ;
#23801=DIRECTION ( 'NONE',  ( 1.000000000000000000, 0.000000000000000000, 0.000000000000000000 ) ) ;
#23802=CARTESIAN_POINT ( 'NONE',  ( -13.00999358272542494, -0.8602714556717691030, 1.500000000000001332 ) ) ;
#23803=CYLINDRICAL_SURFACE ( 'NONE', #14753, 0.7499999999999997780 ) ;
#23804=CARTESIAN_POINT ( 'NONE',  ( 10.50506478158603407, 13.32952022457704544, 24.50000000000000000 ) ) ;
#23808=VECTOR ( 'NONE', #23817, 1000.000000000000000 ) ;
#23809=CIRCLE ( 'NONE', #24328, 20.00000000000000000 ) ;
#23812=AXIS2_PLACEMENT_3D ( 'NONE', #2211, #9692, #25774 ) ;
#23815=CARTESIAN_POINT ( 'NONE',  ( -15.89566665641788745, 12.13797781250046270, 7.161525567826887873 ) ) ;
#23817=DIRECTION ( 'NONE',  ( 0.9898214418809327952, -0.1423148382732850048, 0.000000000000000000 ) ) ;
#23825=CARTESIAN_POINT ( 'NONE',  ( 18.59976559251667183, -7.400385892474094618, 18.56793045041961321 ) ) ;
#23826=CARTESIAN_POINT ( 'NONE',  ( 16.58777033243660526, 4.040313317649107283, 19.89182036555910571 ) ) ;
#23832=VECTOR ( 'NONE', #7668, 1000.000000000000000 ) ;
#23835=AXIS2_PLACEMENT_3D ( 'NONE', #30050, #15387, #17727 ) ;
#23839=CARTESIAN_POINT ( 'NONE',  ( -0.02788623088963465904, -17.02558298240835555, 19.96344307082652492 ) ) ;
#23841=CARTESIAN_POINT ( 'NONE',  ( 1.219801289189188287, -17.01504883035041260, 7.559636331181775581 ) ) ;
#23842=CARTESIAN_POINT ( 'NONE',  ( -14.70309389971831848, -8.688337726274234285, 19.47952243369110903 ) ) ;
#23845=ORIENTED_EDGE ( 'NONE', *, *, #27715, .T. ) ;
#23848=CARTESIAN_POINT ( 'NONE',  ( -4.163336342344337027E-14, 1.387778780781445676E-14, 1.500000000000000000 ) ) ;
#23850=ORIENTED_EDGE ( 'NONE', *, *, #26503, .T. ) ;
#23855=CARTESIAN_POINT ( 'NONE',  ( 1.000000000000008438, 13.00000000000001421, 24.50000000000000000 ) ) ;
#23857=CARTESIAN_POINT ( 'NONE',  ( 18.33793066653144876, -7.982499537706464920, 18.34798005863226678 ) ) ;
#23858=CARTESIAN_POINT ( 'NONE',  ( 0.000000000000000000, 0.000000000000000000, 21.50000000000000000 ) ) ;
#23864=ADVANCED_FACE ( 'NONE', ( #3783 ), #17663, .F. ) ;
#23866=AXIS2_PLACEMENT_3D ( 'NONE', #20425, #18411, #15907 ) ;
#23867=CARTESIAN_POINT ( 'NONE',  ( -17.98413878735053828, -8.751483025296222351, 18.34869673959212122 ) ) ;
#23868=CARTESIAN_POINT ( 'NONE',  ( 19.76377475971901632, 3.067715173639368853, 18.34726407865098707 ) ) ;
#23871=CARTESIAN_POINT ( 'NONE',  ( 14.89738168138696217, 13.37085340703111491, 7.652108011868850035 ) ) ;
#23873=EDGE_CURVE ( 'NONE', #4071, #13443, #20154, .T. ) ;
#23875=VECTOR ( 'NONE', #23102, 1000.000000000000000 ) ;
#23880=CARTESIAN_POINT ( 'NONE',  ( 10.29553672485768523, -13.60582241711869322, 20.24143955528809613 ) ) ;
#23886=CARTESIAN_POINT ( 'NONE',  ( 15.47543066133721901, -7.098048983968496373, 7.267659094423558841 ) ) ;
#23887=VECTOR ( 'NONE', #11151, 1000.000000000000000 ) ;
#23890=VERTEX_POINT ( 'NONE', #7844 ) ;
#23894=LINE ( 'NONE', #11737, #24172 ) ;
#23902=FACE_OUTER_BOUND ( 'NONE', #3484, .T. ) ;
#23904=CARTESIAN_POINT ( 'NONE',  ( 1.000000000000008438, 16.48749217771910125, 1.500000000000000000 ) ) ;
#23907=LINE ( 'NONE', #14696, #13461 ) ;
#23908=ORIENTED_EDGE ( 'NONE', *, *, #4791, .T. ) ;
#23909=VERTEX_POINT ( 'NONE', #2041 ) ;
#23910=DIRECTION ( 'NONE',  ( 1.000000000000000000, 0.000000000000000000, 0.000000000000000000 ) ) ;
#23911=VERTEX_POINT ( 'NONE', #18450 ) ;
#23912=AXIS2_PLACEMENT_3D ( 'NONE', #22802, #22638, #27184 ) ;
#23914=ORIENTED_EDGE ( 'NONE', *, *, #15246, .F. ) ;
#23915=FACE_OUTER_BOUND ( 'NONE', #22363, .T. ) ;
#23916=LINE ( 'NONE', #2562, #21457 ) ;
#23917=CARTESIAN_POINT ( 'NONE',  ( 4.303751186633993697, 16.48600304573620789, 20.32222155561919053 ) ) ;
#23918=CARTESIAN_POINT ( 'NONE',  ( 0.5710336623368660325, -20.00960304012541258, 20.32367522806703874 ) ) ;
#23919=ORIENTED_EDGE ( 'NONE', *, *, #25723, .T. ) ;
#23920=CARTESIAN_POINT ( 'NONE',  ( 18.44003002641400712, -7.744679585886125928, 7.626218077512941562 ) ) ;
#23922=CARTESIAN_POINT ( 'NONE',  ( 11.86828576611215347, 12.26598719735377152, 20.06253562465620632 ) ) ;
#23925=ADVANCED_FACE ( 'NONE', ( #22951 ), #15948, .F. ) ;
#23928=DIRECTION ( 'NONE',  ( -0.000000000000000000, -0.000000000000000000, 1.000000000000000000 ) ) ;
#23929=CARTESIAN_POINT ( 'NONE',  ( -6.914714884271990769, 18.78545221144173638, 6.892848776733236704 ) ) ;
#23934=CARTESIAN_POINT ( 'NONE',  ( 3.912171961291952993, 8.637616862297855747, 13.00000000000000178 ) ) ;
#23940=CARTESIAN_POINT ( 'NONE',  ( 11.77028954461707144, -16.17000817291664205, 19.96797677718664588 ) ) ;
#23941=EDGE_LOOP ( 'NONE', ( #11234, #6116, #22211, #4061 ) ) ;
#23943=CARTESIAN_POINT ( 'NONE',  ( 4.744089322959556654, 16.35312844164165114, 7.359006845440219102 ) ) ;
#23945=CARTESIAN_POINT ( 'NONE',  ( 4.996079307276525938, 16.27198743970616235, 19.11611934778430921 ) ) ;
#23946=CARTESIAN_POINT ( 'NONE',  ( 14.67322144252663740, 13.61684651386558187, 7.603368798681074736 ) ) ;
#23957=CARTESIAN_POINT ( 'NONE',  ( 14.20168120032941950, 14.08243226175161844, 6.392525840300335105 ) ) ;
#23958=CARTESIAN_POINT ( 'NONE',  ( 0.01636335959932776890, -20.01808238691632624, 5.701226463332907279 ) ) ;
#23970=( NAMED_UNIT ( * ) PLANE_ANGLE_UNIT ( ) SI_UNIT ( $, .RADIAN. ) );
#23971=ORIENTED_EDGE ( 'NONE', *, *, #11146, .T. ) ;
#23975=CARTESIAN_POINT ( 'NONE',  ( 16.19545619402287073, -5.420160174983553958, 19.25672174529527325 ) ) ;
#23976=CARTESIAN_POINT ( 'NONE',  ( 19.70397673731432064, 3.532048315275336581, 18.39992786714538298 ) ) ;
#23979=CARTESIAN_POINT ( 'NONE',  ( 15.44249669567090777, -7.165351778216223266, 19.85270094495842130 ) ) ;
#23981=VECTOR ( 'NONE', #13881, 1000.000000000000000 ) ;
#23984=CARTESIAN_POINT ( 'NONE',  ( -17.92868989761418774, -8.864358285757575118, 7.626218077512941562 ) ) ;
#23985=VECTOR ( 'NONE', #10389, 1000.000000000000000 ) ;
#23986=CARTESIAN_POINT ( 'NONE',  ( -8.163758309741956154, -14.97879848885351173, 18.44527579819791185 ) ) ;
#23987=CARTESIAN_POINT ( 'NONE',  ( -14.72786953156221301, -8.642539778700260911, 19.02573955821368656 ) ) ;
#23988=DIRECTION ( 'NONE',  ( 1.000000000000000000, 0.000000000000000000, 0.000000000000000000 ) ) ;
#23990=VERTEX_POINT ( 'NONE', #8620 ) ;
#23991=EDGE_CURVE ( 'NONE', #16019, #12864, #25614, .T. ) ;
#23992=CARTESIAN_POINT ( 'NONE',  ( 9.766261594859265927, -13.96654203752514967, 7.652108011868850035 ) ) ;
#23993=CARTESIAN_POINT ( 'NONE',  ( 15.81416325002591527, -6.360572704314728654, 5.652196082367003882 ) ) ;
#23995=CARTESIAN_POINT ( 'NONE',  ( -5.971396161871752817, 19.08775596758252036, 20.34789198813115263 ) ) ;
#24001=CARTESIAN_POINT ( 'NONE',  ( -4.786560543001536772, 16.33923032321832025, 18.71435384576123440 ) ) ;
#24002=CARTESIAN_POINT ( 'NONE',  ( -10.47960520055065636, -7.757439966934454034, 1.500000000000001332 ) ) ;
#24006=CARTESIAN_POINT ( 'NONE',  ( -2.959227181723746547, 8.499586724479465616, 21.50000000000000000 ) ) ;
#24007=DIRECTION ( 'NONE',  ( -1.000000000000000000, 0.000000000000000000, 0.000000000000000000 ) ) ;
#24009=EDGE_LOOP ( 'NONE', ( #17779, #14076, #18943, #7215 ) ) ;
#24010=CARTESIAN_POINT ( 'NONE',  ( 15.36220013476732404, 12.83425670785759110, 5.940635272151477686 ) ) ;
#24011=CARTESIAN_POINT ( 'NONE',  ( -15.26435939152463384, 8.070345032481604619, 24.50000000000000000 ) ) ;
#24019=CARTESIAN_POINT ( 'NONE',  ( 5.080682615984644990, 19.36225455879193902, 5.678370764302467677 ) ) ;
#24020=EDGE_CURVE ( 'NONE', #7300, #11919, #13750, .T. ) ;
#24023=LINE ( 'NONE', #2990, #23768 ) ;
#24024=CARTESIAN_POINT ( 'NONE',  ( -18.37606348208443663, -7.894877446839462465, 6.033082186765047261 ) ) ;
#24025=CARTESIAN_POINT ( 'NONE',  ( 0.000000000000000000, 0.000000000000000000, 1.500000000000001332 ) ) ;
#24029=VERTEX_POINT ( 'NONE', #23244 ) ;
#24030=EDGE_CURVE ( 'NONE', #13582, #16299, #21912, .T. ) ;
#24031=CARTESIAN_POINT ( 'NONE',  ( 15.75996277362376752, -6.485024779661078043, 7.652108011868851811 ) ) ;
#24036=CARTESIAN_POINT ( 'NONE',  ( -14.77756128048222983, -8.549967187541072988, 19.89182036555910571 ) ) ;
#24041=EDGE_CURVE ( 'NONE', #17088, #27593, #3918, .T. ) ;
#24042=ORIENTED_EDGE ( 'NONE', *, *, #29953, .F. ) ;
#24043=DIRECTION ( 'NONE',  ( 1.000000000000000000, 0.000000000000000000, 0.000000000000000000 ) ) ;
#24044=EDGE_CURVE ( 'NONE', #30524, #27003, #7496, .T. ) ;
#24055=CARTESIAN_POINT ( 'NONE',  ( -10.51100883930069863, -17.01524884273342053, 5.652196082369965069 ) ) ;
#24058=CARTESIAN_POINT ( 'NONE',  ( -0.1272161363927089561, -17.02285684280287725, 18.90679857307105749 ) ) ;
#24063=CARTESIAN_POINT ( 'NONE',  ( -7.857295329535767259, -15.15488436941561901, 6.041646659195333058 ) ) ;
#24064=CARTESIAN_POINT ( 'NONE',  ( 4.537114061097054396, 16.41705816686735986, 20.22273502201483453 ) ) ;
#24065=CARTESIAN_POINT ( 'NONE',  ( 1.327349630778745793, -17.01025715289075535, 18.50655187082627862 ) ) ;
#24067=EDGE_CURVE ( 'NONE', #8165, #23071, #25899, .T. ) ;
#24068=CARTESIAN_POINT ( 'NONE',  ( 18.39103589699441699, -7.860502636612781480, 5.652912763329822177 ) ) ;
#24072=CARTESIAN_POINT ( 'NONE',  ( 11.80864398233534907, 12.32734916534601943, 18.73743063545763121 ) ) ;
#24073=DIRECTION ( 'NONE',  ( 1.000000000000000000, -0.000000000000000000, 0.000000000000000000 ) ) ;
#24076=EDGE_CURVE ( 'NONE', #24787, #2507, #18461, .T. ) ;
#24079=CARTESIAN_POINT ( 'NONE',  ( -6.374050743166105981, 15.83881588044504163, 6.131018562779544823 ) ) ;
#24080=CARTESIAN_POINT ( 'NONE',  ( -19.91205802435384697, 1.875831072725643089, 5.853797745100181693 ) ) ;
#24084=CARTESIAN_POINT ( 'NONE',  ( -18.09182123201597747, -8.567353834808583812, 18.34969686940295830 ) ) ;
#24086=ORIENTED_EDGE ( 'NONE', *, *, #11278, .T. ) ;
#24087=ORIENTED_EDGE ( 'NONE', *, *, #23044, .F. ) ;
#24089=CARTESIAN_POINT ( 'NONE',  ( -5.719992972340611104, 19.16498258860013237, 20.32243167357988867 ) ) ;
#24090=CARTESIAN_POINT ( 'NONE',  ( -12.96319695304515029, 11.04295072071645478, 7.429667576816606278 ) ) ;
#24092=ORIENTED_EDGE ( 'NONE', *, *, #4703, .T. ) ;
#24094=CARTESIAN_POINT ( 'NONE',  ( 9.406652940105985294, -1.195154792889428608, 1.500000000000001332 ) ) ;
#24095=CIRCLE ( 'NONE', #4685, 0.7500000000000011102 ) ;
#24098=CARTESIAN_POINT ( 'NONE',  ( 4.930301257365631962, 16.29355789806660582, 19.77662771831109367 ) ) ;
#24100=CARTESIAN_POINT ( 'NONE',  ( 12.20938699334973165, 11.90340052968386075, 7.627891251804737927 ) ) ;
#24112=CARTESIAN_POINT ( 'NONE',  ( -0.6060441907983112886, -20.00878639882294863, 6.310736198168394928 ) ) ;
#24113=LINE ( 'NONE', #561, #21217 ) ;
#24119=DIRECTION ( 'NONE',  ( 0.000000000000000000, 0.000000000000000000, 1.000000000000000000 ) ) ;
#24121=ORIENTED_EDGE ( 'NONE', *, *, #7324, .T. ) ;
#24127=CARTESIAN_POINT ( 'NONE',  ( -9.310272263096074141, -14.25176022191445391, 6.211014596808754007 ) ) ;
#24129=CARTESIAN_POINT ( 'NONE',  ( 15.84452017418781367, -6.290821626254204268, 18.34838970509067479 ) ) ;
#24130=CARTESIAN_POINT ( 'NONE',  ( 19.58381725123994244, 4.144794415032112767, 19.03762469184452755 ) ) ;
#24133=ORIENTED_EDGE ( 'NONE', *, *, #21808, .T. ) ;
#24137=ORIENTED_EDGE ( 'NONE', *, *, #24255, .T. ) ;
#24139=CIRCLE ( 'NONE', #1259, 20.00000000000000000 ) ;
#24141=CARTESIAN_POINT ( 'NONE',  ( -6.240920525956804354, 15.88642679632095600, 18.64703902303423178 ) ) ;
#24143=CARTESIAN_POINT ( 'NONE',  ( -9.723733991145053324, -17.49730778217156413, 18.92976555901915603 ) ) ;
#24145=DIRECTION ( 'NONE',  ( -0.000000000000000000, -0.000000000000000000, 1.000000000000000000 ) ) ;
#24147=ORIENTED_EDGE ( 'NONE', *, *, #23562, .T. ) ;
#24148=CARTESIAN_POINT ( 'NONE',  ( 10.66524827722686197, -16.94040236790928944, 5.796888747622817029 ) ) ;
#24150=CARTESIAN_POINT ( 'NONE',  ( -15.56646378676711784, 12.58598989586693939, 7.603368798681074736 ) ) ;
#24155=FACE_OUTER_BOUND ( 'NONE', #23793, .T. ) ;
#24156=CARTESIAN_POINT ( 'NONE',  ( -5.364573742045088522, 19.28565133533678733, 7.429667576816606278 ) ) ;
#24157=CARTESIAN_POINT ( 'NONE',  ( 8.840471615930072247, -1.687027447297460236, 1.500000000000001332 ) ) ;
#24158=CARTESIAN_POINT ( 'NONE',  ( -5.196396160405787334, 19.31337320890706977, 7.267242832833944455 ) ) ;
#24159=VERTEX_POINT ( 'NONE', #7653 ) ;
#24160=VERTEX_POINT ( 'NONE', #26676 ) ;
#24164=VERTEX_POINT ( 'NONE', #5305 ) ;
#24165=FACE_OUTER_BOUND ( 'NONE', #3275, .T. ) ;
#24172=VECTOR ( 'NONE', #28896, 1000.000000000000000 ) ;
#24173=CARTESIAN_POINT ( 'NONE',  ( 3.718735505629741311, 16.64535199026476420, 5.704143890883081269 ) ) ;
#24175=ORIENTED_EDGE ( 'NONE', *, *, #23095, .T. ) ;
#24178=CARTESIAN_POINT ( 'NONE',  ( -13.11527592942575282, -10.04126165406389326, -0.6213203435596476032 ) ) ;
#24179=CARTESIAN_POINT ( 'NONE',  ( 9.489008252200360261, -14.14611184196830784, 20.25336174263950184 ) ) ;
#24186=VERTEX_POINT ( 'NONE', #16539 ) ;
#24187=CARTESIAN_POINT ( 'NONE',  ( -17.62838677698389489, -9.483948870226237560, 19.69140814234746273 ) ) ;
#24199=CARTESIAN_POINT ( 'NONE',  ( 9.249586724479433641, 2.959227181723830036, 1.500000000000001332 ) ) ;
#24203=ORIENTED_EDGE ( 'NONE', *, *, #12625, .T. ) ;
#24211=CARTESIAN_POINT ( 'NONE',  ( -0.3606176111512355287, -20.01462698034515242, 18.63641924841378028 ) ) ;
#24215=CARTESIAN_POINT ( 'NONE',  ( 5.015798959889849584, 16.26549279019886995, 19.21496526180054332 ) ) ;
#24218=VERTEX_POINT ( 'NONE', #19806 ) ;
#24219=AXIS2_PLACEMENT_3D ( 'NONE', #7920, #26317, #267 ) ;
#24220=ADVANCED_FACE ( 'NONE', ( #768 ), #29830, .T. ) ;
#24223=CARTESIAN_POINT ( 'NONE',  ( 11.75961732103505497, 12.37772240090665932, 18.82680253904184298 ) ) ;
#24229=DIRECTION ( 'NONE',  ( 0.000000000000000000, 0.000000000000000000, -1.000000000000000000 ) ) ;
#24230=CARTESIAN_POINT ( 'NONE',  ( -6.509484584620659930, 15.78915919539661949, 6.560937769032974209 ) ) ;
#24231=CARTESIAN_POINT ( 'NONE',  ( -19.87571927687823248, 2.229464111918809888, 5.679672709359370408 ) ) ;
#24233=CARTESIAN_POINT ( 'NONE',  ( -18.46504858183724096, -7.730374101464834169, 19.11611934778430921 ) ) ;
#24235=VECTOR ( 'NONE', #28427, 1000.000000000000000 ) ;
#24237=VERTEX_POINT ( 'NONE', #4192 ) ;
#24241=CARTESIAN_POINT ( 'NONE',  ( -14.68399241520484466, 13.60504237629023017, 6.641371103590088865 ) ) ;
#24244=ORIENTED_EDGE ( 'NONE', *, *, #2531, .F. ) ;
#24248=CIRCLE ( 'NONE', #25259, 0.7500000000000002220 ) ;
#24250=CARTESIAN_POINT ( 'NONE',  ( -10.51513057463695411, -17.01270198993486460, 7.652108011868850035 ) ) ;
#24251=AXIS2_PLACEMENT_3D ( 'NONE', #20050, #873, #10395 ) ;
#24254=VECTOR ( 'NONE', #10157, 1000.000000000000000 ) ;
#24255=EDGE_CURVE ( 'NONE', #17054, #12148, #11384, .T. ) ;
#24268=ORIENTED_EDGE ( 'NONE', *, *, #5186, .T. ) ;
#24269=CARTESIAN_POINT ( 'NONE',  ( -15.39003174319561218, -7.295547530644704182, 5.796888747622817029 ) ) ;
#24271=CARTESIAN_POINT ( 'NONE',  ( -0.6388627779519707728, -20.00771244368418067, 6.420335371522007506 ) ) ;
#24272=CIRCLE ( 'NONE', #11833, 9.482273699623480212 ) ;
#24284=VERTEX_POINT ( 'NONE', #20716 ) ;
#24289=VECTOR ( 'NONE', #18913, 1000.000000000000000 ) ;
#24291=CIRCLE ( 'NONE', #8879, 0.7500000000000006661 ) ;
#24292=CARTESIAN_POINT ( 'NONE',  ( 12.64536614603775888, 11.41255465792765378, 18.44501272782439827 ) ) ;
#24293=CARTESIAN_POINT ( 'NONE',  ( -8.643687819870516265, -14.68753251638875845, 5.657991946698900598 ) ) ;
#24294=ORIENTED_EDGE ( 'NONE', *, *, #18157, .F. ) ;
#24295=CARTESIAN_POINT ( 'NONE',  ( 16.14429390779610785, -5.555032456232098959, 18.82680253904184298 ) ) ;
#24296=CARTESIAN_POINT ( 'NONE',  ( 16.68596330270455752, 3.532048315275336581, 18.39992786714538298 ) ) ;
#24299=VERTEX_POINT ( 'NONE', #1562 ) ;
#24300=VECTOR ( 'NONE', #28458, 1000.000000000000000 ) ;
#24301=CARTESIAN_POINT ( 'NONE',  ( 15.81416692036122207, -6.360574302898111654, 18.34798005863078885 ) ) ;
#24304=AXIS2_PLACEMENT_3D ( 'NONE', #1852, #30396, #19002 ) ;
#24305=CARTESIAN_POINT ( 'NONE',  ( -7.706848733600993206, -5.524309650260738280, 21.50000000000000000 ) ) ;
#24306=CARTESIAN_POINT ( 'NONE',  ( -6.507320782993286201, 15.78995902672676621, 19.36813350477385143 ) ) ;
#24307=CARTESIAN_POINT ( 'NONE',  ( -14.69323076807464545, 13.59505578765952727, 19.22654678686458141 ) ) ;
#24311=CARTESIAN_POINT ( 'NONE',  ( 7.724883619896791842, 5.687793815610376669, 1.500000000000001332 ) ) ;
#24312=CARTESIAN_POINT ( 'NONE',  ( 8.499586724479435418, 2.959227181723830036, 1.500000000000001332 ) ) ;
#24314=CARTESIAN_POINT ( 'NONE',  ( -16.97503503882430209, 1.572081968053592904, 5.652605728828373977 ) ) ;
#24316=VECTOR ( 'NONE', #5402, 1000.000000000000000 ) ;
#24317=CARTESIAN_POINT ( 'NONE',  ( 19.83258132550259845, 2.584089194578472970, 5.849008070840543638 ) ) ;
#24319=VERTEX_POINT ( 'NONE', #11071 ) ;
#24321=CARTESIAN_POINT ( 'NONE',  ( 10.42970548045642509, -17.06546344489797207, 6.033082186765059696 ) ) ;
#24323=DIRECTION ( 'NONE',  ( -1.000000000000000000, 0.000000000000000000, 0.000000000000000000 ) ) ;
#24326=EDGE_CURVE ( 'NONE', #27034, #14242, #28048, .T. ) ;
#24328=AXIS2_PLACEMENT_3D ( 'NONE', #7910, #1190, #25041 ) ;
#24329=DIRECTION ( 'NONE',  ( -0.000000000000000000, -0.000000000000000000, 1.000000000000000000 ) ) ;
#24332=DIRECTION ( 'NONE',  ( 0.000000000000000000, 0.000000000000000000, 1.000000000000000000 ) ) ;
#24333=VERTEX_POINT ( 'NONE', #25107 ) ;
#24336=CARTESIAN_POINT ( 'NONE',  ( 16.08779849516156446, -5.700297231796353614, 7.366751648393900176 ) ) ;
#24337=DIRECTION ( 'NONE',  ( 0.000000000000000000, 0.000000000000000000, 1.000000000000000000 ) ) ;
#24338=AXIS2_PLACEMENT_3D ( 'NONE', #30642, #28331, #16007 ) ;
#24340=ORIENTED_EDGE ( 'NONE', *, *, #29680, .T. ) ;
#24341=CARTESIAN_POINT ( 'NONE',  ( 5.298969250677092013, 19.30368332842023094, 5.652196082364323360 ) ) ;
#24343=CARTESIAN_POINT ( 'NONE',  ( -4.163336342344337027E-14, 1.387778780781445676E-14, 24.50000000000000000 ) ) ;
#24345=LINE ( 'NONE', #27318, #23832 ) ;
#24352=CARTESIAN_POINT ( 'NONE',  ( -15.57270467870639052, 12.57827228024024713, 18.39992786714538298 ) ) ;
#24353=FACE_OUTER_BOUND ( 'NONE', #8264, .T. ) ;
#24357=B_SPLINE_CURVE_WITH_KNOTS ( 'NONE', 3,
 ( #5301, #17624, #12492, #5623, #14812, #7797, #27296, #934, #3584, #21984, #1092, #5465, #20116, #29634, #17474, #14967, #12795, #10132 ),
 .UNSPECIFIED., .F., .F.,
 ( 4, 2, 2, 2, 2, 2, 2, 2, 4 ),
 ( 0.003174295595554332133, 0.003570702171545570968, 0.003967108747536809803, 0.004363515323528049071, 0.004759921899519287472, 0.005156328475510526740, 0.005552735051501766009, 0.005949141627493005277, 0.006345548203484243678 ),
 .UNSPECIFIED. ) ;
#24359=CARTESIAN_POINT ( 'NONE',  ( 4.176140024716620047, 16.52246432929376496, 7.652108011868850035 ) ) ;
#24361=CIRCLE ( 'NONE', #10432, 0.7500000000000006661 ) ;
#24363=CARTESIAN_POINT ( 'NONE',  ( 16.87858066272421809, 2.200498455867148984, 6.782064869129510676 ) ) ;
#24366=CIRCLE ( 'NONE', #4452, 0.7500000000000002220 ) ;
#24370=CYLINDRICAL_SURFACE ( 'NONE', #4, 9.482273699623480212 ) ;
#24373=CARTESIAN_POINT ( 'NONE',  ( 1.964582201835851638, -2.267248723062833538, 24.50000000000000000 ) ) ;
#24375=AXIS2_PLACEMENT_3D ( 'NONE', #26597, #5223, #17686 ) ;
#24386=CARTESIAN_POINT ( 'NONE',  ( 1.424502173535766802, -17.00587888132690395, 5.872146474157316831 ) ) ;
#24390=DIRECTION ( 'NONE',  ( 1.000000000000000000, 0.000000000000000000, 0.000000000000000000 ) ) ;
#24391=DIRECTION ( 'NONE',  ( 0.000000000000000000, 0.000000000000000000, 1.000000000000000000 ) ) ;
#24396=CARTESIAN_POINT ( 'NONE',  ( -9.131494062835631809, -2.555255504830933333, 13.00000000000000178 ) ) ;
#24398=DIRECTION ( 'NONE',  ( 0.000000000000000000, 0.000000000000000000, 1.000000000000000000 ) ) ;
#24399=DIRECTION ( 'NONE',  ( 1.000000000000000000, 0.000000000000000000, 0.000000000000000000 ) ) ;
#24400=CARTESIAN_POINT ( 'NONE',  ( -15.20706373417739776, 13.01805446572691594, 7.632642797338977658 ) ) ;
#24405=CARTESIAN_POINT ( 'NONE',  ( 15.63429980755321225, -6.761683097800862186, 18.44501272782439827 ) ) ;
#24408=ORIENTED_EDGE ( 'NONE', *, *, #2304, .T. ) ;
#24409=CARTESIAN_POINT ( 'NONE',  ( 4.155601639749238352, 16.52779251924067339, 18.35377592296120497 ) ) ;
#24410=CARTESIAN_POINT ( 'NONE',  ( -8.430595340551228389, 4.340342926365043930, 21.50000000000000000 ) ) ;
#24413=ORIENTED_EDGE ( 'NONE', *, *, #27082, .F. ) ;
#24416=CARTESIAN_POINT ( 'NONE',  ( -19.77413607932157902, 2.999736578675611387, 20.22277707861862339 ) ) ;
#24418=CARTESIAN_POINT ( 'NONE',  ( -15.16307466657772451, -7.786257835515858261, 5.652196082367002106 ) ) ;
#24420=EDGE_CURVE ( 'NONE', #321, #21094, #13497, .T. ) ;
#24421=CARTESIAN_POINT ( 'NONE',  ( 14.45728346696244238, 13.82012126338014468, 5.853797745100180805 ) ) ;
#24423=DIRECTION ( 'NONE',  ( 1.000000000000000000, 0.000000000000000000, 0.000000000000000000 ) ) ;
#24424=VECTOR ( 'NONE', #24753, 1000.000000000000000 ) ;
#24431=VERTEX_POINT ( 'NONE', #19158 ) ;
#24432=ADVANCED_FACE ( 'NONE', ( #7308 ), #18858, .F. ) ;
#24433=CARTESIAN_POINT ( 'NONE',  ( -5.544451647051929832, 16.11829164193972019, 7.652108011868850923 ) ) ;
#24434=DIRECTION ( 'NONE',  ( -0.000000000000000000, -0.000000000000000000, 1.000000000000000000 ) ) ;
#24443=CARTESIAN_POINT ( 'NONE',  ( 15.51850634784530136, 12.64495090725178983, 19.00652017443069752 ) ) ;
#24444=EDGE_CURVE ( 'NONE', #19956, #2072, #10009, .T. ) ;
#24445=CARTESIAN_POINT ( 'NONE',  ( -11.12409513110480397, -16.64241105543193555, 5.940635272151477686 ) ) ;
#24447=CARTESIAN_POINT ( 'NONE',  ( -19.81587719261256098, 2.836291464538556628, 7.595116371587256054 ) ) ;
#24448=AXIS2_PLACEMENT_3D ( 'NONE', #8493, #15635, #1465 ) ;
#24449=CARTESIAN_POINT ( 'NONE',  ( 18.28362707703099588, -8.107168301167737567, 7.652108011868849147 ) ) ;
#24450=CARTESIAN_POINT ( 'NONE',  ( 8.499586724479435418, 2.959227181723830036, 21.50000000000000000 ) ) ;
#24455=ORIENTED_EDGE ( 'NONE', *, *, #15251, .T. ) ;
#24457=EDGE_CURVE ( 'NONE', #2397, #4512, #3535, .T. ) ;
#24459=CARTESIAN_POINT ( 'NONE',  ( -5.764374838704560133, 16.04809504443725743, 18.37415474056476938 ) ) ;
#24460=CARTESIAN_POINT ( 'NONE',  ( -13.37849590052435289, 10.56201291103764284, 20.34789198813115263 ) ) ;
#24461=EDGE_CURVE ( 'NONE', #19951, #16299, #515, .T. ) ;
#24467=CARTESIAN_POINT ( 'NONE',  ( 10.39222174957287770, -17.10906616942579817, 6.111214848085761986 ) ) ;
#24470=DIRECTION ( 'NONE',  ( 1.000000000000000000, 0.000000000000000000, 0.000000000000000000 ) ) ;
#24473=CARTESIAN_POINT ( 'NONE',  ( 18.12921809165262843, -8.446683920555059899, 18.47110296274025387 ) ) ;
#24474=CARTESIAN_POINT ( 'NONE',  ( 10.68464666747177105, -16.90719797777716948, 5.775318986477953942 ) ) ;
#24477=CARTESIAN_POINT ( 'NONE',  ( 11.65964093050818917, 12.47882650181265163, 6.588756557121052460 ) ) ;
#24478=DIRECTION ( 'NONE',  ( 0.000000000000000000, 0.000000000000000000, 1.000000000000000000 ) ) ;
#24482=CARTESIAN_POINT ( 'NONE',  ( -9.815074746724004484, -17.42621888692031717, 18.73377938172347967 ) ) ;
#24484=CARTESIAN_POINT ( 'NONE',  ( 19.76665705046225696, 3.161078882829541747, 5.651989602109218858 ) ) ;
#24485=VERTEX_POINT ( 'NONE', #5120 ) ;
#24486=CARTESIAN_POINT ( 'NONE',  ( 15.54774248266353176, 12.60889669900781129, 6.530762810602277924 ) ) ;
#24488=CARTESIAN_POINT ( 'NONE',  ( 16.05603743463489863, -5.780788835868666986, 7.441806358946449151 ) ) ;
#24489=EDGE_CURVE ( 'NONE', #20736, #17664, #27107, .T. ) ;
#24499=CARTESIAN_POINT ( 'NONE',  ( 9.186411229153639724, -14.33460949872161549, 19.96783386855779341 ) ) ;
#24503=FACE_OUTER_BOUND ( 'NONE', #21235, .T. ) ;
#24504=DIRECTION ( 'NONE',  ( 0.000000000000000000, 0.000000000000000000, 1.000000000000000000 ) ) ;
#24508=CARTESIAN_POINT ( 'NONE',  ( -15.01515151829605976, 13.21212483861245346, 18.47110296274025742 ) ) ;
#24513=FACE_OUTER_BOUND ( 'NONE', #30808, .T. ) ;
#24518=CYLINDRICAL_SURFACE ( 'NONE', #736, 0.7500000000000011102 ) ;
#24523=CARTESIAN_POINT ( 'NONE',  ( -10.07574916981069357, -17.27697906656895910, 5.779535427900759359 ) ) ;
#24525=ORIENTED_EDGE ( 'NONE', *, *, #29838, .T. ) ;
#24532=DIRECTION ( 'NONE',  ( -0.000000000000000000, -0.000000000000000000, 1.000000000000000000 ) ) ;
#24536=CARTESIAN_POINT ( 'NONE',  ( 1.964582201835905151, 2.267248723062786908, 24.50000000000000000 ) ) ;
#24539=CARTESIAN_POINT ( 'NONE',  ( -9.378051617232568304, -14.20529941771991211, 19.11611934778430921 ) ) ;
#24541=CARTESIAN_POINT ( 'NONE',  ( -6.426383236738485216, 15.81971323177988253, 6.233981582756856987 ) ) ;
#24543=CARTESIAN_POINT ( 'NONE',  ( 10.68026781623521693, -13.32599531033824825, 6.447548852708279377 ) ) ;
#24547=ORIENTED_EDGE ( 'NONE', *, *, #25581, .F. ) ;
#24549=CARTESIAN_POINT ( 'NONE',  ( -5.976020107417636673, 19.08630880174946043, 18.34798005863226678 ) ) ;
#24551=CARTESIAN_POINT ( 'NONE',  ( 6.631244434206235105, 6.812559277181991391, 21.50000000000000000 ) ) ;
#24552=ORIENTED_EDGE ( 'NONE', *, *, #27507, .F. ) ;
#24554=CARTESIAN_POINT ( 'NONE',  ( 18.33777834721833599, -8.027392848387998825, 18.34777357837152323 ) ) ;
#24558=CARTESIAN_POINT ( 'NONE',  ( -7.706848733600993206, -5.524309650260738280, 13.00000000000000178 ) ) ;
#24559=B_SPLINE_SURFACE_WITH_KNOTS ( 'NONE', 3, 1, ( 
 ( #16739, #17049 ),
 ( #25954, #18945 ),
 ( #9880, #4732 ),
 ( #14562, #23749 ),
 ( #2560, #14234 ),
 ( #205, #26253 ),
 ( #28603, #28758 ),
 ( #21098, #11929 ),
 ( #2401, #61 ),
 ( #28455, #26577 ),
 ( #19398, #7079 ),
 ( #7395, #16906 ),
 ( #12218, #359 ),
 ( #7226, #21719 ),
 ( #4582, #26422 ),
 ( #23593, #28916 ),
 ( #28304, #5202 ),
 ( #19230, #12073 ),
 ( #14705, #24058 ),
 ( #2237, #16586 ),
 ( #21419, #30618 ),
 ( #24211, #2863 ),
 ( #6929, #9574 ),
 ( #4893, #16441 ),
 ( #9265, #21569 ),
 ( #11756, #18784 ),
 ( #14084, #21252 ),
 ( #14412, #30780 ),
 ( #9429, #19856 ),
 ( #13001, #670 ),
 ( #17838, #29530 ) ),
 .UNSPECIFIED., .F., .F., .F.,
 ( 4, 3, 3, 3, 3, 3, 3, 3, 3, 3, 4 ),
 ( 2, 2 ),
 ( 0.000000000000000000, 0.05425176834609614362, 0.1085332949128348518, 0.1623767749169379715, 0.2157504826133058717, 0.2688657508888169789, 0.3218907763505471364, 0.3749548578363334772, 0.4282048033836237666, 0.4818374082110496448, 0.4999999999131651274 ),
 ( 0.000000000000000000, 1.000000000000000000 ),
 .UNSPECIFIED. ) ;
#24561=CARTESIAN_POINT ( 'NONE',  ( 0.000000000000000000, 0.000000000000000000, 21.50000000000000000 ) ) ;
#24567=AXIS2_PLACEMENT_3D ( 'NONE', #24157, #7340, #2806 ) ;
#24569=DIRECTION ( 'NONE',  ( 0.000000000000000000, 0.000000000000000000, -1.000000000000000000 ) ) ;
#24570=ORIENTED_EDGE ( 'NONE', *, *, #16290, .F. ) ;
#24575=LINE ( 'NONE', #14755, #13838 ) ;
#24580=AXIS2_PLACEMENT_3D ( 'NONE', #21031, #4665, #13726 ) ;
#24581=CARTESIAN_POINT ( 'NONE',  ( 4.690519134554615555, 19.44242338873975484, 5.853797745100186134 ) ) ;
#24582=ORIENTED_EDGE ( 'NONE', *, *, #3065, .T. ) ;
#24583=ORIENTED_EDGE ( 'NONE', *, *, #24644, .T. ) ;
#24584=AXIS2_PLACEMENT_3D ( 'NONE', #19067, #10284, #14810 ) ;
#24585=CARTESIAN_POINT ( 'NONE',  ( -4.668110441710642711, -19.44758969394387194, 24.50000000000000000 ) ) ;
#24591=CARTESIAN_POINT ( 'NONE',  ( 14.94527285076313916, 13.31737086058187458, 18.34969686940296185 ) ) ;
#24594=EDGE_CURVE ( 'NONE', #24164, #7313, #1064, .T. ) ;
#24595=CARTESIAN_POINT ( 'NONE',  ( -19.74495986540963344, 3.294819794740638574, 7.272049892295485485 ) ) ;
#24596=CARTESIAN_POINT ( 'NONE',  ( 19.74942470869275724, 3.267558643021993614, 20.34789198813115263 ) ) ;
#24599=EDGE_LOOP ( 'NONE', ( #10300, #30044 ) ) ;
#24600=LINE ( 'NONE', #29603, #12874 ) ;
#24601=EDGE_CURVE ( 'NONE', #13769, #4888, #20939, .T. ) ;
#24602=ORIENTED_EDGE ( 'NONE', *, *, #14950, .T. ) ;
#24604=CARTESIAN_POINT ( 'NONE',  ( -16.96556290498877573, 1.647560670993253540, 18.34798005863078885 ) ) ;
#24605=ORIENTED_EDGE ( 'NONE', *, *, #16017, .T. ) ;
#24607=CARTESIAN_POINT ( 'NONE',  ( -6.228680293130164358, 19.00574304797303782, 18.37545668562167478 ) ) ;
#24611=CARTESIAN_POINT ( 'NONE',  ( -18.04365185506137337, -8.627086862512673093, 7.652108011868850035 ) ) ;
#24613=CARTESIAN_POINT ( 'NONE',  ( -10.23401665697057084, -17.20427178438287541, 18.39992786714538298 ) ) ;
#24617=PLANE ( 'NONE',  #12867 ) ;
#24619=CARTESIAN_POINT ( 'NONE',  ( 9.864935476506833112, -13.90063640520463650, 5.652196082367002106 ) ) ;
#24621=LINE ( 'NONE', #29936, #16073 ) ;
#24622=ORIENTED_EDGE ( 'NONE', *, *, #3854, .T. ) ;
#24625=CARTESIAN_POINT ( 'NONE',  ( 10.27641578865090466, -17.15802603149301220, 6.913388067999417963 ) ) ;
#24626=CARTESIAN_POINT ( 'NONE',  ( -5.973960059363099262, 19.10558826632599860, 7.652108011868850035 ) ) ;
#24627=ORIENTED_EDGE ( 'NONE', *, *, #29018, .F. ) ;
#24631=EDGE_CURVE ( 'NONE', #19956, #17125, #10998, .T. ) ;
#24638=CARTESIAN_POINT ( 'NONE',  ( 16.87938398529693984, 2.193321724558644714, 6.755862304746362845 ) ) ;
#24639=B_SPLINE_CURVE_WITH_KNOTS ( 'NONE', 3,
 ( #7423, #10064, #17547, #27065, #10213, #29093, #19723, #29246, #2588, #12105, #28785, #26450, #5080, #14591, #11149, #8191 ),
 .UNSPECIFIED., .F., .F.,
 ( 4, 2, 2, 2, 2, 2, 2, 4 ),
 ( 0.5000000000000000000, 0.6250000000000013323, 0.6875000000000022204, 0.7187500000000025535, 0.7500000000000028866, 0.8125000000000017764, 0.8750000000000008882, 1.000000000000000000 ),
 .UNSPECIFIED. ) ;
#24640=ORIENTED_EDGE ( 'NONE', *, *, #28308, .F. ) ;
#24641=CARTESIAN_POINT ( 'NONE',  ( 15.11794152162359062, 13.12142272612526206, 5.701226463332907279 ) ) ;
#24644=EDGE_CURVE ( 'NONE', #8165, #13794, #5016, .T. ) ;
#24645=CARTESIAN_POINT ( 'NONE',  ( -4.163336342344337027E-14, 1.387778780781445676E-14, 21.50000000000000000 ) ) ;
#24647=ADVANCED_FACE ( 'NONE', ( #8852 ), #18375, .F. ) ;
#24652=AXIS2_PLACEMENT_3D ( 'NONE', #26093, #14227, #23289 ) ;
#24653=DIRECTION ( 'NONE',  ( 0.000000000000000000, 0.000000000000000000, -1.000000000000000000 ) ) ;
#24654=CARTESIAN_POINT ( 'NONE',  ( 10.28124378133233741, -17.17592898829030901, 19.56050940960062690 ) ) ;
#24660=VERTEX_POINT ( 'NONE', #23340 ) ;
#24664=CARTESIAN_POINT ( 'NONE',  ( 12.44591117076090647, 11.64178973132370487, 7.652108011868854476 ) ) ;
#24667=DIRECTION ( 'NONE',  ( 1.000000000000000000, 0.000000000000000000, 0.000000000000000000 ) ) ;
#24668=DIRECTION ( 'NONE',  ( -0.000000000000000000, -0.000000000000000000, 1.000000000000000000 ) ) ;
#24675=EDGE_LOOP ( 'NONE', ( #2450, #10183, #5050, #23659 ) ) ;
#24677=ORIENTED_EDGE ( 'NONE', *, *, #4787, .T. ) ;
#24682=CARTESIAN_POINT ( 'NONE',  ( -9.056208293496290196, 2.810445847081952664, 1.500000000000001332 ) ) ;
#24684=CYLINDRICAL_SURFACE ( 'NONE', #12779, 0.7499999999999988898 ) ;
#24688=CARTESIAN_POINT ( 'NONE',  ( 0.9359619706472933620, -17.02419289499718502, 5.661398277488801867 ) ) ;
#24690=ORIENTED_EDGE ( 'NONE', *, *, #14387, .T. ) ;
#24692=CARTESIAN_POINT ( 'NONE',  ( -11.06207408980607099, -16.68369011021418302, 20.12545155307891065 ) ) ;
#24693=CARTESIAN_POINT ( 'NONE',  ( -14.81015662609900119, -8.488192507792282626, 7.280727868105637768 ) ) ;
#24694=CARTESIAN_POINT ( 'NONE',  ( -6.485253725360689891, 18.93805017237212951, 7.500147780736496017 ) ) ;
#24696=CARTESIAN_POINT ( 'NONE',  ( 10.38186781339405584, -13.54365823448426553, 7.441806358946449151 ) ) ;
#24701=ORIENTED_EDGE ( 'NONE', *, *, #19859, .T. ) ;
#24702=PLANE ( 'NONE',  #5560 ) ;
#24706=CARTESIAN_POINT ( 'NONE',  ( -0.1790877313959190476, -17.02136788083225838, 6.973843882838226094 ) ) ;
#24708=DIRECTION ( 'NONE',  ( -0.000000000000000000, -0.000000000000000000, 1.000000000000000000 ) ) ;
#24718=AXIS2_PLACEMENT_3D ( 'NONE', #17207, #1142, #20164 ) ;
#24726=CARTESIAN_POINT ( 'NONE',  ( 12.99340803228413144, 10.99622480872967500, 19.60617949693493500 ) ) ;
#24727=CARTESIAN_POINT ( 'NONE',  ( 15.81223572262637589, -6.365019322297389870, 7.652108011868850923 ) ) ;
#24730=CARTESIAN_POINT ( 'NONE',  ( 9.436481611552752113, 0.9307681286968877421, 1.500000000000001332 ) ) ;
#24735=EDGE_LOOP ( 'NONE', ( #11698, #2968, #25555, #9641 ) ) ;
#24736=CYLINDRICAL_SURFACE ( 'NONE', #16261, 1.000000000000004441 ) ;
#24741=VECTOR ( 'NONE', #20618, 1000.000000000000000 ) ;
#24747=DIRECTION ( 'NONE',  ( -0.000000000000000000, -0.000000000000000000, 1.000000000000000000 ) ) ;
#24748=EDGE_LOOP ( 'NONE', ( #12839, #10123, #3546, #16281 ) ) ;
#24749=ORIENTED_EDGE ( 'NONE', *, *, #20483, .T. ) ;
#24750=CARTESIAN_POINT ( 'NONE',  ( -6.028330626922774549, 10.93629592680536788, 1.500000000000001332 ) ) ;
#24753=DIRECTION ( 'NONE',  ( -0.000000000000000000, -0.000000000000000000, 1.000000000000000000 ) ) ;
#24755=DIRECTION ( 'NONE',  ( 1.000000000000000000, 0.000000000000000000, 0.000000000000000000 ) ) ;
#24763=CARTESIAN_POINT ( 'NONE',  ( 19.57285800138751597, 4.196195780087079719, 6.560937769032974209 ) ) ;
#24765=VECTOR ( 'NONE', #26195, 1000.000000000000000 ) ;
#24766=CARTESIAN_POINT ( 'NONE',  ( -9.702532784345956784, -17.50903092980014719, 19.69140814234746273 ) ) ;
#24772=VECTOR ( 'NONE', #18345, 1000.000000000000000 ) ;
#24774=CARTESIAN_POINT ( 'NONE',  ( 9.002475149809910704, -14.44561766934883984, 6.641371103590088865 ) ) ;
#24779=EDGE_CURVE ( 'NONE', #27593, #17088, #12080, .T. ) ;
#24780=ORIENTED_EDGE ( 'NONE', *, *, #25575, .F. ) ;
#24782=CARTESIAN_POINT ( 'NONE',  ( 0.000000000000000000, 0.000000000000000000, 21.50000000000000000 ) ) ;
#24783=CARTESIAN_POINT ( 'NONE',  ( 9.349584168494304848, 12.69858007495367680, 24.50000000000000000 ) ) ;
#24786=CARTESIAN_POINT ( 'NONE',  ( -5.222323004038177174, 16.21609733491351690, 7.595116371587256054 ) ) ;
#24787=VERTEX_POINT ( 'NONE', #15825 ) ;
#24792=CARTESIAN_POINT ( 'NONE',  ( 6.974883619896790954, 5.687793815610376669, 1.500000000000001332 ) ) ;
#24793=EDGE_LOOP ( 'NONE', ( #29660, #29376, #23850, #2048 ) ) ;
#24797=CARTESIAN_POINT ( 'NONE',  ( 16.83479397774492980, 2.565335765644449761, 7.429667576816606278 ) ) ;
#24798=ORIENTED_EDGE ( 'NONE', *, *, #30525, .T. ) ;
#24801=ORIENTED_EDGE ( 'NONE', *, *, #27256, .F. ) ;
#24802=AXIS2_PLACEMENT_3D ( 'NONE', #1178, #30024, #1642 ) ;
#24808=CARTESIAN_POINT ( 'NONE',  ( 4.454645749177148062, 19.51581340210660187, 6.131018562779544823 ) ) ;
#24814=DIRECTION ( 'NONE',  ( 0.000000000000000000, 0.000000000000000000, -1.000000000000000000 ) ) ;
#24816=CARTESIAN_POINT ( 'NONE',  ( 11.00066062335189621, -16.70338693167702004, 18.34726407865098707 ) ) ;
#24821=CARTESIAN_POINT ( 'NONE',  ( -13.87349289520723339, 9.945669722324359086, 19.97651184436794125 ) ) ;
#24823=EDGE_CURVE ( 'NONE', #16110, #2810, #28849, .T. ) ;
#24829=B_SPLINE_SURFACE_WITH_KNOTS ( 'NONE', 3, 1, ( 
 ( #17290, #16834 ),
 ( #19622, #29309 ),
 ( #26977, #5603 ),
 ( #26349, #14641 ),
 ( #24613, #9973 ),
 ( #3246, #23986 ),
 ( #9656, #21495 ),
 ( #136, #12154 ),
 ( #21653, #287 ),
 ( #9812, #456 ),
 ( #19325, #28846 ),
 ( #24143, #7481 ),
 ( #14791, #19477 ),
 ( #16977, #28991 ),
 ( #7625, #2960 ),
 ( #26654, #30072 ),
 ( #11049, #17754 ),
 ( #5746, #15565 ),
 ( #24766, #15888 ),
 ( #3882, #20098 ),
 ( #27274, #917 ),
 ( #29929, #6213 ),
 ( #1539, #5906 ),
 ( #15717, #15406 ),
 ( #25083, #24930 ),
 ( #25235, #8099 ),
 ( #15237, #8710 ),
 ( #3727, #17923 ),
 ( #22731, #13089 ),
 ( #3412, #27436 ),
 ( #20550, #10584 ) ),
 .UNSPECIFIED., .F., .F., .F.,
 ( 4, 3, 3, 3, 3, 3, 3, 3, 3, 3, 4 ),
 ( 2, 2 ),
 ( 0.4999999998345688312, 0.5360336730431939367, 0.5907651151589012883, 0.6456034593241830599, 0.6998270958050434309, 0.7529536536315937223, 0.8052385063053260073, 0.8575343587103997356, 0.9106564858195042023, 0.9648414833209685293, 1.000000006602610236 ),
 ( 0.000000000000000000, 1.000000000000000000 ),
 .UNSPECIFIED. ) ;
#24830=DIRECTION ( 'NONE',  ( 0.000000000000000000, 0.000000000000000000, 1.000000000000000000 ) ) ;
#24834=AXIS2_PLACEMENT_3D ( 'NONE', #25048, #6328, #27702 ) ;
#24835=EDGE_CURVE ( 'NONE', #10944, #4071, #553, .T. ) ;
#24836=DIRECTION ( 'NONE',  ( -0.000000000000000000, -0.000000000000000000, 1.000000000000000000 ) ) ;
#24840=DIRECTION ( 'NONE',  ( 1.000000000000000000, 0.000000000000000000, 0.000000000000000000 ) ) ;
#24845=ORIENTED_EDGE ( 'NONE', *, *, #28978, .F. ) ;
#24846=DIRECTION ( 'NONE',  ( 1.000000000000000000, 0.000000000000000000, 0.000000000000000000 ) ) ;
#24848=ORIENTED_EDGE ( 'NONE', *, *, #17374, .F. ) ;
#24854=DIRECTION ( 'NONE',  ( 1.000000000000000000, 0.000000000000000000, 0.000000000000000000 ) ) ;
#24857=LINE ( 'NONE', #27046, #18391 ) ;
#24859=CARTESIAN_POINT ( 'NONE',  ( 12.25849595087226085, 11.84990609407550721, 20.33971507717571114 ) ) ;
#24861=EDGE_CURVE ( 'NONE', #17088, #8561, #10435, .T. ) ;
#24862=ORIENTED_EDGE ( 'NONE', *, *, #8848, .T. ) ;
#24863=EDGE_CURVE ( 'NONE', #9060, #29096, #28993, .T. ) ;
#24865=CARTESIAN_POINT ( 'NONE',  ( -8.925879454855031980, -14.50801274514188322, 20.25336174263950184 ) ) ;
#24866=CARTESIAN_POINT ( 'NONE',  ( -17.73902742151046752, -9.275718677609276597, 7.366751648393900176 ) ) ;
#24867=EDGE_CURVE ( 'NONE', #26243, #22916, #26499, .T. ) ;
#24868=CARTESIAN_POINT ( 'NONE',  ( -5.058868514924372839, 16.26385723641531555, 7.526951045817046548 ) ) ;
#24869=CARTESIAN_POINT ( 'NONE',  ( 10.31307689846358677, -13.59231953480260024, 5.810767894563978686 ) ) ;
#24877=CARTESIAN_POINT ( 'NONE',  ( -12.96684546537104765, 11.03909700805841609, 5.862424720655265098 ) ) ;
#24878=CARTESIAN_POINT ( 'NONE',  ( 0.7836604620899301210, -17.02735026737548552, 5.652196082368483587 ) ) ;
#24880=CARTESIAN_POINT ( 'NONE',  ( 4.045242219987652987, 16.55840560649981441, 5.652196082368482699 ) ) ;
#24883=CARTESIAN_POINT ( 'NONE',  ( 9.169883732660084164, -9.268939115642975679, 1.500000000000001332 ) ) ;
#24892=DIRECTION ( 'NONE',  ( 0.6548607339452783282, -0.7557495743542641531, 0.000000000000000000 ) ) ;
#24894=ORIENTED_EDGE ( 'NONE', *, *, #5961, .F. ) ;
#24898=CARTESIAN_POINT ( 'NONE',  ( -8.884323311075783991, -1.438332125858144295, 1.500000000000001332 ) ) ;
#24902=CARTESIAN_POINT ( 'NONE',  ( -7.028330626922778990, 10.93629592680536788, 1.500000000000001332 ) ) ;
#24903=AXIS2_PLACEMENT_3D ( 'NONE', #30612, #11750, #21244 ) ;
#24912=DIRECTION ( 'NONE',  ( 0.000000000000000000, 0.000000000000000000, 1.000000000000000000 ) ) ;
#24915=CARTESIAN_POINT ( 'NONE',  ( -16.92011235424303806, 1.986018190673853434, 7.595116371587256054 ) ) ;
#24916=CARTESIAN_POINT ( 'NONE',  ( 18.12802117124498835, -8.449244086891155803, 7.526993102356316356 ) ) ;
#24917=LINE ( 'NONE', #23170, #4846 ) ;
#24918=DIRECTION ( 'NONE',  ( 1.000000000000000000, 0.000000000000000000, 0.000000000000000000 ) ) ;
#24921=DIRECTION ( 'NONE',  ( 1.000000000000000000, 0.000000000000000000, 0.000000000000000000 ) ) ;
#24922=EDGE_LOOP ( 'NONE', ( #10963, #14461 ) ) ;
#24925=ORIENTED_EDGE ( 'NONE', *, *, #2199, .F. ) ;
#24928=CARTESIAN_POINT ( 'NONE',  ( 16.71770988170262129, 3.349230485916621092, 5.661398277488801867 ) ) ;
#24930=CARTESIAN_POINT ( 'NONE',  ( -8.089106849613330041, -15.02215080929124369, 20.19593175699879595 ) ) ;
#24931=DIRECTION ( 'NONE',  ( -1.000000000000000000, 0.000000000000000000, 0.000000000000000000 ) ) ;
#24932=CARTESIAN_POINT ( 'NONE',  ( -9.390093949357552816, -14.19700018541241882, 6.782064869129510676 ) ) ;
#24934=ORIENTED_EDGE ( 'NONE', *, *, #8534, .T. ) ;
#24936=CARTESIAN_POINT ( 'NONE',  ( 10.23384659304339017, -13.64843352988229519, 18.44527579819791185 ) ) ;
#24939=VERTEX_POINT ( 'NONE', #458 ) ;
#24942=CARTESIAN_POINT ( 'NONE',  ( -5.225937649208977298, 16.21530267322276941, 5.701226463332907279 ) ) ;
#24950=CARTESIAN_POINT ( 'NONE',  ( 14.34755844633281363, 13.95901041572539292, 6.041646659195333058 ) ) ;
#24951=CARTESIAN_POINT ( 'NONE',  ( 19.86222817340373226, 2.491431357970654403, 5.940635272151477686 ) ) ;
#24952=VERTEX_POINT ( 'NONE', #599 ) ;
#24955=DIRECTION ( 'NONE',  ( 1.000000000000000000, 0.000000000000000000, 0.000000000000000000 ) ) ;
#24961=CARTESIAN_POINT ( 'NONE',  ( 3.978203543573296308, 16.57681993851655733, 7.652108011868850035 ) ) ;
#24967=CARTESIAN_POINT ( 'NONE',  ( -4.163336342344337027E-14, 1.387778780781445676E-14, 24.50000000000000000 ) ) ;
#24968=VERTEX_POINT ( 'NONE', #22274 ) ;
#24970=CARTESIAN_POINT ( 'NONE',  ( 15.63062718528785489, -6.770321384568316780, 7.557577766377196582 ) ) ;
#24973=EDGE_LOOP ( 'NONE', ( #15197, #17094, #22100, #29239 ) ) ;
#24975=CARTESIAN_POINT ( 'NONE',  ( -4.163336342344337027E-14, 1.387778780781445676E-14, 1.500000000000000000 ) ) ;
#24976=DIRECTION ( 'NONE',  ( 0.000000000000000000, 0.000000000000000000, 1.000000000000000000 ) ) ;
#24977=CARTESIAN_POINT ( 'NONE',  ( 12.53055695656565582, 11.54555247029871268, 5.676815824193228721 ) ) ;
#24979=CARTESIAN_POINT ( 'NONE',  ( -6.187077094091591789, 11.47693674426096955, 24.50000000000000000 ) ) ;
#24981=CARTESIAN_POINT ( 'NONE',  ( 16.74328841314637017, 3.194145055459935545, 7.652108011868850923 ) ) ;
#24983=ADVANCED_FACE ( 'NONE', ( #17608 ), #290, .F. ) ;
#24986=CARTESIAN_POINT ( 'NONE',  ( 6.630478080506912342, 6.778663211761485563, 21.50000000000000000 ) ) ;
#24989=EDGE_CURVE ( 'NONE', #6567, #3146, #7604, .T. ) ;
#24993=CARTESIAN_POINT ( 'NONE',  ( -19.92837724392306242, 1.693712106646816151, 19.96797677718663522 ) ) ;
#24994=VERTEX_POINT ( 'NONE', #20699 ) ;
#24996=EDGE_CURVE ( 'NONE', #1715, #1564, #15567, .T. ) ;
#24998=EDGE_CURVE ( 'NONE', #27915, #24299, #8531, .T. ) ;
#25005=CARTESIAN_POINT ( 'NONE',  ( 12.06031594364850967, 12.06435167025951749, 20.25542030744407640 ) ) ;
#25010=CARTESIAN_POINT ( 'NONE',  ( -11.24862133554823274, -16.55851774953665867, 19.87181966307587544 ) ) ;
#25012=CARTESIAN_POINT ( 'NONE',  ( -5.964083977939222514, 15.98216206238708637, 7.559636331181775581 ) ) ;
#25013=ADVANCED_FACE ( 'NONE', ( #20408 ), #15613, .T. ) ;
#25014=CARTESIAN_POINT ( 'NONE',  ( 9.991354877675743040, -13.81564317159775968, 5.661398277488802755 ) ) ;
#25016=CARTESIAN_POINT ( 'NONE',  ( -5.393256883115301825, -14.81828060999315433, 24.50000000000000000 ) ) ;
#25017=ORIENTED_EDGE ( 'NONE', *, *, #4026, .T. ) ;
#25021=CARTESIAN_POINT ( 'NONE',  ( -14.75808792347767984, 13.52460813173914289, 6.211014596808754007 ) ) ;
#25022=LINE ( 'NONE', #3663, #19562 ) ;
#25023=ORIENTED_EDGE ( 'NONE', *, *, #12838, .F. ) ;
#25025=CARTESIAN_POINT ( 'NONE',  ( -11.13550902248300467, -16.63501148641496030, 7.359006845440219102 ) ) ;
#25027=ORIENTED_EDGE ( 'NONE', *, *, #20075, .T. ) ;
#25030=ADVANCED_FACE ( 'NONE', ( #26010 ), #13999, .F. ) ;
#25033=CARTESIAN_POINT ( 'NONE',  ( 9.454746441592959627, -0.7220001660362816986, 13.00000000000000178 ) ) ;
#25034=EDGE_CURVE ( 'NONE', #1255, #24968, #21148, .T. ) ;
#25035=CARTESIAN_POINT ( 'NONE',  ( 1.964582201835851638, -2.267248723062833538, 24.50000000000000000 ) ) ;
#25036=CARTESIAN_POINT ( 'NONE',  ( -19.82706496683077191, 2.627678016133617955, 20.34789198813115618 ) ) ;
#25038=DIRECTION ( 'NONE',  ( 1.000000000000000000, 0.000000000000000000, 0.000000000000000000 ) ) ;
#25040=CIRCLE ( 'NONE', #14637, 0.7500000000000006661 ) ;
#25041=DIRECTION ( 'NONE',  ( 1.000000000000000000, 0.000000000000000000, 0.000000000000000000 ) ) ;
#25043=EDGE_CURVE ( 'NONE', #21089, #6958, #30385, .T. ) ;
#25048=CARTESIAN_POINT ( 'NONE',  ( -2.703030265324078307, -12.75514121382991384, 1.500000000000001332 ) ) ;
#25051=CARTESIAN_POINT ( 'NONE',  ( -9.824744466605366711, -8.513189541288717521, 1.500000000000001332 ) ) ;
#25054=DIRECTION ( 'NONE',  ( 1.000000000000000000, 0.000000000000000000, 0.000000000000000000 ) ) ;
#25056=EDGE_CURVE ( 'NONE', #4949, #6035, #19485, .T. ) ;
#25061=CARTESIAN_POINT ( 'NONE',  ( 9.864937699929956949, -13.90063973435163724, 18.34798005863078885 ) ) ;
#25065=FACE_OUTER_BOUND ( 'NONE', #5379, .T. ) ;
#25067=CARTESIAN_POINT ( 'NONE',  ( 15.28831480992544911, 12.89481865072260547, 7.454139397117724997 ) ) ;
#25075=CARTESIAN_POINT ( 'NONE',  ( 4.622016212553096359, -12.19167610014704906, 1.500000000000001332 ) ) ;
#25077=CARTESIAN_POINT ( 'NONE',  ( -5.976020107417636673, 19.08630880174946043, 18.34798005863226678 ) ) ;
#25079=B_SPLINE_SURFACE_WITH_KNOTS ( 'NONE', 3, 1, ( 
 ( #23764, #21735 ),
 ( #377, #12556 ),
 ( #21900, #7240 ),
 ( #10052, #5066 ),
 ( #9896, #7094 ),
 ( #9733, #19560 ),
 ( #19411, #9443 ),
 ( #14720, #16601 ),
 ( #26114, #26593 ),
 ( #4907, #19246 ),
 ( #4743, #14575 ),
 ( #7721, #17218 ),
 ( #28928, #26743 ),
 ( #5372, #7562 ),
 ( #14246, #21434 ),
 ( #76, #14425 ),
 ( #28770, #7409 ),
 ( #16917, #26433 ),
 ( #15026, #15645 ),
 ( #22046, #8338 ),
 ( #20020, #10826 ),
 ( #15493, #24693 ),
 ( #24866, #5678 ),
 ( #1149, #27200 ),
 ( #12708, #27516 ),
 ( #8506, #20170 ),
 ( #27051, #27370 ),
 ( #29393, #18008 ),
 ( #841, #19708 ),
 ( #10662, #17852 ),
 ( #8028, #3649 ) ),
 .UNSPECIFIED., .F., .F., .F.,
 ( 4, 3, 3, 3, 3, 3, 3, 3, 3, 3, 4 ),
 ( 2, 2 ),
 ( 0.4999999998345686647, 0.5360336730431942698, 0.5907651151589017324, 0.6456034593241839481, 0.6998270958050443191, 0.7529536536315944995, 0.8052385063053264513, 0.8575343587103996246, 0.9106564858195047574, 0.9648414833209688624, 1.000000006602610014 ),
 ( 0.000000000000000000, 1.000000000000000000 ),
 .UNSPECIFIED. ) ;
#25083=CARTESIAN_POINT ( 'NONE',  ( -10.06548534245863280, -17.30301317789300697, 20.19593175699879595 ) ) ;
#25084=CARTESIAN_POINT ( 'NONE',  ( -17.06581907267799636, 0.6464955982430669046, 19.21769074125272425 ) ) ;
#25086=CARTESIAN_POINT ( 'NONE',  ( -8.550548372801092256, -14.74545326687210611, 7.652108011868850923 ) ) ;
#25090=DIRECTION ( 'NONE',  ( 1.000000000000000000, 0.000000000000000000, 0.000000000000000000 ) ) ;
#25094=EDGE_LOOP ( 'NONE', ( #22529, #12765 ) ) ;
#25097=CARTESIAN_POINT ( 'NONE',  ( -4.850186825639134724, 16.32197540402033198, 7.359006845440219102 ) ) ;
#25098=EDGE_LOOP ( 'NONE', ( #22699, #1981, #8998, #11776 ) ) ;
#25107=CARTESIAN_POINT ( 'NONE',  ( -1.195154792889458806, -9.406652940105983518, 1.500000000000001332 ) ) ;
#25111=ORIENTED_EDGE ( 'NONE', *, *, #25197, .T. ) ;
#25112=CARTESIAN_POINT ( 'NONE',  ( -16.46198811862381817, -1.356593340923033075, 1.500000000000000000 ) ) ;
#25116=CARTESIAN_POINT ( 'NONE',  ( 0.000000000000000000, 0.000000000000000000, 21.50000000000000000 ) ) ;
#25118=EDGE_LOOP ( 'NONE', ( #14858, #16062, #20721, #14928 ) ) ;
#25120=CARTESIAN_POINT ( 'NONE',  ( 9.801156115998399088, -13.94312737849039330, 18.34969686940296185 ) ) ;
#25123=CARTESIAN_POINT ( 'NONE',  ( -19.84651427434118176, 2.615565199888951753, 20.34789198813115263 ) ) ;
#25124=CARTESIAN_POINT ( 'NONE',  ( 15.71976421978571459, -6.574744378264575140, 7.632642797338977658 ) ) ;
#25125=CARTESIAN_POINT ( 'NONE',  ( -13.88241978398541221, 9.934084310449181388, 6.041646659195333058 ) ) ;
#25126=CARTESIAN_POINT ( 'NONE',  ( 3.529212228261827011, 16.69261290539733977, 20.19593175699879595 ) ) ;
#25131=CARTESIAN_POINT ( 'NONE',  ( -4.661329110590011204, 16.37253524622244427, 19.77662771831109367 ) ) ;
#25141=ORIENTED_EDGE ( 'NONE', *, *, #6377, .T. ) ;
#25142=CARTESIAN_POINT ( 'NONE',  ( -4.608906612435655248, -7.730328572437724866, 21.50000000000000000 ) ) ;
#25144=CARTESIAN_POINT ( 'NONE',  ( -19.90071050938331609, 1.994113959836040451, 20.22386025856690139 ) ) ;
#25147=AXIS2_PLACEMENT_3D ( 'NONE', #30051, #8692, #22561 ) ;
#25148=DIRECTION ( 'NONE',  ( 1.000000000000000000, 0.000000000000000000, 0.000000000000000000 ) ) ;
#25153=CARTESIAN_POINT ( 'NONE',  ( 1.367976436446960875, -19.97081545247029410, 6.560937769032974209 ) ) ;
#25154=DIRECTION ( 'NONE',  ( 1.000000000000000000, 0.000000000000000000, 0.000000000000000000 ) ) ;
#25156=CARTESIAN_POINT ( 'NONE',  ( -9.081360402260857612, -14.40588898056577705, 18.55820869691756769 ) ) ;
#25159=CARTESIAN_POINT ( 'NONE',  ( -14.70205207497229871, -8.690259054815006934, 19.25672174529527325 ) ) ;
#25170=CYLINDRICAL_SURFACE ( 'NONE', #26082, 20.00000000000000000 ) ;
#25173=CARTESIAN_POINT ( 'NONE',  ( -10.55542352351189095, -17.00870908956209249, 5.651989602109218858 ) ) ;
#25174=ORIENTED_EDGE ( 'NONE', *, *, #20090, .F. ) ;
#25175=ADVANCED_FACE ( 'NONE', ( #7754 ), #17258, .T. ) ;
#25179=DIRECTION ( 'NONE',  ( 1.000000000000000000, 0.000000000000000000, 0.000000000000000000 ) ) ;
#25183=CARTESIAN_POINT ( 'NONE',  ( 7.548823014270646503, -5.738360882149970976, 21.50000000000000000 ) ) ;
#25186=CIRCLE ( 'NONE', #28687, 9.482273699623480212 ) ;
#25187=CARTESIAN_POINT ( 'NONE',  ( 8.999114229549594057, -0.1262659238204522361, 21.50000000000000000 ) ) ;
#25188=CARTESIAN_POINT ( 'NONE',  ( 0.3567147238643519902, -19.99681861211371370, 18.34798005863226678 ) ) ;
#25191=CARTESIAN_POINT ( 'NONE',  ( -17.05026832884990995, 0.8441673869621679760, 6.037360021877316463 ) ) ;
#25192=LINE ( 'NONE', #16602, #8850 ) ;
#25197=EDGE_CURVE ( 'NONE', #16236, #9004, #13517, .T. ) ;
#25200=CARTESIAN_POINT ( 'NONE',  ( -9.072316094201720915, -14.41194981467785929, 20.14907003336612945 ) ) ;
#25207=EDGE_CURVE ( 'NONE', #8705, #27809, #15498, .T. ) ;
#25209=CARTESIAN_POINT ( 'NONE',  ( -6.458576814772031049, 15.80792270644134767, 19.02573955821369367 ) ) ;
#25210=DIRECTION ( 'NONE',  ( 0.000000000000000000, 0.000000000000000000, 1.000000000000000000 ) ) ;
#25215=VERTEX_POINT ( 'NONE', #13521 ) ;
#25216=CARTESIAN_POINT ( 'NONE',  ( -11.35972605147144598, -16.46076013017338013, 19.21471108562412766 ) ) ;
#25220=CARTESIAN_POINT ( 'NONE',  ( -8.832446728800206870, -14.56826516372322367, 18.39701043959520987 ) ) ;
#25226=CARTESIAN_POINT ( 'NONE',  ( -16.84890868872602354, 2.447051129731594887, 18.72771030977187579 ) ) ;
#25228=ORIENTED_EDGE ( 'NONE', *, *, #18508, .F. ) ;
#25233=FACE_OUTER_BOUND ( 'NONE', #1224, .T. ) ;
#25235=CARTESIAN_POINT ( 'NONE',  ( -10.14924625765044119, -17.25430667454972067, 20.25542030744407640 ) ) ;
#25236=DIRECTION ( 'NONE',  ( 0.9898214418809327952, -0.1423148382732850048, 0.000000000000000000 ) ) ;
#25237=CARTESIAN_POINT ( 'NONE',  ( -17.00515754968433768, 1.312003563659740690, 18.39992786714538298 ) ) ;
#25239=VERTEX_POINT ( 'NONE', #17714 ) ;
#25241=EDGE_CURVE ( 'NONE', #24237, #20108, #30189, .T. ) ;
#25246=ORIENTED_EDGE ( 'NONE', *, *, #14151, .F. ) ;
#25248=CYLINDRICAL_SURFACE ( 'NONE', #13641, 0.7500000000000006661 ) ;
#25249=CARTESIAN_POINT ( 'NONE',  ( -4.673829994069186533, 16.36915245889226256, 6.211014596808754007 ) ) ;
#25254=CARTESIAN_POINT ( 'NONE',  ( -12.79952941389652921, 11.22436372988652664, 6.143977687428009204 ) ) ;
#25256=LINE ( 'NONE', #29794, #18895 ) ;
#25259=AXIS2_PLACEMENT_3D ( 'NONE', #13982, #1670, #9005 ) ;
#25262=AXIS2_PLACEMENT_3D ( 'NONE', #10302, #5636, #14827 ) ;
#25263=CARTESIAN_POINT ( 'NONE',  ( 12.57902516942791671, 11.48976026227458291, 5.701226463332907279 ) ) ;
#25265=CARTESIAN_POINT ( 'NONE',  ( -13.37849590498012553, 10.56201291617987792, 20.34789198813115263 ) ) ;
#25268=ORIENTED_EDGE ( 'NONE', *, *, #14679, .F. ) ;
#25270=EDGE_CURVE ( 'NONE', #5874, #21024, #11017, .T. ) ;
#25271=DIRECTION ( 'NONE',  ( 1.000000000000000000, 0.000000000000000000, 0.000000000000000000 ) ) ;
#25272=CARTESIAN_POINT ( 'NONE',  ( 6.237549684377466264, 19.00251437819607858, 19.60917204426171523 ) ) ;
#25277=CARTESIAN_POINT ( 'NONE',  ( 9.138492726993298731, -14.36378254522091780, 18.80699882434806369 ) ) ;
#25278=DIRECTION ( 'NONE',  ( 1.000000000000000000, 0.000000000000000000, 0.000000000000000000 ) ) ;
#25280=AXIS2_PLACEMENT_3D ( 'NONE', #24343, #5639, #3285 ) ;
#25283=VECTOR ( 'NONE', #27303, 1000.000000000000227 ) ;
#25285=CARTESIAN_POINT ( 'NONE',  ( 5.303644920943711760, 19.30240823413181062, 20.34789198813115263 ) ) ;
#25286=EDGE_LOOP ( 'NONE', ( #27111, #22027, #1829, #29101 ) ) ;
#25291=CARTESIAN_POINT ( 'NONE',  ( -5.205279254987321025, 19.32936484843851588, 19.96783386855779341 ) ) ;
#25294=FACE_OUTER_BOUND ( 'NONE', #24922, .T. ) ;
#25298=ORIENTED_EDGE ( 'NONE', *, *, #21799, .F. ) ;
#25299=VECTOR ( 'NONE', #18305, 1000.000000000000000 ) ;
#25303=CARTESIAN_POINT ( 'NONE',  ( 19.74328841314634886, 3.194145055459934213, 20.34789198813115263 ) ) ;
#25305=VERTEX_POINT ( 'NONE', #29897 ) ;
#25308=DIRECTION ( 'NONE',  ( 0.1423148382732889183, 0.9898214418809321291, 0.000000000000000000 ) ) ;
#25310=CARTESIAN_POINT ( 'NONE',  ( -0.4553004113513133833, -19.99503986737293815, 7.267242832833950672 ) ) ;
#25311=VECTOR ( 'NONE', #21102, 1000.000000000000227 ) ;
#25315=CARTESIAN_POINT ( 'NONE',  ( 15.43499236066653779, -3.229500095980125440, 1.500000000000001332 ) ) ;
#25317=CARTESIAN_POINT ( 'NONE',  ( -16.89625272878625140, 2.150609578402132183, 5.774779864094945481 ) ) ;
#25318=ORIENTED_EDGE ( 'NONE', *, *, #1002, .F. ) ;
#25320=AXIS2_PLACEMENT_3D ( 'NONE', #13158, #22359, #15486 ) ;
#25323=CARTESIAN_POINT ( 'NONE',  ( -6.028330626922774549, 10.93629592680536788, 24.50000000000000000 ) ) ;
#25325=CARTESIAN_POINT ( 'NONE',  ( -15.06439250341027147, -7.989583865232170012, 18.37415474056476938 ) ) ;
#25329=ORIENTED_EDGE ( 'NONE', *, *, #7744, .F. ) ;
#25336=CARTESIAN_POINT ( 'NONE',  ( 3.089102459999460315, 16.79563822435759590, 6.917457548096561659 ) ) ;
#25338=DIRECTION ( 'NONE',  ( -0.000000000000000000, -0.000000000000000000, 1.000000000000000000 ) ) ;
#25340=CIRCLE ( 'NONE', #30810, 0.7500000000000024425 ) ;
#25346=CARTESIAN_POINT ( 'NONE',  ( 11.10715495309692891, -16.63223102436628409, 7.652108011868850035 ) ) ;
#25350=CARTESIAN_POINT ( 'NONE',  ( 0.7836603910024348973, -17.02734626465442247, 18.34798005862662507 ) ) ;
#25351=ORIENTED_EDGE ( 'NONE', *, *, #80, .T. ) ;
#25359=EDGE_CURVE ( 'NONE', #3526, #17261, #576, .T. ) ;
#25363=CARTESIAN_POINT ( 'NONE',  ( 7.974144905643788306, 5.130938270761631337, 1.500000000000001332 ) ) ;
#25364=CARTESIAN_POINT ( 'NONE',  ( 19.78337026033623403, 2.938244205458795388, 5.676722608126685721 ) ) ;
#25365=CARTESIAN_POINT ( 'NONE',  ( -9.395142731145691428, -14.19351217900080719, 19.21496526180053976 ) ) ;
#25369=B_SPLINE_CURVE_WITH_KNOTS ( 'NONE', 3,
 ( #8226, #27419, #6036, #15545, #18050, #25209, #9459, #23474, #25678, #9140, #20975, #25835, #23166, #6794, #16621, #16319 ),
 .UNSPECIFIED., .F., .F.,
 ( 4, 2, 2, 2, 2, 2, 2, 4 ),
 ( 0.5000000000000001110, 0.6250000000000007772, 0.6875000000000013323, 0.7187500000000017764, 0.7500000000000022204, 0.8125000000000015543, 0.8750000000000006661, 1.000000000000000000 ),
 .UNSPECIFIED. ) ;
#25378=CARTESIAN_POINT ( 'NONE',  ( 5.687793815610356241, -6.974883619896809606, 1.500000000000001332 ) ) ;
#25379=ORIENTED_EDGE ( 'NONE', *, *, #9404, .T. ) ;
#25381=CARTESIAN_POINT ( 'NONE',  ( -11.03465445395214672, -16.68068344163647510, 18.54479204710284890 ) ) ;
#25394=ORIENTED_EDGE ( 'NONE', *, *, #23124, .F. ) ;
#25395=DIRECTION ( 'NONE',  ( -0.5406408174555976665, 0.8412535328311812055, 0.000000000000000000 ) ) ;
#25399=CARTESIAN_POINT ( 'NONE',  ( 16.68770897235365780, 3.522277800415036353, 7.603368798681074736 ) ) ;
#25400=CARTESIAN_POINT ( 'NONE',  ( 1.588511040490847792, -16.99700008610011182, 7.269896094239231665 ) ) ;
#25403=CARTESIAN_POINT ( 'NONE',  ( -9.290115248528675096, -14.26557846602795188, 7.156916968540300239 ) ) ;
#25404=DIRECTION ( 'NONE',  ( 0.000000000000000000, 0.000000000000000000, -1.000000000000000000 ) ) ;
#25405=ORIENTED_EDGE ( 'NONE', *, *, #14566, .F. ) ;
#25406=EDGE_CURVE ( 'NONE', #15501, #11969, #16148, .T. ) ;
#25412=ORIENTED_EDGE ( 'NONE', *, *, #29419, .F. ) ;
#25415=CARTESIAN_POINT ( 'NONE',  ( -4.626122995383915359, 16.38173570853530592, 6.310736198168394928 ) ) ;
#25416=VERTEX_POINT ( 'NONE', #13815 ) ;
#25417=CARTESIAN_POINT ( 'NONE',  ( 11.61739189738757894, -16.28020533589261376, 20.15039051365864253 ) ) ;
#25430=ORIENTED_EDGE ( 'NONE', *, *, #189, .F. ) ;
#25433=EDGE_LOOP ( 'NONE', ( #12690, #30505 ) ) ;
#25435=CARTESIAN_POINT ( 'NONE',  ( 4.608906612435600181, 7.730328572437758616, 21.50000000000000000 ) ) ;
#25436=FACE_OUTER_BOUND ( 'NONE', #11255, .T. ) ;
#25439=CARTESIAN_POINT ( 'NONE',  ( 10.30772981839320579, -17.16011447240169474, 19.00652017443069752 ) ) ;
#25440=DIRECTION ( 'NONE',  ( 0.000000000000000000, 0.000000000000000000, 1.000000000000000000 ) ) ;
#25441=ORIENTED_EDGE ( 'NONE', *, *, #3451, .T. ) ;
#25444=CARTESIAN_POINT ( 'NONE',  ( 18.21411928606760711, -8.304179478877907528, 7.595116371587256054 ) ) ;
#25446=CARTESIAN_POINT ( 'NONE',  ( -13.59632618586111441, 10.29740991163844832, 5.704143890883081269 ) ) ;
#25447=CARTESIAN_POINT ( 'NONE',  ( 3.215610563331060767, 16.76717343535964133, 19.89182036555910571 ) ) ;
#25449=ORIENTED_EDGE ( 'NONE', *, *, #9192, .F. ) ;
#25451=CARTESIAN_POINT ( 'NONE',  ( 9.860909914091287476, -13.90333503830274609, 7.652108011868850923 ) ) ;
#25452=CARTESIAN_POINT ( 'NONE',  ( 12.99340803228152197, 10.99622480873287955, 6.910395520694541993 ) ) ;
#25454=CARTESIAN_POINT ( 'NONE',  ( 12.17894461897553526, 11.93905285453845089, 5.653604225791663218 ) ) ;
#25458=EDGE_CURVE ( 'NONE', #1564, #21044, #20489, .T. ) ;
#25459=EDGE_LOOP ( 'NONE', ( #2348, #8799 ) ) ;
#25461=CARTESIAN_POINT ( 'NONE',  ( -17.03429152191317542, 1.023117790763819590, 7.441806358946449151 ) ) ;
#25467=CARTESIAN_POINT ( 'NONE',  ( 18.35307771382468900, -7.992233955150555680, 5.652196082364320695 ) ) ;
#25473=CARTESIAN_POINT ( 'NONE',  ( -0.4522595252855811654, -19.99510590919688013, 6.033082186765056143 ) ) ;
#25476=VECTOR ( 'NONE', #8185, 1000.000000000000000 ) ;
#25477=DIRECTION ( 'NONE',  ( -0.9898214418809327952, 0.1423148382732851158, 0.000000000000000000 ) ) ;
#25478=CARTESIAN_POINT ( 'NONE',  ( -10.51100883930070040, -17.01524884273342764, 18.34798005863226678 ) ) ;
#25483=FACE_OUTER_BOUND ( 'NONE', #28393, .T. ) ;
#25492=FACE_OUTER_BOUND ( 'NONE', #15008, .T. ) ;
#25494=FACE_BOUND ( 'NONE', #2202, .T. ) ;
#25495=ORIENTED_EDGE ( 'NONE', *, *, #21025, .T. ) ;
#25496=CARTESIAN_POINT ( 'NONE',  ( -13.93282946021075830, 9.868441342986791653, 6.147510495896838734 ) ) ;
#25509=CARTESIAN_POINT ( 'NONE',  ( 8.549050687778162683, 4.102102735472488604, 1.500000000000001332 ) ) ;
#25511=ORIENTED_EDGE ( 'NONE', *, *, #9181, .T. ) ;
#25516=CARTESIAN_POINT ( 'NONE',  ( -15.16307827826492449, -7.786259562520723598, 18.34798005863078885 ) ) ;
#25521=CARTESIAN_POINT ( 'NONE',  ( -15.46558767506643761, -7.123678207069782609, 20.05479082170252525 ) ) ;
#25523=VERTEX_POINT ( 'NONE', #22489 ) ;
#25526=DIRECTION ( 'NONE',  ( 0.000000000000000000, 0.000000000000000000, 1.000000000000000000 ) ) ;
#25527=FACE_OUTER_BOUND ( 'NONE', #22936, .T. ) ;
#25531=CARTESIAN_POINT ( 'NONE',  ( 9.343263424981191889, -14.23786665600031576, 18.54473042795395443 ) ) ;
#25536=CARTESIAN_POINT ( 'NONE',  ( -9.958038337755704461, 17.34466697471556884, 24.50000000000000000 ) ) ;
#25539=EDGE_LOOP ( 'NONE', ( #10868, #15758 ) ) ;
#25541=DIRECTION ( 'NONE',  ( 0.000000000000000000, 0.000000000000000000, 1.000000000000000000 ) ) ;
#25544=LINE ( 'NONE', #2281, #30280 ) ;
#25547=CARTESIAN_POINT ( 'NONE',  ( -0.1973194101962248148, -20.01708124257649146, 7.500898271101006820 ) ) ;
#25550=CARTESIAN_POINT ( 'NONE',  ( -9.395348974764877070, -14.19336984580851713, 6.714907520933424578 ) ) ;
#25555=ORIENTED_EDGE ( 'NONE', *, *, #23630, .T. ) ;
#25558=DIRECTION ( 'NONE',  ( 1.000000000000000000, 0.000000000000000000, 0.000000000000000000 ) ) ;
#25559=EDGE_CURVE ( 'NONE', #6583, #5896, #7024, .T. ) ;
#25561=CARTESIAN_POINT ( 'NONE',  ( -5.941992259041530389, 19.11559255287553682, 5.651989602109218858 ) ) ;
#25563=B_SPLINE_CURVE_WITH_KNOTS ( 'NONE', 3,
 ( #23105, #22958, #8628, #20762, #23255, #25310, #3956, #30292, #6442, #13476, #22644, #17995, #25473, #18457, #13758, #27502, #1612, #28110 ),
 .UNSPECIFIED., .F., .F.,
 ( 4, 2, 2, 2, 2, 2, 2, 2, 4 ),
 ( 0.003174295595554301776, 0.003570702171545528901, 0.003967108747536756026, 0.004363515323527983152, 0.004759921899519211144, 0.005156328475510438270, 0.005552735051501665395, 0.005949141627492892520, 0.006345548203484119645 ),
 .UNSPECIFIED. ) ;
#25565=CARTESIAN_POINT ( 'NONE',  ( -13.29453093336401537, 10.66243031773958805, 7.652108011868852699 ) ) ;
#25566=EDGE_CURVE ( 'NONE', #606, #7300, #29961, .T. ) ;
#25567=DIRECTION ( 'NONE',  ( 0.000000000000000000, 0.000000000000000000, 1.000000000000000000 ) ) ;
#25572=EDGE_LOOP ( 'NONE', ( #20610, #12280, #8718, #25268 ) ) ;
#25575=EDGE_CURVE ( 'NONE', #22258, #14561, #27500, .T. ) ;
#25578=ORIENTED_EDGE ( 'NONE', *, *, #4936, .F. ) ;
#25581=EDGE_CURVE ( 'NONE', #20124, #6265, #3059, .T. ) ;
#25590=DIRECTION ( 'NONE',  ( -0.000000000000000000, -0.000000000000000000, 1.000000000000000000 ) ) ;
#25591=CARTESIAN_POINT ( 'NONE',  ( 18.08817148584474310, -8.575141465928741269, 7.429667576816606278 ) ) ;
#25592=CARTESIAN_POINT ( 'NONE',  ( -15.50193441389834881, 12.66492269502747092, 5.678370764302467677 ) ) ;
#25593=CARTESIAN_POINT ( 'NONE',  ( 3.518760595952255876, 16.69517982287620939, 18.50655187082627862 ) ) ;
#25597=ADVANCED_FACE ( 'NONE', ( #18138 ), #27649, .T. ) ;
#25601=CARTESIAN_POINT ( 'NONE',  ( 15.28716501070585565, 12.89617714416416128, 18.54479204710283469 ) ) ;
#25602=CARTESIAN_POINT ( 'NONE',  ( -4.775770841707818626, 16.34206821731733328, 19.96783386855779341 ) ) ;
#25604=CARTESIAN_POINT ( 'NONE',  ( 11.69640250239185342, 12.44177653179680476, 6.329955581934035180 ) ) ;
#25605=ADVANCED_FACE ( 'NONE', ( #9080 ), #28255, .F. ) ;
#25612=CARTESIAN_POINT ( 'NONE',  ( -17.02601880987614535, 1.106972870283160493, 5.810767894563978686 ) ) ;
#25614=LINE ( 'NONE', #27953, #30402 ) ;
#25615=EDGE_CURVE ( 'NONE', #16773, #29972, #6063, .T. ) ;
#25618=ORIENTED_EDGE ( 'NONE', *, *, #1794, .F. ) ;
#25619=EDGE_CURVE ( 'NONE', #25635, #13348, #11718, .T. ) ;
#25629=CARTESIAN_POINT ( 'NONE',  ( -16.93131609043279795, 1.909234121842571019, 5.676815824193228721 ) ) ;
#25630=EDGE_LOOP ( 'NONE', ( #23040, #30538, #19801, #2559 ) ) ;
#25635=VERTEX_POINT ( 'NONE', #16397 ) ;
#25636=FACE_OUTER_BOUND ( 'NONE', #26750, .T. ) ;
#25640=ORIENTED_EDGE ( 'NONE', *, *, #23214, .T. ) ;
#25641=CARTESIAN_POINT ( 'NONE',  ( -4.163336342344337027E-14, 1.387778780781445676E-14, 24.50000000000000000 ) ) ;
#25649=AXIS2_PLACEMENT_3D ( 'NONE', #22181, #19539, #28907 ) ;
#25654=CARTESIAN_POINT ( 'NONE',  ( -8.163758309741957930, -14.97879848885351706, 5.749491821935610147 ) ) ;
#25657=VERTEX_POINT ( 'NONE', #9385 ) ;
#25661=ADVANCED_FACE ( 'NONE', ( #20916 ), #25913, .F. ) ;
#25663=DIRECTION ( 'NONE',  ( 0.000000000000000000, 0.000000000000000000, -1.000000000000000000 ) ) ;
#25665=CARTESIAN_POINT ( 'NONE',  ( -12.79825419741609771, 11.22575876276140505, 19.85270094495842130 ) ) ;
#25669=CARTESIAN_POINT ( 'NONE',  ( -18.15888143814678557, -8.424936462863952258, 20.32842677360128292 ) ) ;
#25672=VERTEX_POINT ( 'NONE', #18903 ) ;
#25673=CARTESIAN_POINT ( 'NONE',  ( -0.7220001660362882490, -9.454746441592959627, 1.500000000000001332 ) ) ;
#25678=CARTESIAN_POINT ( 'NONE',  ( -6.507549961782360448, 15.78987431823413523, 19.28454053338349183 ) ) ;
#25679=CARTESIAN_POINT ( 'NONE',  ( 5.908622583341371026, 19.12614776545568418, 5.862424720655265098 ) ) ;
#25681=CARTESIAN_POINT ( 'NONE',  ( -16.95096719779282424, 1.761153487549136587, 5.657991946698900598 ) ) ;
#25682=DIRECTION ( 'NONE',  ( 1.000000000000000000, 0.000000000000000000, 0.000000000000000000 ) ) ;
#25688=CARTESIAN_POINT ( 'NONE',  ( -14.80112376882104819, -8.505769479164674962, 7.269896094239229889 ) ) ;
#25691=LINE ( 'NONE', #18218, #2380 ) ;
#25692=FACE_OUTER_BOUND ( 'NONE', #11616, .T. ) ;
#25694=CARTESIAN_POINT ( 'NONE',  ( -0.1834311997418870965, -17.02123387943971977, 6.974106381145714018 ) ) ;
#25699=CARTESIAN_POINT ( 'NONE',  ( -17.06612199394662710, 0.6423840055640230862, 19.47783254395485031 ) ) ;
#25701=VERTEX_POINT ( 'NONE', #26683 ) ;
#25713=CARTESIAN_POINT ( 'NONE',  ( -15.73693831436014179, 12.34332084443492938, 18.54958172136248606 ) ) ;
#25718=MECHANICAL_DESIGN_GEOMETRIC_PRESENTATION_REPRESENTATION('',(#26725),#12794);
#25719=ORIENTED_EDGE ( 'NONE', *, *, #2700, .F. ) ;
#25723=EDGE_CURVE ( 'NONE', #12979, #23733, #485, .T. ) ;
#25727=CARTESIAN_POINT ( 'NONE',  ( 0.2758680007052473626, -17.03033689273113183, 18.47056384035244037 ) ) ;
#25730=CARTESIAN_POINT ( 'NONE',  ( 1.743352590885965281, -16.98718212385403348, 19.02573955821369367 ) ) ;
#25731=CARTESIAN_POINT ( 'NONE',  ( 19.79578860058543910, 2.975267875541937723, 18.36582235739946611 ) ) ;
#25734=CARTESIAN_POINT ( 'NONE',  ( 11.11463893384431323, -16.64861865631835514, 7.652108011868850035 ) ) ;
#25735=DIRECTION ( 'NONE',  ( 1.000000000000000000, 0.000000000000000000, 0.000000000000000000 ) ) ;
#25737=CARTESIAN_POINT ( 'NONE',  ( 3.898220458062930049, 16.59828442330440978, 18.35718225375110180 ) ) ;
#25744=EDGE_CURVE ( 'NONE', #13119, #4772, #23481, .T. ) ;
#25747=EDGE_CURVE ( 'NONE', #18622, #11660, #17011, .T. ) ;
#25752=AXIS2_PLACEMENT_3D ( 'NONE', #30271, #27941, #6568 ) ;
#25753=CARTESIAN_POINT ( 'NONE',  ( -16.99143801116385433, 1.432169416036910725, 7.627891251804737927 ) ) ;
#25754=CARTESIAN_POINT ( 'NONE',  ( 14.20332585465777520, 14.08077620357339299, 19.61564845152805603 ) ) ;
#25756=ORIENTED_EDGE ( 'NONE', *, *, #15723, .F. ) ;
#25759=CARTESIAN_POINT ( 'NONE',  ( 18.44211820063743446, -7.784504718833763270, 5.678370764302467677 ) ) ;
#25770=CARTESIAN_POINT ( 'NONE',  ( -6.413028646417897605, 15.82458379172921603, 19.79423548914561692 ) ) ;
#25773=EDGE_CURVE ( 'NONE', #27607, #3383, #6082, .T. ) ;
#25774=DIRECTION ( 'NONE',  ( 1.000000000000000000, 0.000000000000000000, 0.000000000000000000 ) ) ;
#25777=VECTOR ( 'NONE', #755, 1000.000000000000227 ) ;
#25779=CARTESIAN_POINT ( 'NONE',  ( -12.24063095261064227, 4.490763173670005770, 1.500000000000001332 ) ) ;
#25780=EDGE_LOOP ( 'NONE', ( #22416, #12875, #7092, #20839 ) ) ;
#25784=CIRCLE ( 'NONE', #2376, 0.7499999999999997780 ) ;
#25789=AXIS2_PLACEMENT_3D ( 'NONE', #14247, #1957, #9277 ) ;
#25792=EDGE_CURVE ( 'NONE', #28054, #19044, #3595, .T. ) ;
#25795=FACE_BOUND ( 'NONE', #694, .T. ) ;
#25796=ORIENTED_EDGE ( 'NONE', *, *, #17216, .F. ) ;
#25799=CARTESIAN_POINT ( 'NONE',  ( -9.454746441592954298, 0.7220001660363423168, 1.500000000000001332 ) ) ;
#25800=LINE ( 'NONE', #28138, #30852 ) ;
#25808=CARTESIAN_POINT ( 'NONE',  ( -7.931808866138727154, -15.11281102451792080, 7.366751648393900176 ) ) ;
#25811=CARTESIAN_POINT ( 'NONE',  ( 1.709141304117141047, -16.98942507101831012, 18.92976555901915603 ) ) ;
#25813=CARTESIAN_POINT ( 'NONE',  ( 18.57491549710359635, -7.414944001931016437, 7.454606537396340826 ) ) ;
#25814=CARTESIAN_POINT ( 'NONE',  ( 12.93167884983506610, 11.07185515090903749, 18.83976166372256245 ) ) ;
#25820=CARTESIAN_POINT ( 'NONE',  ( -15.37673962019493956, -7.325595981656340960, 18.47056384035244747 ) ) ;
#25821=FACE_OUTER_BOUND ( 'NONE', #2788, .T. ) ;
#25823=CARTESIAN_POINT ( 'NONE',  ( -4.163336342344337027E-14, 1.387778780781445676E-14, 24.50000000000000000 ) ) ;
#25825=CARTESIAN_POINT ( 'NONE',  ( 9.755266892098159559, -13.97392213622798707, 5.651492010659114662 ) ) ;
#25827=VERTEX_POINT ( 'NONE', #22883 ) ;
#25830=CARTESIAN_POINT ( 'NONE',  ( -8.097046320181942036, -15.01856385382801129, 5.759928666072747561 ) ) ;
#25831=FACE_OUTER_BOUND ( 'NONE', #3570, .T. ) ;
#25832=ORIENTED_EDGE ( 'NONE', *, *, #11452, .F. ) ;
#25835=CARTESIAN_POINT ( 'NONE',  ( -6.384540597184203747, 15.83495921351375735, 19.85459532544248162 ) ) ;
#25837=CIRCLE ( 'NONE', #12390, 20.00000000000000000 ) ;
#25838=CARTESIAN_POINT ( 'NONE',  ( 5.413395986729065079, 19.27227163692344902, 7.652108011868850035 ) ) ;
#25839=EDGE_CURVE ( 'NONE', #1882, #30491, #12265, .T. ) ;
#25840=VERTEX_POINT ( 'NONE', #27889 ) ;
#25841=CARTESIAN_POINT ( 'NONE',  ( -16.95590486909633654, 1.723587065725475265, 5.653912893140659257 ) ) ;
#25842=FACE_OUTER_BOUND ( 'NONE', #26369, .T. ) ;
#25849=CARTESIAN_POINT ( 'NONE',  ( -14.79998981352115983, -8.507912210563924660, 6.037360021877317351 ) ) ;
#25850=CARTESIAN_POINT ( 'NONE',  ( -7.974144905643821168, -5.130938270761581599, 21.50000000000000000 ) ) ;
#25857=FACE_OUTER_BOUND ( 'NONE', #21675, .T. ) ;
#25858=CARTESIAN_POINT ( 'NONE',  ( 7.856594496258195726, 4.390207617113981442, 21.50000000000000000 ) ) ;
#25859=CARTESIAN_POINT ( 'NONE',  ( -19.89984252009588062, 2.172142757504853972, 20.29915277494337644 ) ) ;
#25861=ORIENTED_EDGE ( 'NONE', *, *, #8693, .T. ) ;
#25862=CARTESIAN_POINT ( 'NONE',  ( 10.13630142350640462, -13.71646693216190371, 20.29915277494337644 ) ) ;
#25877=ORIENTED_EDGE ( 'NONE', *, *, #26976, .F. ) ;
#25880=ORIENTED_EDGE ( 'NONE', *, *, #12606, .F. ) ;
#25884=CARTESIAN_POINT ( 'NONE',  ( -17.59500444164590149, -9.508866521682284301, 6.919864475265789849 ) ) ;
#25885=CIRCLE ( 'NONE', #29391, 0.7500000000000006661 ) ;
#25886=CARTESIAN_POINT ( 'NONE',  ( -14.76516729830842500, -8.573104839187553949, 19.85459532544248162 ) ) ;
#25887=CARTESIAN_POINT ( 'NONE',  ( 0.7836604620899298990, -17.02735026737547841, 18.34798005863078885 ) ) ;
#25888=CARTESIAN_POINT ( 'NONE',  ( 16.86202325244926570, 2.345734461008496474, 18.80699882434806369 ) ) ;
#25890=CARTESIAN_POINT ( 'NONE',  ( -19.78695419347077333, 3.033347482080938740, 18.49267272388512140 ) ) ;
#25897=CARTESIAN_POINT ( 'NONE',  ( -4.940218127011004157, 16.29708528951388402, 18.55820869691756769 ) ) ;
#25899=CIRCLE ( 'NONE', #2011, 0.7500000000000003331 ) ;
#25904=CARTESIAN_POINT ( 'NONE',  ( -17.06249589246194276, 0.6902251470929409161, 6.341840715582230281 ) ) ;
#25906=CARTESIAN_POINT ( 'NONE',  ( 19.83281414115336005, 2.582324728781443923, 20.14992337338002670 ) ) ;
#25907=EDGE_LOOP ( 'NONE', ( #14645, #1678, #23168, #26379 ) ) ;
#25909=EDGE_CURVE ( 'NONE', #17261, #7591, #7583, .T. ) ;
#25912=ADVANCED_FACE ( 'NONE', ( #4020 ), #6204, .F. ) ;
#25913=CYLINDRICAL_SURFACE ( 'NONE', #9050, 0.7499999999999988898 ) ;
#25914=ORIENTED_EDGE ( 'NONE', *, *, #8874, .T. ) ;
#25917=CARTESIAN_POINT ( 'NONE',  ( -7.548823014270604759, 5.738360882150026931, 1.500000000000001332 ) ) ;
#25918=CARTESIAN_POINT ( 'NONE',  ( -18.45576848551221971, -7.706141034055812966, 6.518927109361836614 ) ) ;
#25923=LINE ( 'NONE', #26071, #26823 ) ;
#25929=CARTESIAN_POINT ( 'NONE',  ( -1.000000000000008438, 13.00000000000001421, 24.50000000000000000 ) ) ;
#25930=CARTESIAN_POINT ( 'NONE',  ( -17.64660589602035046, -9.450098986197517092, 19.79423548914561692 ) ) ;
#25940=LINE ( 'NONE', #14074, #17066 ) ;
#25941=ORIENTED_EDGE ( 'NONE', *, *, #8874, .F. ) ;
#25942=AXIS2_PLACEMENT_3D ( 'NONE', #27817, #15790, #3793 ) ;
#25944=AXIS2_PLACEMENT_3D ( 'NONE', #9166, #19140, #1843 ) ;
#25945=CARTESIAN_POINT ( 'NONE',  ( -13.54809176561740358, 10.35918576918405343, 7.652108011868851811 ) ) ;
#25946=DIRECTION ( 'NONE',  ( 0.000000000000000000, 0.000000000000000000, 1.000000000000000000 ) ) ;
#25947=CYLINDRICAL_SURFACE ( 'NONE', #6960, 9.482273699623480212 ) ;
#25951=DIRECTION ( 'NONE',  ( 0.000000000000000000, 0.000000000000000000, 1.000000000000000000 ) ) ;
#25954=CARTESIAN_POINT ( 'NONE',  ( 0.2355109517537158914, -20.01673911375432269, 20.34789198813115263 ) ) ;
#25956=CARTESIAN_POINT ( 'NONE',  ( -9.650234827617415689, -17.53789701089549879, 6.782048567692550378 ) ) ;
#25957=LINE ( 'NONE', #28143, #28299 ) ;
#25959=CARTESIAN_POINT ( 'NONE',  ( 1.219801289189190729, -17.01504883035040905, 20.25542030744407640 ) ) ;
#25960=ORIENTED_EDGE ( 'NONE', *, *, #1395, .T. ) ;
#25964=CARTESIAN_POINT ( 'NONE',  ( 1.367923798957378034, -19.95316478012377104, 19.48477075383299351 ) ) ;
#25969=CARTESIAN_POINT ( 'NONE',  ( -13.37849590498012553, 10.56201291617987792, 20.34789198813115263 ) ) ;
#25971=CARTESIAN_POINT ( 'NONE',  ( 3.094187858400090363, 16.79444423853913904, 19.08844262864049668 ) ) ;
#25973=PLANE ( 'NONE',  #21860 ) ;
#25975=EDGE_LOOP ( 'NONE', ( #21202, #28249 ) ) ;
#25976=ORIENTED_EDGE ( 'NONE', *, *, #22911, .F. ) ;
#25979=EDGE_CURVE ( 'NONE', #3526, #16618, #2276, .T. ) ;
#25980=DIRECTION ( 'NONE',  ( 0.5406408174555976665, -0.8412535328311810945, 0.000000000000000000 ) ) ;
#25982=AXIS2_PLACEMENT_3D ( 'NONE', #25858, #23354, #23496 ) ;
#25983=CARTESIAN_POINT ( 'NONE',  ( 11.93908819109399921, -16.04550321516295242, 19.21940439362674979 ) ) ;
#25984=ORIENTED_EDGE ( 'NONE', *, *, #6675, .F. ) ;
#25986=CARTESIAN_POINT ( 'NONE',  ( 15.81223571690235019, -6.365019318618784006, 20.34789198813115263 ) ) ;
#25988=CARTESIAN_POINT ( 'NONE',  ( 4.373786442354537840, 16.46525014965066092, 7.595116371587256054 ) ) ;
#25990=CARTESIAN_POINT ( 'NONE',  ( 6.225165711324287088, 19.02535939286849498, 19.66989035740801839 ) ) ;
#25992=CARTESIAN_POINT ( 'NONE',  ( 14.46722394715956561, 13.83532015011945937, 7.441806358946449151 ) ) ;
#25997=FACE_OUTER_BOUND ( 'NONE', #27961, .T. ) ;
#25998=EDGE_CURVE ( 'NONE', #1974, #4023, #8079, .T. ) ;
#26002=CARTESIAN_POINT ( 'NONE',  ( -15.49606647121365910, -7.052879176030718789, 7.272049892295485485 ) ) ;
#26003=CARTESIAN_POINT ( 'NONE',  ( 16.85582347140584858, 2.398957759809809076, 18.72771030977187579 ) ) ;
#26007=CARTESIAN_POINT ( 'NONE',  ( -0.5107318660475965721, -20.01137538934480986, 7.176035686813569292 ) ) ;
#26010=FACE_OUTER_BOUND ( 'NONE', #21247, .T. ) ;
#26015=CARTESIAN_POINT ( 'NONE',  ( -6.507434545313858898, 15.78991698230835361, 6.783738457429056012 ) ) ;
#26016=CARTESIAN_POINT ( 'NONE',  ( 0.000000000000000000, 0.000000000000000000, 21.50000000000000000 ) ) ;
#26024=FACE_OUTER_BOUND ( 'NONE', #2293, .T. ) ;
#26025=CARTESIAN_POINT ( 'NONE',  ( 19.59127448685153894, 4.109591991357616436, 18.92976555901915603 ) ) ;
#26027=VERTEX_POINT ( 'NONE', #21136 ) ;
#26028=DIRECTION ( 'NONE',  ( 1.000000000000000000, 0.000000000000000000, 0.000000000000000000 ) ) ;
#26031=ORIENTED_EDGE ( 'NONE', *, *, #10695, .T. ) ;
#26034=CARTESIAN_POINT ( 'NONE',  ( 1.068432182113367990, -19.98925970413798936, 7.366751648393900176 ) ) ;
#26042=CARTESIAN_POINT ( 'NONE',  ( -13.59008529392184883, 10.30512752726515124, 7.603368798681074736 ) ) ;
#26053=CARTESIAN_POINT ( 'NONE',  ( -5.485816626893764258, 19.23332246807784784, 7.526993102356320797 ) ) ;
#26055=CARTESIAN_POINT ( 'NONE',  ( -19.93127403599639891, 1.860458748833899278, 5.872146474157316831 ) ) ;
#26056=CARTESIAN_POINT ( 'NONE',  ( -0.4564504349075017564, 9.471281197126600659, 1.500000000000001332 ) ) ;
#26061=EDGE_LOOP ( 'NONE', ( #13263, #5648, #6093, #5151 ) ) ;
#26069=CARTESIAN_POINT ( 'NONE',  ( -18.30192086700450815, -8.065271870204650639, 7.454139397117723220 ) ) ;
#26071=CARTESIAN_POINT ( 'NONE',  ( -3.668292057955944596, 8.743977807160110416, 13.00000000000000178 ) ) ;
#26073=CARTESIAN_POINT ( 'NONE',  ( 15.55638214364780758, -6.928938690364088160, 7.453286057244487672 ) ) ;
#26074=AXIS2_PLACEMENT_3D ( 'NONE', #19097, #2723, #12231 ) ;
#26078=CARTESIAN_POINT ( 'NONE',  ( 8.840471615930072247, -1.687027447297460236, 1.500000000000001332 ) ) ;
#26079=AXIS2_PLACEMENT_3D ( 'NONE', #11061, #9032, #25558 ) ;
#26080=CARTESIAN_POINT ( 'NONE',  ( -14.81015662609899408, -8.488192507792284403, 19.97651184436794125 ) ) ;
#26082=AXIS2_PLACEMENT_3D ( 'NONE', #30162, #6466, #29704 ) ;
#26084=DIRECTION ( 'NONE',  ( -0.000000000000000000, -0.000000000000000000, 1.000000000000000000 ) ) ;
#26086=CARTESIAN_POINT ( 'NONE',  ( -0.6299556268942225756, -19.99014111075368305, 19.08232364404839743 ) ) ;
#26089=CARTESIAN_POINT ( 'NONE',  ( -6.813581335325352484, 18.80366338534912529, 6.149077423860700442 ) ) ;
#26090=ORIENTED_EDGE ( 'NONE', *, *, #13014, .F. ) ;
#26093=CARTESIAN_POINT ( 'NONE',  ( 5.687793815610356241, -6.974883619896809606, 1.500000000000001332 ) ) ;
#26101=CARTESIAN_POINT ( 'NONE',  ( 6.187077094091595342, 11.47693674426096599, 24.50000000000000000 ) ) ;
#26102=AXIS2_PLACEMENT_3D ( 'NONE', #20935, #2069, #16124 ) ;
#26104=CARTESIAN_POINT ( 'NONE',  ( 4.823417667949169818, 16.32807078418213464, 19.96344307082652492 ) ) ;
#26105=CARTESIAN_POINT ( 'NONE',  ( 1.365674945463512646, -19.97097327164668812, 19.36813350477385143 ) ) ;
#26106=ORIENTED_EDGE ( 'NONE', *, *, #2534, .T. ) ;
#26107=CARTESIAN_POINT ( 'NONE',  ( 18.64567588040446111, -7.235161915364464846, 6.037995405461180631 ) ) ;
#26109=CARTESIAN_POINT ( 'NONE',  ( 1.159631224985661513, -19.96657546246603943, 19.96797677718664232 ) ) ;
#26114=CARTESIAN_POINT ( 'NONE',  ( -17.73231296732452478, -9.288543855440103414, 5.951255046771932733 ) ) ;
#26119=LINE ( 'NONE', #23934, #12588 ) ;
#26120=EDGE_LOOP ( 'NONE', ( #20881, #3886, #809, #9029 ) ) ;
#26124=CARTESIAN_POINT ( 'NONE',  ( -13.37849590052435289, 10.56201291103764106, 7.652108011868850035 ) ) ;
#26127=CARTESIAN_POINT ( 'NONE',  ( 18.12620810650619418, -8.494884113463653463, 20.19668224736330941 ) ) ;
#26129=CARTESIAN_POINT ( 'NONE',  ( 5.008980049945720658, 16.26773947435521706, 6.530762810602277924 ) ) ;
#26130=B_SPLINE_CURVE_WITH_KNOTS ( 'NONE', 3,
 ( #24880, #20348, #8659, #3518, #10841, #3665, #8350, #15817, #10527, #5691, #25336, #13179, #8798, #15187, #22520, #6152 ),
 .UNSPECIFIED., .F., .F.,
 ( 4, 2, 2, 2, 2, 2, 2, 4 ),
 ( 0.4999999999999997780, 0.6249999999999996669, 0.6874999999999995559, 0.7187499999999995559, 0.7499999999999996669, 0.8124999999999996669, 0.8749999999999997780, 1.000000000000000000 ),
 .UNSPECIFIED. ) ;
#26132=ORIENTED_EDGE ( 'NONE', *, *, #2137, .T. ) ;
#26133=CARTESIAN_POINT ( 'NONE',  ( 6.270562923531076471, 19.01045013183040311, 19.45164628100866722 ) ) ;
#26135=LINE ( 'NONE', #1979, #26288 ) ;
#26137=ORIENTED_EDGE ( 'NONE', *, *, #2926, .T. ) ;
#26140=CARTESIAN_POINT ( 'NONE',  ( -8.413215745754975217, 3.196529495465474380, 1.500000000000001332 ) ) ;
#26142=CARTESIAN_POINT ( 'NONE',  ( -6.962021646281573162, -6.437683520590147701, 13.00000000000000178 ) ) ;
#26144=FACE_OUTER_BOUND ( 'NONE', #20730, .T. ) ;
#26145=EDGE_CURVE ( 'NONE', #5487, #13230, #29717, .T. ) ;
#26146=DIRECTION ( 'NONE',  ( -0.000000000000000000, -0.000000000000000000, -1.000000000000000000 ) ) ;
#26153=DIRECTION ( 'NONE',  ( 0.000000000000000000, 0.000000000000000000, -1.000000000000000000 ) ) ;
#26158=CARTESIAN_POINT ( 'NONE',  ( 10.61155637842188959, -13.37681800088531503, 19.79423548914561692 ) ) ;
#26160=VERTEX_POINT ( 'NONE', #12428 ) ;
#26162=EDGE_CURVE ( 'NONE', #15912, #12022, #29494, .T. ) ;
#26163=CARTESIAN_POINT ( 'NONE',  ( -15.51115086193518700, 12.62612245312785753, 7.626218077512942450 ) ) ;
#26164=EDGE_CURVE ( 'NONE', #863, #25840, #29569, .T. ) ;
#26167=CARTESIAN_POINT ( 'NONE',  ( 12.65169814564036521, 11.40562544919841237, 20.25336174263950184 ) ) ;
#26172=CARTESIAN_POINT ( 'NONE',  ( 16.73033351903584176, 3.274018421667484802, 18.34838970509067479 ) ) ;
#26174=ORIENTED_EDGE ( 'NONE', *, *, #25998, .F. ) ;
#26179=ORIENTED_EDGE ( 'NONE', *, *, #24067, .F. ) ;
#26181=EDGE_CURVE ( 'NONE', #26711, #10771, #3104, .T. ) ;
#26184=CARTESIAN_POINT ( 'NONE',  ( 1.771654956907825262, -16.98531529776322913, 6.892848776733236704 ) ) ;
#26186=CARTESIAN_POINT ( 'NONE',  ( -15.16307827826492449, -7.786259562520723598, 18.34798005863078885 ) ) ;
#26187=CARTESIAN_POINT ( 'NONE',  ( 1.788804076106752072, -16.98411955790561123, 19.21769074125273136 ) ) ;
#26188=CARTESIAN_POINT ( 'NONE',  ( 19.77852387640474419, 3.085824932809439591, 18.35377592296120497 ) ) ;
#26189=ORIENTED_EDGE ( 'NONE', *, *, #16466, .F. ) ;
#26190=CARTESIAN_POINT ( 'NONE',  ( -16.83148396119934276, 2.548526378087590416, 18.90679857307105749 ) ) ;
#26193=EDGE_LOOP ( 'NONE', ( #11423, #25984, #2216, #29971 ) ) ;
#26195=DIRECTION ( 'NONE',  ( -0.8412535328311804284, 0.5406408174555987767, 0.000000000000000000 ) ) ;
#26197=B_SPLINE_CURVE_WITH_KNOTS ( 'NONE', 3,
 ( #16465, #7251, #25830, #16764, #16159, #1814, #11335, #11488, #18655, #28160, #16314, #23469, #12411, #22214, #5229, #12563 ),
 .UNSPECIFIED., .F., .F.,
 ( 4, 2, 2, 2, 2, 2, 2, 4 ),
 ( 0.5000000000000000000, 0.6249999999999995559, 0.6874999999999997780, 0.7187500000000000000, 0.7500000000000002220, 0.8125000000000001110, 0.8750000000000000000, 1.000000000000000000 ),
 .UNSPECIFIED. ) ;
#26199=CARTESIAN_POINT ( 'NONE',  ( -5.941992259041529501, 19.11559255287554393, 18.34777357837151968 ) ) ;
#26203=CARTESIAN_POINT ( 'NONE',  ( -5.125804696664927995, 19.33206434738279356, 6.144783687052520094 ) ) ;
#26204=EDGE_LOOP ( 'NONE', ( #14593, #6689, #55, #22490 ) ) ;
#26209=CARTESIAN_POINT ( 'NONE',  ( 12.97958999564962568, 11.01328844340111068, 6.310736198168394928 ) ) ;
#26211=CARTESIAN_POINT ( 'NONE',  ( 18.35115018089978633, -7.996680568998187688, 7.652108011868850035 ) ) ;
#26213=VECTOR ( 'NONE', #15473, 1000.000000000000000 ) ;
#26218=CARTESIAN_POINT ( 'NONE',  ( 10.52757208845869208, -13.43854510672091074, 18.73314399819311760 ) ) ;
#26221=CIRCLE ( 'NONE', #16250, 0.7499999999999988898 ) ;
#26223=CARTESIAN_POINT ( 'NONE',  ( 10.58781394000596343, -16.96782583993082838, 20.14992337338002670 ) ) ;
#26224=ORIENTED_EDGE ( 'NONE', *, *, #13042, .F. ) ;
#26226=AXIS2_PLACEMENT_3D ( 'NONE', #11931, #17206, #7083 ) ;
#26230=CARTESIAN_POINT ( 'NONE',  ( -19.84344116185556217, 2.497567387674351824, 20.34789198813115263 ) ) ;
#26232=CARTESIAN_POINT ( 'NONE',  ( -17.73902742151047107, -9.275718677609281926, 20.06253562465620632 ) ) ;
#26236=VECTOR ( 'NONE', #13601, 1000.000000000000000 ) ;
#26238=EDGE_LOOP ( 'NONE', ( #24894, #8087, #18201, #7619 ) ) ;
#26243=VERTEX_POINT ( 'NONE', #20806 ) ;
#26245=CYLINDRICAL_SURFACE ( 'NONE', #19424, 9.482273699623480212 ) ;
#26246=ORIENTED_EDGE ( 'NONE', *, *, #8648, .T. ) ;
#26250=AXIS2_PLACEMENT_3D ( 'NONE', #17590, #27423, #29448 ) ;
#26251=VERTEX_POINT ( 'NONE', #11465 ) ;
#26253=CARTESIAN_POINT ( 'NONE',  ( 0.2321890030833208829, -17.02978461145532307, 20.19668224736330941 ) ) ;
#26262=CARTESIAN_POINT ( 'NONE',  ( 14.35775550668713585, 13.94852561378611711, 19.97651184436794125 ) ) ;
#26267=CIRCLE ( 'NONE', #12842, 0.7499999999999988898 ) ;
#26271=DIRECTION ( 'NONE',  ( 1.000000000000000000, 0.000000000000000000, 0.000000000000000000 ) ) ;
#26277=EDGE_LOOP ( 'NONE', ( #19941, #17195, #25756, #5458 ) ) ;
#26279=AXIS2_PLACEMENT_3D ( 'NONE', #14127, #1677, #8859 ) ;
#26286=CARTESIAN_POINT ( 'NONE',  ( 17.92217092160593950, -8.916983838002000340, 19.33715507985239412 ) ) ;
#26287=CARTESIAN_POINT ( 'NONE',  ( 4.917955972067796111, 16.29747060413738069, 6.211014596808754007 ) ) ;
#26288=VECTOR ( 'NONE', #14271, 1000.000000000000000 ) ;
#26290=CARTESIAN_POINT ( 'NONE',  ( 5.303645853345010153, 19.30241027580586177, 20.34789198813115263 ) ) ;
#26297=CARTESIAN_POINT ( 'NONE',  ( 15.75094665830062723, -12.32508334119354210, 1.500000000000001332 ) ) ;
#26298=ADVANCED_FACE ( 'NONE', ( #20946 ), #6158, .T. ) ;
#26299=EDGE_CURVE ( 'NONE', #5590, #16236, #13949, .T. ) ;
#26302=AXIS2_PLACEMENT_3D ( 'NONE', #30506, #13842, #23173 ) ;
#26308=CARTESIAN_POINT ( 'NONE',  ( 0.000000000000000000, 13.00000000000001421, 1.500000000000001332 ) ) ;
#26312=CARTESIAN_POINT ( 'NONE',  ( -19.96096598928918908, 1.505335854884785274, 19.14333282897057842 ) ) ;
#26315=( GEOMETRIC_REPRESENTATION_CONTEXT ( 3 ) GLOBAL_UNCERTAINTY_ASSIGNED_CONTEXT ( ( #1745 ) ) GLOBAL_UNIT_ASSIGNED_CONTEXT ( ( #891, #23970, #14468 ) ) REPRESENTATION_CONTEXT ( 'NONE', 'WORKASPACE' ) );
#26316=AXIS2_PLACEMENT_3D ( 'NONE', #23600, #30789, #16912 ) ;
#26317=DIRECTION ( 'NONE',  ( 0.000000000000000000, 0.000000000000000000, 1.000000000000000000 ) ) ;
#26325=EDGE_CURVE ( 'NONE', #3062, #24994, #23916, .T. ) ;
#26330=VERTEX_POINT ( 'NONE', #3024 ) ;
#26331=EDGE_CURVE ( 'NONE', #23022, #580, #12008, .T. ) ;
#26333=CARTESIAN_POINT ( 'NONE',  ( -15.84912786217080516, 12.19893545703369320, 19.96797677718664588 ) ) ;
#26335=ORIENTED_EDGE ( 'NONE', *, *, #28127, .T. ) ;
#26336=DIRECTION ( 'NONE',  ( -0.000000000000000000, 0.000000000000000000, -1.000000000000000000 ) ) ;
#26338=ORIENTED_EDGE ( 'NONE', *, *, #15125, .T. ) ;
#26341=CIRCLE ( 'NONE', #2931, 0.7500000000000006661 ) ;
#26342=VECTOR ( 'NONE', #13532, 1000.000000000000114 ) ;
#26346=CARTESIAN_POINT ( 'NONE',  ( -15.28186893989758310, 12.93018916568089338, 20.34789198813115263 ) ) ;
#26347=AXIS2_PLACEMENT_3D ( 'NONE', #5881, #8545, #17581 ) ;
#26349=CARTESIAN_POINT ( 'NONE',  ( -10.32985675426556327, -17.14655349859505051, 18.37415474056476938 ) ) ;
#26351=DIRECTION ( 'NONE',  ( 1.000000000000000000, 2.081668171172166620E-14, 0.000000000000000000 ) ) ;
#26352=CYLINDRICAL_SURFACE ( 'NONE', #13835, 0.7499999999999997780 ) ;
#26357=DIRECTION ( 'NONE',  ( 0.2817325568414296710, -0.9594929736144973687, 0.000000000000000000 ) ) ;
#26362=DIRECTION ( 'NONE',  ( -0.000000000000000000, -0.000000000000000000, 1.000000000000000000 ) ) ;
#26363=CARTESIAN_POINT ( 'NONE',  ( 18.64567588040448598, -7.235161915364460405, 18.73377938172350099 ) ) ;
#26368=CARTESIAN_POINT ( 'NONE',  ( -5.027435569059562681, 19.35787894679208065, 6.386539667786100161 ) ) ;
#26369=EDGE_LOOP ( 'NONE', ( #668, #6531, #13337, #24798 ) ) ;
#26371=CARTESIAN_POINT ( 'NONE',  ( 0.000000000000000000, 0.000000000000000000, 1.500000000000001332 ) ) ;
#26375=CARTESIAN_POINT ( 'NONE',  ( -1.687027447297492211, -8.840471615930066918, 21.50000000000000000 ) ) ;
#26377=CARTESIAN_POINT ( 'NONE',  ( 12.83215063165195424, 11.19227874472585960, 7.359006845440219102 ) ) ;
#26378=EDGE_CURVE ( 'NONE', #3771, #13976, #3037, .T. ) ;
#26379=ORIENTED_EDGE ( 'NONE', *, *, #22737, .T. ) ;
#26380=CARTESIAN_POINT ( 'NONE',  ( 18.71580048965418186, -7.100988023106707736, 6.341840715582230281 ) ) ;
#26382=DIRECTION ( 'NONE',  ( -0.000000000000000000, -0.000000000000000000, -1.000000000000000000 ) ) ;
#26383=CIRCLE ( 'NONE', #12943, 0.7500000000000006661 ) ;
#26384=DIRECTION ( 'NONE',  ( 1.000000000000000000, 0.000000000000000000, 0.000000000000000000 ) ) ;
#26389=DIRECTION ( 'NONE',  ( 0.000000000000000000, 0.000000000000000000, 1.000000000000000000 ) ) ;
#26398=VERTEX_POINT ( 'NONE', #24682 ) ;
#26401=CARTESIAN_POINT ( 'NONE',  ( 12.72536390617885438, -2.839914339433650348, 1.500000000000001332 ) ) ;
#26404=ADVANCED_FACE ( 'NONE', ( #26581 ), #14708, .T. ) ;
#26408=DIRECTION ( 'NONE',  ( 0.000000000000000000, 0.000000000000000000, 1.000000000000000000 ) ) ;
#26410=CARTESIAN_POINT ( 'NONE',  ( 19.56124041029250549, 4.166605025611198165, 6.919864475265779191 ) ) ;
#26415=VERTEX_POINT ( 'NONE', #13478 ) ;
#26417=CARTESIAN_POINT ( 'NONE',  ( -10.40347366321433675, -17.08171436691437961, 7.652108011868850923 ) ) ;
#26419=AXIS2_PLACEMENT_3D ( 'NONE', #17001, #11713, #2513 ) ;
#26422=CARTESIAN_POINT ( 'NONE',  ( -0.2365265214052963694, -17.01953242238517916, 19.33715507985239412 ) ) ;
#26423=CARTESIAN_POINT ( 'NONE',  ( -7.671865949551465391, -15.25812906914210565, 6.672349528511551497 ) ) ;
#26424=CARTESIAN_POINT ( 'NONE',  ( 8.840471615930072247, -1.687027447297460236, 1.500000000000001332 ) ) ;
#26425=CARTESIAN_POINT ( 'NONE',  ( 1.795183039316617268, -16.98367886218520795, 19.36813350477385143 ) ) ;
#26426=EDGE_LOOP ( 'NONE', ( #28822, #3622, #18231, #12964 ) ) ;
#26429=CARTESIAN_POINT ( 'NONE',  ( 11.91933518721469554, 12.21304923692660260, 18.56793045041961321 ) ) ;
#26431=ORIENTED_EDGE ( 'NONE', *, *, #16710, .T. ) ;
#26433=CARTESIAN_POINT ( 'NONE',  ( -14.71441417907129434, -8.667509008793196301, 6.892848776733236704 ) ) ;
#26434=CARTESIAN_POINT ( 'NONE',  ( -6.413028646417895828, 15.82458379172922314, 7.098451512883313441 ) ) ;
#26436=CARTESIAN_POINT ( 'NONE',  ( -18.28579658156515819, -8.145820804509366297, 18.49267272388512140 ) ) ;
#26437=AXIS2_PLACEMENT_3D ( 'NONE', #21803, #16666, #4655 ) ;
#26446=CARTESIAN_POINT ( 'NONE',  ( -14.68762770759668612, 13.60113105281362955, 6.755862304746362845 ) ) ;
#26450=CARTESIAN_POINT ( 'NONE',  ( 16.14824862690563378, -5.544579173785682435, 19.85459532544248162 ) ) ;
#26451=CARTESIAN_POINT ( 'NONE',  ( 1.000000000000008438, 13.00000000000001421, 1.500000000000001332 ) ) ;
#26453=CARTESIAN_POINT ( 'NONE',  ( 4.659914667891703388, 16.37914622779766916, 20.12545155307891065 ) ) ;
#26455=CARTESIAN_POINT ( 'NONE',  ( -7.700393225232525118, -15.24241778594406327, 19.08844262864050023 ) ) ;
#26457=VERTEX_POINT ( 'NONE', #16105 ) ;
#26458=DIRECTION ( 'NONE',  ( 1.000000000000000000, 0.000000000000000000, 0.000000000000000000 ) ) ;
#26459=VECTOR ( 'NONE', #208, 1000.000000000000000 ) ;
#26464=CARTESIAN_POINT ( 'NONE',  ( -15.55925901137642064, -6.904021205104067249, 6.974106381145714018 ) ) ;
#26465=CARTESIAN_POINT ( 'NONE',  ( 14.27394986618626582, 14.00917565527015896, 6.149077423860691560 ) ) ;
#26466=CARTESIAN_POINT ( 'NONE',  ( 0.2396382576306479717, -20.01636569787185138, 5.657991946698900598 ) ) ;
#26470=FACE_OUTER_BOUND ( 'NONE', #15517, .T. ) ;
#26479=SHAPE_REPRESENTATION_RELATIONSHIP ( 'NONE' , 'NONE' ,  #10497, #6874 ) ;
#26482=CARTESIAN_POINT ( 'NONE',  ( 7.869584159753955532, 10.39565510934977333, 1.500000000000001332 ) ) ;
#26485=CARTESIAN_POINT ( 'NONE',  ( 18.59495189863232412, -7.412450086248064451, 20.13759033520874908 ) ) ;
#26488=ORIENTED_EDGE ( 'NONE', *, *, #26648, .T. ) ;
#26494=FACE_OUTER_BOUND ( 'NONE', #7984, .T. ) ;
#26495=FACE_OUTER_BOUND ( 'NONE', #15210, .T. ) ;
#26499=LINE ( 'NONE', #24311, #18498 ) ;
#26502=ORIENTED_EDGE ( 'NONE', *, *, #15844, .F. ) ;
#26503=EDGE_CURVE ( 'NONE', #28158, #7938, #113, .T. ) ;
#26504=CARTESIAN_POINT ( 'NONE',  ( 10.30179067644846747, -17.16362715220463997, 6.974106381145714018 ) ) ;
#26507=ORIENTED_EDGE ( 'NONE', *, *, #30549, .T. ) ;
#26508=ORIENTED_EDGE ( 'NONE', *, *, #21750, .F. ) ;
#26513=ADVANCED_FACE ( 'NONE', ( #1906 ), #10813, .F. ) ;
#26515=CARTESIAN_POINT ( 'NONE',  ( 18.57491549710361767, -7.414944001931020878, 20.15039051365864609 ) ) ;
#26516=CARTESIAN_POINT ( 'NONE',  ( -15.27573937290510031, -7.547610621728815694, 5.676815824193227833 ) ) ;
#26517=CARTESIAN_POINT ( 'NONE',  ( -5.199332475351345906, 19.31257985896675677, 6.033082186765055255 ) ) ;
#26520=ORIENTED_EDGE ( 'NONE', *, *, #5959, .T. ) ;
#26527=CARTESIAN_POINT ( 'NONE',  ( 15.19061449783604623, 13.03728791304909329, 7.557577766377196582 ) ) ;
#26529=CARTESIAN_POINT ( 'NONE',  ( 15.87141697993283529, -6.228091237695526416, 7.643931100913408550 ) ) ;
#26530=CARTESIAN_POINT ( 'NONE',  ( 16.70031948171297387, 3.459335818475211877, 18.34938820207544907 ) ) ;
#26531=CARTESIAN_POINT ( 'NONE',  ( 1.000000000000008438, 16.48749217771910125, 24.50000000000000000 ) ) ;
#26540=FACE_OUTER_BOUND ( 'NONE', #24675, .T. ) ;
#26541=CARTESIAN_POINT ( 'NONE',  ( 10.83311381505435023, -16.83321666392360427, 20.29090034784956131 ) ) ;
#26542=CARTESIAN_POINT ( 'NONE',  ( 10.25394813640221336, -17.17138746996170795, 19.47728749465737863 ) ) ;
#26555=CARTESIAN_POINT ( 'NONE',  ( 3.196529495465388226, 8.413215745755008967, 21.50000000000000000 ) ) ;
#26563=FACE_OUTER_BOUND ( 'NONE', #16910, .T. ) ;
#26565=ORIENTED_EDGE ( 'NONE', *, *, #18571, .T. ) ;
#26566=CARTESIAN_POINT ( 'NONE',  ( 7.706848733600955015, 5.524309650260791571, 21.50000000000000000 ) ) ;
#26569=CARTESIAN_POINT ( 'NONE',  ( 14.87898868866547097, 13.36471831362574747, 5.652196082369964181 ) ) ;
#26575=VERTEX_POINT ( 'NONE', #14524 ) ;
#26577=CARTESIAN_POINT ( 'NONE',  ( -0.08122345276805303937, -17.02407875822364147, 19.87181966307587544 ) ) ;
#26581=FACE_OUTER_BOUND ( 'NONE', #13544, .T. ) ;
#26584=CARTESIAN_POINT ( 'NONE',  ( -8.499586724479453181, -2.959227181723774525, 1.500000000000001332 ) ) ;
#26586=ORIENTED_EDGE ( 'NONE', *, *, #1389, .T. ) ;
#26587=VECTOR ( 'NONE', #8578, 1000.000000000000000 ) ;
#26588=CYLINDRICAL_SURFACE ( 'NONE', #12387, 1.000000000000008438 ) ;
#26590=CARTESIAN_POINT ( 'NONE',  ( 14.34755844633281718, 13.95901041572539469, 18.73743063545763121 ) ) ;
#26592=FACE_OUTER_BOUND ( 'NONE', #23016, .T. ) ;
#26593=CARTESIAN_POINT ( 'NONE',  ( -14.83655028254229968, -8.438271213925730763, 5.951255046771932733 ) ) ;
#26594=CARTESIAN_POINT ( 'NONE',  ( -6.240920525956804354, 15.88642679632095955, 5.951255046771932733 ) ) ;
#26597=CARTESIAN_POINT ( 'NONE',  ( -4.163336342344337027E-14, 1.387778780781445676E-14, 24.50000000000000000 ) ) ;
#26598=CARTESIAN_POINT ( 'NONE',  ( -8.550548372801092256, -14.74545326687210611, 7.652108011868850923 ) ) ;
#26601=DIRECTION ( 'NONE',  ( 1.000000000000000000, 0.000000000000000000, 0.000000000000000000 ) ) ;
#26603=FACE_OUTER_BOUND ( 'NONE', #26277, .T. ) ;
#26611=CARTESIAN_POINT ( 'NONE',  ( 6.262709072525339593, 19.01302309856007966, 19.22654678686458141 ) ) ;
#26612=CIRCLE ( 'NONE', #13162, 0.7499999999999997780 ) ;
#26616=ORIENTED_EDGE ( 'NONE', *, *, #29545, .T. ) ;
#26622=CARTESIAN_POINT ( 'NONE',  ( -18.41515300997268056, -7.848447721146238010, 7.176035686813569292 ) ) ;
#26626=CARTESIAN_POINT ( 'NONE',  ( 6.778663211761462470, -6.630478080506934546, 21.50000000000000000 ) ) ;
#26630=CARTESIAN_POINT ( 'NONE',  ( 0.000000000000000000, 0.000000000000000000, 21.50000000000000000 ) ) ;
#26631=VERTEX_POINT ( 'NONE', #25917 ) ;
#26639=CARTESIAN_POINT ( 'NONE',  ( 15.42025756663164948, 12.76459690492384880, 19.96783386855779341 ) ) ;
#26640=CARTESIAN_POINT ( 'NONE',  ( -9.159129059799164807, -14.35414742152909717, 7.359006845440219102 ) ) ;
#26643=CARTESIAN_POINT ( 'NONE',  ( 19.74834695364560844, 3.274018421667484802, 18.34838970509067479 ) ) ;
#26645=ORIENTED_EDGE ( 'NONE', *, *, #8838, .T. ) ;
#26648=EDGE_CURVE ( 'NONE', #2787, #24319, #23528, .T. ) ;
#26651=CARTESIAN_POINT ( 'NONE',  ( -6.936828876846347747, 18.77725343618825349, 19.36813350477385143 ) ) ;
#26652=CARTESIAN_POINT ( 'NONE',  ( -14.68762770759668257, 13.60113105281362955, 19.45164628100866722 ) ) ;
#26654=CARTESIAN_POINT ( 'NONE',  ( -9.648244442396764597, -17.53899143774386715, 19.36813350477385143 ) ) ;
#26656=DIRECTION ( 'NONE',  ( 1.000000000000000000, 0.000000000000000000, 0.000000000000000000 ) ) ;
#26659=CARTESIAN_POINT ( 'NONE',  ( 9.582629137048309431, -14.08615220418401215, 5.701226463332907279 ) ) ;
#26661=CARTESIAN_POINT ( 'NONE',  ( 19.87925100141003654, 2.194397331962206987, 6.518927109361849936 ) ) ;
#26662=VERTEX_POINT ( 'NONE', #2205 ) ;
#26663=ORIENTED_EDGE ( 'NONE', *, *, #3856, .T. ) ;
#26665=CARTESIAN_POINT ( 'NONE',  ( 17.99898938545033289, -8.720395568141155351, 19.96302680909623817 ) ) ;
#26667=CYLINDRICAL_SURFACE ( 'NONE', #19835, 20.00000000000000000 ) ;
#26668=CARTESIAN_POINT ( 'NONE',  ( -15.37673962019508522, -7.325595981656019440, 5.774779864094946369 ) ) ;
#26669=FACE_OUTER_BOUND ( 'NONE', #3656, .T. ) ;
#26676=CARTESIAN_POINT ( 'NONE',  ( 14.87898868866547097, 13.36471831362575102, 18.34798005863227388 ) ) ;
#26678=CARTESIAN_POINT ( 'NONE',  ( 15.04974025769138990, 13.19961543621590572, 7.632642797338977658 ) ) ;
#26679=EDGE_LOOP ( 'NONE', ( #19768, #15248, #20680, #29795 ) ) ;
#26683=CARTESIAN_POINT ( 'NONE',  ( -18.58529988941444699, 7.388276390372320535, 24.50000000000000000 ) ) ;
#26684=ORIENTED_EDGE ( 'NONE', *, *, #19265, .T. ) ;
#26687=EDGE_CURVE ( 'NONE', #12864, #13348, #9321, .T. ) ;
#26692=CARTESIAN_POINT ( 'NONE',  ( 10.38931136226422147, -17.11076273665785763, 19.87181966307587544 ) ) ;
#26699=VERTEX_POINT ( 'NONE', #12663 ) ;
#26701=B_SPLINE_CURVE_WITH_KNOTS ( 'NONE', 3,
 ( #3423, #29477, #19792, #12947, #10596, #26665, #17618, #20110, #29625, #17467, #14961, #8261, #17767, #27286, #24473, #3257, #5918, #26989 ),
 .UNSPECIFIED., .F., .F.,
 ( 4, 2, 2, 2, 2, 2, 2, 2, 4 ),
 ( 0.003174295595554365527, 0.003570702171545611300, 0.003967108747536857508, 0.004363515323528103715, 0.004759921899519349055, 0.005156328475510595262, 0.005552735051501840602, 0.005949141627493086809, 0.006345548203484333016 ),
 .UNSPECIFIED. ) ;
#26705=CARTESIAN_POINT ( 'NONE',  ( -5.815855718377446415, -16.25752007041490188, -0.6213203435596476032 ) ) ;
#26707=FACE_OUTER_BOUND ( 'NONE', #3922, .T. ) ;
#26711=VERTEX_POINT ( 'NONE', #780 ) ;
#26712=AXIS2_PLACEMENT_3D ( 'NONE', #6541, #21163, #1701 ) ;
#26713=DIRECTION ( 'NONE',  ( -0.000000000000000000, -0.000000000000000000, -1.000000000000000000 ) ) ;
#26721=DIRECTION ( 'NONE',  ( -0.000000000000000000, -0.000000000000000000, -1.000000000000000000 ) ) ;
#26725=STYLED_ITEM('',(#30914),#2508);
#26730=CARTESIAN_POINT ( 'NONE',  ( -14.58213539500865785, 7.758783772730382111, -0.6213203435596476032 ) ) ;
#26733=CIRCLE ( 'NONE', #4301, 0.7500000000000006661 ) ;
#26734=LINE ( 'NONE', #21428, #10901 ) ;
#26736=CARTESIAN_POINT ( 'NONE',  ( 1.327349630778746237, -17.01025715289075890, 5.810767894563978686 ) ) ;
#26741=VECTOR ( 'NONE', #7529, 1000.000000000000114 ) ;
#26743=CARTESIAN_POINT ( 'NONE',  ( -14.72704883620386340, -8.644027383692558075, 6.341840715582230281 ) ) ;
#26747=CARTESIAN_POINT ( 'NONE',  ( -15.53738272950673327, -6.955830428693968059, 18.90679857307105749 ) ) ;
#26748=CARTESIAN_POINT ( 'NONE',  ( -4.102102735472397121, 8.549050687778208868, 21.50000000000000000 ) ) ;
#26750=EDGE_LOOP ( 'NONE', ( #13526, #12598, #19017, #19545 ) ) ;
#26751=EDGE_LOOP ( 'NONE', ( #3091, #22064, #26488, #7144 ) ) ;
#26752=DIRECTION ( 'NONE',  ( 1.000000000000000000, 0.000000000000000000, 0.000000000000000000 ) ) ;
#26754=CARTESIAN_POINT ( 'NONE',  ( -5.199332475351349458, 19.31257985896675322, 18.72886616302735163 ) ) ;
#26756=CARTESIAN_POINT ( 'NONE',  ( 0.5197766397933876181, -17.03069205084988980, 5.676815824193226057 ) ) ;
#26759=CARTESIAN_POINT ( 'NONE',  ( 18.35307960222155899, -7.992235168165439774, 18.34798005862930736 ) ) ;
#26760=CARTESIAN_POINT ( 'NONE',  ( -15.34618562042307843, 12.82554431217322310, 18.34798005863227388 ) ) ;
#26761=AXIS2_PLACEMENT_3D ( 'NONE', #22001, #9847, #19653 ) ;
#26763=ORIENTED_EDGE ( 'NONE', *, *, #17979, .T. ) ;
#26767=CARTESIAN_POINT ( 'NONE',  ( 9.249586724479433641, 2.959227181723830036, 21.50000000000000000 ) ) ;
#26773=CARTESIAN_POINT ( 'NONE',  ( 11.91798344328409875, -16.06126763266893320, 6.392525840300340434 ) ) ;
#26775=CIRCLE ( 'NONE', #28254, 0.7500000000000003331 ) ;
#26778=VECTOR ( 'NONE', #16377, 1000.000000000000000 ) ;
#26780=CARTESIAN_POINT ( 'NONE',  ( -18.10797733959154243, -8.533081443083743167, 5.657991946698900598 ) ) ;
#26781=FACE_BOUND ( 'NONE', #11405, .T. ) ;
#26785=VECTOR ( 'NONE', #9679, 1000.000000000000000 ) ;
#26788=DIRECTION ( 'NONE',  ( 0.000000000000000000, 0.000000000000000000, 1.000000000000000000 ) ) ;
#26794=LINE ( 'NONE', #14926, #13594 ) ;
#26798=VECTOR ( 'NONE', #8000, 1000.000000000000114 ) ;
#26803=ORIENTED_EDGE ( 'NONE', *, *, #332, .T. ) ;
#26805=CARTESIAN_POINT ( 'NONE',  ( 15.53792925084563059, 12.62098510012954655, 19.56050940960062690 ) ) ;
#26806=CARTESIAN_POINT ( 'NONE',  ( -10.58794734610131627, -16.98849370068515086, 5.653912893140659257 ) ) ;
#26807=ORIENTED_EDGE ( 'NONE', *, *, #6108, .T. ) ;
#26808=CARTESIAN_POINT ( 'NONE',  ( -16.95074943597165529, 1.765291926024247671, 7.652108011868850035 ) ) ;
#26818=B_SPLINE_CURVE_WITH_KNOTS ( 'NONE', 3,
 ( #12024, #23867, #19804, #2814, #17314, #619, #7348, #7186, #10137, #16697, #4841, #29165, #12337, #28872, #14357, #16859, #14512, #2511 ),
 .UNSPECIFIED., .F., .F.,
 ( 4, 2, 2, 2, 2, 2, 2, 2, 4 ),
 ( 0.000000000000000000, 0.0003967869494442872883, 0.0007935738988885745766, 0.001190360848332861973, 0.001587147797777149153, 0.001983934747221436333, 0.002380721696665723947, 0.002777508646110011126, 0.003174295595554298306 ),
 .UNSPECIFIED. ) ;
#26820=CARTESIAN_POINT ( 'NONE',  ( -6.509484584620661707, 15.78915919539661594, 19.25672174529527325 ) ) ;
#26821=CARTESIAN_POINT ( 'NONE',  ( -13.23068377149358987, 10.73719040084102794, 20.32842677360128292 ) ) ;
#26823=VECTOR ( 'NONE', #4706, 1000.000000000000000 ) ;
#26827=CYLINDRICAL_SURFACE ( 'NONE', #916, 20.00000000000000355 ) ;
#26828=EDGE_LOOP ( 'NONE', ( #21320, #4050, #7513, #2696 ) ) ;
#26829=CARTESIAN_POINT ( 'NONE',  ( 10.58525311124732227, -16.99040216561238381, 5.862424720655265098 ) ) ;
#26832=ORIENTED_EDGE ( 'NONE', *, *, #24326, .T. ) ;
#26835=CARTESIAN_POINT ( 'NONE',  ( 10.36341371996392091, -17.10561997787537436, 7.156831654632823003 ) ) ;
#26836=CARTESIAN_POINT ( 'NONE',  ( 7.827050521741880651, -5.352643706120488787, 1.500000000000001332 ) ) ;
#26837=CARTESIAN_POINT ( 'NONE',  ( -15.42263072605321916, -7.221902784610292336, 5.848946451764563292 ) ) ;
#26841=DIRECTION ( 'NONE',  ( 0.000000000000000000, 0.000000000000000000, -1.000000000000000000 ) ) ;
#26844=CIRCLE ( 'NONE', #17873, 0.7499999999999997780 ) ;
#26847=CARTESIAN_POINT ( 'NONE',  ( 19.87340826026480656, 2.401441585233818010, 7.272049892295485485 ) ) ;
#26849=CARTESIAN_POINT ( 'NONE',  ( 12.58124959699792988, 11.48680237977196406, 7.595116371587256054 ) ) ;
#26851=CARTESIAN_POINT ( 'NONE',  ( 16.19545619402288494, -5.420160174983561951, 6.560937769032974209 ) ) ;
#26857=DIRECTION ( 'NONE',  ( 0.5406408174555976665, -0.8412535328311810945, -0.000000000000000000 ) ) ;
#26860=CARTESIAN_POINT ( 'NONE',  ( -9.406652940105976413, 1.195154792889490114, 1.500000000000001332 ) ) ;
#26863=CARTESIAN_POINT ( 'NONE',  ( -8.840471615930058036, 1.687027447297517080, 1.500000000000001332 ) ) ;
#26864=ORIENTED_EDGE ( 'NONE', *, *, #25207, .T. ) ;
#26867=CARTESIAN_POINT ( 'NONE',  ( -13.99683207193583812, 9.784088562599670524, 19.58863275299554019 ) ) ;
#26868=CARTESIAN_POINT ( 'NONE',  ( -7.856594496258223259, -4.390207617113929039, 1.500000000000001332 ) ) ;
#26877=EDGE_CURVE ( 'NONE', #29287, #194, #29178, .T. ) ;
#26878=CYLINDRICAL_SURFACE ( 'NONE', #15513, 20.00000000000000000 ) ;
#26880=CIRCLE ( 'NONE', #5454, 0.7500000000000006661 ) ;
#26893=CARTESIAN_POINT ( 'NONE',  ( 0.000000000000000000, 0.000000000000000000, 1.500000000000001332 ) ) ;
#26898=DIRECTION ( 'NONE',  ( 0.000000000000000000, 0.000000000000000000, 1.000000000000000000 ) ) ;
#26902=CARTESIAN_POINT ( 'NONE',  ( -11.19942626343432046, -16.59192963269641652, 19.96783386855779341 ) ) ;
#26904=CARTESIAN_POINT ( 'NONE',  ( -1.000000000000008438, 19.97498435543819539, 1.500000000000001332 ) ) ;
#26905=CARTESIAN_POINT ( 'NONE',  ( 10.69045173577874053, -13.31838649416133791, 6.782048567692550378 ) ) ;
#26906=EDGE_CURVE ( 'NONE', #10785, #26575, #10619, .T. ) ;
#26913=CARTESIAN_POINT ( 'NONE',  ( -5.026174198947129135, 19.35820631361447397, 19.60917204426170102 ) ) ;
#26916=DIRECTION ( 'NONE',  ( -0.9594929736144974797, -0.2817325568414297265, 0.000000000000000000 ) ) ;
#26920=CARTESIAN_POINT ( 'NONE',  ( 15.78348099220816536, -6.430800111306882449, 18.34969686940296185 ) ) ;
#26922=EDGE_CURVE ( 'NONE', #1974, #27180, #17956, .T. ) ;
#26924=LINE ( 'NONE', #24558, #3326 ) ;
#26930=CARTESIAN_POINT ( 'NONE',  ( 11.77028954461706789, -16.17000817291663495, 7.272192800924339728 ) ) ;
#26931=EDGE_CURVE ( 'NONE', #28210, #1255, #14071, .T. ) ;
#26933=CARTESIAN_POINT ( 'NONE',  ( -19.75697076387333340, 3.109827004491391378, 20.14992337338002315 ) ) ;
#26934=ORIENTED_EDGE ( 'NONE', *, *, #1930, .F. ) ;
#26938=CARTESIAN_POINT ( 'NONE',  ( 16.18315216712290550, -5.452792103153281111, 6.392658652357117610 ) ) ;
#26940=AXIS2_PLACEMENT_3D ( 'NONE', #24450, #6653, #15869 ) ;
#26959=EDGE_CURVE ( 'NONE', #3771, #23438, #26612, .T. ) ;
#26961=CARTESIAN_POINT ( 'NONE',  ( 15.84193441942127833, -6.296838616230740371, 20.34789198813115263 ) ) ;
#26966=CARTESIAN_POINT ( 'NONE',  ( 0.000000000000000000, 0.000000000000000000, 1.500000000000001332 ) ) ;
#26968=DIRECTION ( 'NONE',  ( 0.4154150130018864906, -0.9096319953545183301, 0.000000000000000000 ) ) ;
#26970=ORIENTED_EDGE ( 'NONE', *, *, #22710, .F. ) ;
#26971=CARTESIAN_POINT ( 'NONE',  ( -7.322557715923444732, 14.41080185948837311, 24.50000000000000000 ) ) ;
#26972=EDGE_CURVE ( 'NONE', #14561, #27449, #25040, .T. ) ;
#26974=CARTESIAN_POINT ( 'NONE',  ( 16.56580381663018642, 4.144794415032111878, 6.341840715582230281 ) ) ;
#26976=EDGE_CURVE ( 'NONE', #8129, #9428, #9169, .T. ) ;
#26977=CARTESIAN_POINT ( 'NONE',  ( -10.39297074171570401, -17.10854403003572699, 18.35718225375110180 ) ) ;
#26979=DIRECTION ( 'NONE',  ( -1.000000000000000000, 0.000000000000000000, 0.000000000000000000 ) ) ;
#26982=CARTESIAN_POINT ( 'NONE',  ( 9.411519254647288335, -14.19511874370441262, 5.796888747622817029 ) ) ;
#26985=CARTESIAN_POINT ( 'NONE',  ( 6.812559277181973627, -5.881244434206257310, 1.500000000000001332 ) ) ;
#26989=CARTESIAN_POINT ( 'NONE',  ( 18.33793066653144876, -7.982499537706464920, 18.34798005863226678 ) ) ;
#26991=FACE_OUTER_BOUND ( 'NONE', #3611, .T. ) ;
#26995=CARTESIAN_POINT ( 'NONE',  ( -13.38160118231794549, 10.55829203257430038, 5.652196082368482699 ) ) ;
#26997=VECTOR ( 'NONE', #21467, 1000.000000000000000 ) ;
#26998=CARTESIAN_POINT ( 'NONE',  ( 3.668292057956000551, -8.743977807160085547, 13.00000000000000178 ) ) ;
#26999=CARTESIAN_POINT ( 'NONE',  ( 14.52517991353746751, 13.77415465259964478, 5.810767894563978686 ) ) ;
#27000=CARTESIAN_POINT ( 'NONE',  ( 16.87696675355430642, 2.215034284604906922, 6.420335371522007506 ) ) ;
#27003=VERTEX_POINT ( 'NONE', #27774 ) ;
#27005=PRODUCT_DEFINITION_CONTEXT ( 'detailed design', #14576, 'design' ) ;
#27011=DIRECTION ( 'NONE',  ( 0.000000000000000000, 0.000000000000000000, 1.000000000000000000 ) ) ;
#27014=DIRECTION ( 'NONE',  ( -0.000000000000000000, -0.000000000000000000, 1.000000000000000000 ) ) ;
#27016=CIRCLE ( 'NONE', #13573, 1.000000000000009548 ) ;
#27018=CARTESIAN_POINT ( 'NONE',  ( -14.01239083805805485, 9.763392886517387126, 19.25672174529527325 ) ) ;
#27028=CARTESIAN_POINT ( 'NONE',  ( 19.55539447853113799, 4.193631725790827325, 6.788986777570706010 ) ) ;
#27032=LINE ( 'NONE', #5659, #22645 ) ;
#27034=VERTEX_POINT ( 'NONE', #134 ) ;
#27046=CARTESIAN_POINT ( 'NONE',  ( 5.738360882149947884, 7.548823014270664267, 13.00000000000000178 ) ) ;
#27050=CARTESIAN_POINT ( 'NONE',  ( -9.376411575904489482, -14.20642299464376990, 19.56050940960062690 ) ) ;
#27051=CARTESIAN_POINT ( 'NONE',  ( -17.91516185886247925, -8.931344358737685951, 7.603368798681074736 ) ) ;
#27052=CARTESIAN_POINT ( 'NONE',  ( -6.193882932557621679, 19.03538945389874115, 5.678370764302467677 ) ) ;
#27054=FACE_OUTER_BOUND ( 'NONE', #4146, .T. ) ;
#27057=CARTESIAN_POINT ( 'NONE',  ( 0.000000000000000000, 0.000000000000000000, 1.500000000000001332 ) ) ;
#27064=ORIENTED_EDGE ( 'NONE', *, *, #18066, .F. ) ;
#27065=CARTESIAN_POINT ( 'NONE',  ( 16.12178322346233728, -5.613588367413085756, 18.73314399819312115 ) ) ;
#27066=CARTESIAN_POINT ( 'NONE',  ( 5.335947603960573993, 19.29354331951100576, 5.651989602109218858 ) ) ;
#27067=ORIENTED_EDGE ( 'NONE', *, *, #29235, .F. ) ;
#27068=DIRECTION ( 'NONE',  ( 0.9594929736144992560, 0.2817325568414232317, 0.000000000000000000 ) ) ;
#27076=DIRECTION ( 'NONE',  ( 1.000000000000000000, 0.000000000000000000, 0.000000000000000000 ) ) ;
#27077=DIRECTION ( 'NONE',  ( 1.000000000000000000, 0.000000000000000000, 0.000000000000000000 ) ) ;
#27079=ORIENTED_EDGE ( 'NONE', *, *, #23292, .F. ) ;
#27080=CARTESIAN_POINT ( 'NONE',  ( -15.21221250122201596, -7.682808169219083716, 5.657991946698900598 ) ) ;
#27081=DIRECTION ( 'NONE',  ( 1.000000000000000000, 0.000000000000000000, 0.000000000000000000 ) ) ;
#27082=EDGE_CURVE ( 'NONE', #9760, #5348, #23216, .T. ) ;
#27089=DIRECTION ( 'NONE',  ( -0.000000000000000000, -0.000000000000000000, 1.000000000000000000 ) ) ;
#27091=DIRECTION ( 'NONE',  ( -0.000000000000000000, -0.000000000000000000, 1.000000000000000000 ) ) ;
#27094=ORIENTED_EDGE ( 'NONE', *, *, #11521, .F. ) ;
#27096=LINE ( 'NONE', #1050, #16937 ) ;
#27098=CARTESIAN_POINT ( 'NONE',  ( 11.40980092660686118, 6.310027164379057751, 1.500000000000001332 ) ) ;
#27100=CIRCLE ( 'NONE', #11085, 0.7499999999999988898 ) ;
#27102=CARTESIAN_POINT ( 'NONE',  ( 12.91703683527121171, 11.08965543756653283, 18.80699882434806369 ) ) ;
#27104=ORIENTED_EDGE ( 'NONE', *, *, #9932, .F. ) ;
#27105=CARTESIAN_POINT ( 'NONE',  ( 18.52307105101190032, -7.590397700845933571, 20.25542030744407640 ) ) ;
#27106=CARTESIAN_POINT ( 'NONE',  ( 17.99898938545032223, -8.720395568141150022, 7.267242832833938238 ) ) ;
#27107=LINE ( 'NONE', #19765, #24424 ) ;
#27109=CARTESIAN_POINT ( 'NONE',  ( -4.390207617113899730, 7.856594496258241023, 1.500000000000001332 ) ) ;
#27111=ORIENTED_EDGE ( 'NONE', *, *, #2848, .F. ) ;
#27120=CARTESIAN_POINT ( 'NONE',  ( 16.66826434373540877, 3.628879393376895024, 7.559636331181775581 ) ) ;
#27121=CARTESIAN_POINT ( 'NONE',  ( -13.09601454503479445, 10.89247868135537622, 18.44501272782439827 ) ) ;
#27126=DIRECTION ( 'NONE',  ( 0.000000000000000000, -0.000000000000000000, -1.000000000000000000 ) ) ;
#27128=ADVANCED_FACE ( 'NONE', ( #9654 ), #28213, .F. ) ;
#27129=CARTESIAN_POINT ( 'NONE',  ( 10.44969336715137587, -17.07413037334559647, 6.018569869498933578 ) ) ;
#27138=DIRECTION ( 'NONE',  ( 0.000000000000000000, 0.000000000000000000, -1.000000000000000000 ) ) ;
#27144=CARTESIAN_POINT ( 'NONE',  ( -10.07574916981068647, -17.27697906656895199, 18.47531940416305929 ) ) ;
#27146=CARTESIAN_POINT ( 'NONE',  ( 19.84003625978226282, 2.664153601443037367, 5.796888747622817029 ) ) ;
#27148=CARTESIAN_POINT ( 'NONE',  ( 14.89413762494257121, 13.37445394317134095, 5.652196082367002106 ) ) ;
#27151=DIRECTION ( 'NONE',  ( -0.000000000000000000, -0.000000000000000000, 1.000000000000000000 ) ) ;
#27157=CARTESIAN_POINT ( 'NONE',  ( 4.049916830765392106, 16.55712665160099206, 7.652108011868850035 ) ) ;
#27159=LINE ( 'NONE', #20442, #11354 ) ;
#27161=VECTOR ( 'NONE', #5813, 1000.000000000000000 ) ;
#27164=CARTESIAN_POINT ( 'NONE',  ( -4.608906612435655248, -7.730328572437724866, 1.500000000000001332 ) ) ;
#27167=CARTESIAN_POINT ( 'NONE',  ( -13.72472375636738562, 10.13620556525982508, 18.50655187082627862 ) ) ;
#27168=CARTESIAN_POINT ( 'NONE',  ( 0.000000000000000000, 0.000000000000000000, 1.500000000000001332 ) ) ;
#27172=DIRECTION ( 'NONE',  ( 0.000000000000000000, 0.000000000000000000, -1.000000000000000000 ) ) ;
#27173=CARTESIAN_POINT ( 'NONE',  ( 12.35846533491531041, 11.73919094685904696, 7.652108011868850923 ) ) ;
#27175=DIRECTION ( 'NONE',  ( -0.8412535328311884220, -0.5406408174555862312, 0.000000000000000000 ) ) ;
#27177=CARTESIAN_POINT ( 'NONE',  ( 16.83292851407377455, 2.581421006753988223, 7.453286057244488561 ) ) ;
#27179=B_SPLINE_CURVE_WITH_KNOTS ( 'NONE', 3,
 ( #29159, #16850, #2973, #7495, #14807, #21510, #19342, #29007, #10130, #28864, #612, #10282, #16692, #19181, #16993, #26837, #26668, #26516, #4993, #12489 ),
 .UNSPECIFIED., .F., .F.,
 ( 4, 2, 2, 2, 2, 2, 2, 2, 2, 4 ),
 ( 0.000000000000000000, 0.06250000000000045797, 0.1250000000000009159, 0.1875000000000013878, 0.2187500000000014155, 0.2500000000000014433, 0.3125000000000010547, 0.3750000000000007216, 0.4375000000000003331, 0.4999999999999999445 ),
 .UNSPECIFIED. ) ;
#27180=VERTEX_POINT ( 'NONE', #5126 ) ;
#27183=CARTESIAN_POINT ( 'NONE',  ( 2.352830851074115159, 9.185733585337917617, 13.00000000000000178 ) ) ;
#27184=DIRECTION ( 'NONE',  ( 1.000000000000000000, 0.000000000000000000, 0.000000000000000000 ) ) ;
#27187=EDGE_LOOP ( 'NONE', ( #4089, #22185 ) ) ;
#27188=DIRECTION ( 'NONE',  ( 0.000000000000000000, 0.000000000000000000, 1.000000000000000000 ) ) ;
#27191=LINE ( 'NONE', #3487, #24741 ) ;
#27195=CARTESIAN_POINT ( 'NONE',  ( -11.19315777850256488, -16.57474394094692016, 7.267242832833947119 ) ) ;
#27200=CARTESIAN_POINT ( 'NONE',  ( -14.88329716083761411, -8.348731837201613715, 7.441806358946449151 ) ) ;
#27201=LINE ( 'NONE', #5837, #22518 ) ;
#27203=CARTESIAN_POINT ( 'NONE',  ( 10.05214800432092837, -13.77402237313447131, 5.678370764302467677 ) ) ;
#27206=ORIENTED_EDGE ( 'NONE', *, *, #30147, .T. ) ;
#27210=CARTESIAN_POINT ( 'NONE',  ( -15.35797807371378987, 12.83915352957770573, 5.652196082367002106 ) ) ;
#27212=ORIENTED_EDGE ( 'NONE', *, *, #18739, .T. ) ;
#27217=CARTESIAN_POINT ( 'NONE',  ( -8.072557715923444732, 14.41080185948837311, 1.500000000000000000 ) ) ;
#27218=DIRECTION ( 'NONE',  ( 0.9594929736144992560, 0.2817325568414232317, 0.000000000000000000 ) ) ;
#27227=CARTESIAN_POINT ( 'NONE',  ( -19.77456323383488268, 2.996942905618072306, 18.47110296274025387 ) ) ;
#27228=VERTEX_POINT ( 'NONE', #24305 ) ;
#27236=CARTESIAN_POINT ( 'NONE',  ( -18.04155359371238987, -8.631455508453164782, 18.34798005863227388 ) ) ;
#27238=DIRECTION ( 'NONE',  ( -1.000000000000000000, 0.000000000000000000, 0.000000000000000000 ) ) ;
#27244=ORIENTED_EDGE ( 'NONE', *, *, #8081, .T. ) ;
#27245=VECTOR ( 'NONE', #19513, 1000.000000000000000 ) ;
#27247=CARTESIAN_POINT ( 'NONE',  ( 15.75094665830062723, -12.32508334119354210, 24.50000000000000000 ) ) ;
#27250=ORIENTED_EDGE ( 'NONE', *, *, #6330, .T. ) ;
#27253=CARTESIAN_POINT ( 'NONE',  ( 15.55631266752686770, 12.59833113950373651, 19.33715507985239412 ) ) ;
#27255=ORIENTED_EDGE ( 'NONE', *, *, #12030, .T. ) ;
#27256=EDGE_CURVE ( 'NONE', #29319, #25416, #4974, .T. ) ;
#27257=CARTESIAN_POINT ( 'NONE',  ( 15.81223571690235019, -6.365019318618786670, 20.34789198813115263 ) ) ;
#27258=CARTESIAN_POINT ( 'NONE',  ( 19.66823596311670030, 3.724077645907920342, 20.19593175699879595 ) ) ;
#27260=DIRECTION ( 'NONE',  ( 0.000000000000000000, 0.000000000000000000, 1.000000000000000000 ) ) ;
#27263=CARTESIAN_POINT ( 'NONE',  ( -5.058868514795364923, 16.26385723645295656, 20.22273502201483453 ) ) ;
#27265=DIRECTION ( 'NONE',  ( -0.000000000000000000, -0.000000000000000000, 1.000000000000000000 ) ) ;
#27268=AXIS2_PLACEMENT_3D ( 'NONE', #22996, #8674, #25038 ) ;
#27271=CARTESIAN_POINT ( 'NONE',  ( 16.56823697822720476, 4.133291823432031720, 6.995624166085161910 ) ) ;
#27272=CARTESIAN_POINT ( 'NONE',  ( -12.86036580545043506, 11.15762522838069515, 18.71435384576123440 ) ) ;
#27274=CARTESIAN_POINT ( 'NONE',  ( -9.785592877189488448, -17.46290528139148179, 19.89182036555910571 ) ) ;
#27275=LINE ( 'NONE', #5908, #17520 ) ;
#27276=CARTESIAN_POINT ( 'NONE',  ( -19.90092023446657521, 2.162276205174162858, 18.39992786714538298 ) ) ;
#27282=LINE ( 'NONE', #3575, #21507 ) ;
#27286=CARTESIAN_POINT ( 'NONE',  ( 18.08129319977584615, -8.548428815984330242, 18.54479204710283469 ) ) ;
#27288=CARTESIAN_POINT ( 'NONE',  ( 11.00066062335189798, -16.70338693167701649, 5.651480102388687143 ) ) ;
#27290=DIRECTION ( 'NONE',  ( -0.000000000000000000, -0.000000000000000000, 1.000000000000000000 ) ) ;
#27293=VECTOR ( 'NONE', #11503, 1000.000000000000000 ) ;
#27294=CARTESIAN_POINT ( 'NONE',  ( 6.812559277181973627, -5.881244434206257310, 21.50000000000000000 ) ) ;
#27296=CARTESIAN_POINT ( 'NONE',  ( 6.140972302510982139, 19.03394436102034604, 7.156831654632813233 ) ) ;
#27297=ORIENTED_EDGE ( 'NONE', *, *, #8394, .F. ) ;
#27299=CARTESIAN_POINT ( 'NONE',  ( -9.658933677579518928, -17.51307076256854600, 19.08830981656262082 ) ) ;
#27300=CARTESIAN_POINT ( 'NONE',  ( 14.74216733233971510, 13.54174064842195691, 5.678370764302467677 ) ) ;
#27301=CARTESIAN_POINT ( 'NONE',  ( 16.85539258114951267, 2.401441585233818010, 7.272049892295485485 ) ) ;
#27302=ORIENTED_EDGE ( 'NONE', *, *, #13942, .F. ) ;
#27303=DIRECTION ( 'NONE',  ( -0.9096319953545185522, 0.4154150130018859355, 0.000000000000000000 ) ) ;
#27304=VERTEX_POINT ( 'NONE', #20694 ) ;
#27307=CARTESIAN_POINT ( 'NONE',  ( -13.99139173414502579, 9.791236547350349539, 19.08844262864049668 ) ) ;
#27311=AXIS2_PLACEMENT_3D ( 'NONE', #15241, #8713, #29933 ) ;
#27314=CARTESIAN_POINT ( 'NONE',  ( 3.835725748988833672, 16.61467071301744269, 7.627891251804737927 ) ) ;
#27316=CARTESIAN_POINT ( 'NONE',  ( 5.352643706120463918, 7.827050521741900191, 13.00000000000000178 ) ) ;
#27318=CARTESIAN_POINT ( 'NONE',  ( 0.3567158762617962386, -19.99681059701335073, 18.34798005863227388 ) ) ;
#27320=CARTESIAN_POINT ( 'NONE',  ( 19.84141769772507402, 2.653416696629038007, 20.19668224736330941 ) ) ;
#27322=B_SPLINE_CURVE_WITH_KNOTS ( 'NONE', 3,
 ( #537, #21596, #24089, #12717, #17229, #29401, #16926, #26913, #389, #15034, #5534, #19571, #26754, #5382, #12100, #14587, #14728, #24549 ),
 .UNSPECIFIED., .F., .F.,
 ( 4, 2, 2, 2, 2, 2, 2, 2, 4 ),
 ( 0.003174295595554313919, 0.003570702171545549284, 0.003967108747536784649, 0.004363515323528019581, 0.004759921899519254512, 0.005156328475510490311, 0.005552735051501725243, 0.005949141627492960174, 0.006345548203484195973 ),
 .UNSPECIFIED. ) ;
#27323=CARTESIAN_POINT ( 'NONE',  ( -16.82936799811532680, 2.561302842313196493, 19.77662771831109367 ) ) ;
#27324=CARTESIAN_POINT ( 'NONE',  ( 18.05043922081454610, -8.654756627348808351, 7.359006845440219102 ) ) ;
#27325=CARTESIAN_POINT ( 'NONE',  ( -13.98072106069838050, 9.805336070574282914, 19.03762469184452755 ) ) ;
#27326=CARTESIAN_POINT ( 'NONE',  ( -12.72536390617885260, -2.839914339433650348, 1.500000000000001332 ) ) ;
#27327=CARTESIAN_POINT ( 'NONE',  ( 5.296161872597630271, 19.28602264385380849, 20.34789198813115263 ) ) ;
#27330=ADVANCED_FACE ( 'NONE', ( #15562 ), #3407, .F. ) ;
#27331=CIRCLE ( 'NONE', #24304, 0.7500000000000006661 ) ;
#27332=DIRECTION ( 'NONE',  ( 1.000000000000000000, 0.000000000000000000, 0.000000000000000000 ) ) ;
#27333=ADVANCED_FACE ( 'NONE', ( #13238 ), #6369, .F. ) ;
#27334=B_SPLINE_SURFACE_WITH_KNOTS ( 'NONE', 3, 1, ( 
 ( #16039, #18076 ),
 ( #4032, #27596 ),
 ( #5913, #8255 ),
 ( #3418, #30230 ),
 ( #29621, #8877 ),
 ( #8419, #24936 ),
 ( #22436, #3573 ),
 ( #27748, #30080 ),
 ( #17762, #17931 ),
 ( #8715, #13558 ),
 ( #1079, #13095 ),
 ( #10592, #10743 ),
 ( #29780, #13250 ),
 ( #10910, #20412 ),
 ( #15724, #4331 ),
 ( #4495, #14004 ),
 ( #6821, #2290 ),
 ( #7288, #6671 ),
 ( #16348, #14292 ),
 ( #4643, #26158 ),
 ( #13858, #9320 ),
 ( #11812, #23502 ),
 ( #2460, #30390 ),
 ( #21317, #16186 ),
 ( #28660, #11371 ),
 ( #112, #14145 ),
 ( #23647, #25862 ),
 ( #9632, #21151 ),
 ( #7142, #23190 ),
 ( #4785, #16653 ),
 ( #30835, #20864 ) ),
 .UNSPECIFIED., .F., .F., .F.,
 ( 4, 3, 3, 3, 3, 3, 3, 3, 3, 3, 4 ),
 ( 2, 2 ),
 ( 0.4999999998345686092, 0.5360336730431939367, 0.5907651151589012883, 0.6456034593241830599, 0.6998270958050434309, 0.7529536536315937223, 0.8052385063053260073, 0.8575343587103997356, 0.9106564858195042023, 0.9648414833209685293, 1.000000006602610014 ),
 ( 0.000000000000000000, 1.000000000000000000 ),
 .UNSPECIFIED. ) ;
#27335=CARTESIAN_POINT ( 'NONE',  ( -5.279695238918637124, 19.30927203514151103, 20.05479082170252525 ) ) ;
#27336=CARTESIAN_POINT ( 'NONE',  ( 9.755064781586030520, 13.32952022457704544, 24.50000000000000000 ) ) ;
#27337=VECTOR ( 'NONE', #8207, 1000.000000000000000 ) ;
#27338=CARTESIAN_POINT ( 'NONE',  ( 3.662523238938590442, -12.47340865698848056, 1.500000000000001332 ) ) ;
#27340=EDGE_CURVE ( 'NONE', #1637, #20273, #15881, .T. ) ;
#27341=DIRECTION ( 'NONE',  ( 1.000000000000000000, 0.000000000000000000, 0.000000000000000000 ) ) ;
#27350=CARTESIAN_POINT ( 'NONE',  ( -19.80925230797850745, 2.758332870380174384, 7.626647697317573638 ) ) ;
#27354=CARTESIAN_POINT ( 'NONE',  ( 19.88570912806761370, 2.296683858978088466, 18.90679857307105749 ) ) ;
#27357=CARTESIAN_POINT ( 'NONE',  ( 9.131494062835614045, 2.555255504830995061, 21.50000000000000000 ) ) ;
#27358=CARTESIAN_POINT ( 'NONE',  ( -6.051176437752245008, 19.08139585423913331, 18.34838970509067479 ) ) ;
#27359=VECTOR ( 'NONE', #6181, 1000.000000000000000 ) ;
#27363=CARTESIAN_POINT ( 'NONE',  ( 0.4302108320067680181, -20.01327865860579536, 5.652605728828374865 ) ) ;
#27364=CARTESIAN_POINT ( 'NONE',  ( -16.83599852036188338, 2.522587596173209601, 6.143977687428010981 ) ) ;
#27369=CARTESIAN_POINT ( 'NONE',  ( -11.37681265597470137, -16.47072995046971755, 19.33715507985239412 ) ) ;
#27370=CARTESIAN_POINT ( 'NONE',  ( -15.01939917408025238, -8.081071717223313300, 7.603368798681074736 ) ) ;
#27372=CARTESIAN_POINT ( 'NONE',  ( 10.61155637842189314, -13.37681800088532569, 7.098451512883313441 ) ) ;
#27378=CARTESIAN_POINT ( 'NONE',  ( 9.864937699929956949, -13.90063973435163724, 18.34798005863078885 ) ) ;
#27380=CARTESIAN_POINT ( 'NONE',  ( -13.16299300229363567, 10.81582545713519927, 5.701226463332907279 ) ) ;
#27383=DIRECTION ( 'NONE',  ( 0.000000000000000000, 0.000000000000000000, -1.000000000000000000 ) ) ;
#27385=CARTESIAN_POINT ( 'NONE',  ( -9.011666854301585872, -14.45189732017202644, 7.500898271101006820 ) ) ;
#27388=CYLINDRICAL_SURFACE ( 'NONE', #13831, 20.00000000000000355 ) ;
#27396=CARTESIAN_POINT ( 'NONE',  ( -19.75724448635271102, 3.108068420208395910, 18.54479204710283824 ) ) ;
#27397=VERTEX_POINT ( 'NONE', #18530 ) ;
#27398=CARTESIAN_POINT ( 'NONE',  ( 2.555255504830960867, -9.131494062835622927, 13.00000000000000178 ) ) ;
#27402=CARTESIAN_POINT ( 'NONE',  ( -17.06629969734983376, 0.6399978984115163305, 6.783738457429056901 ) ) ;
#27410=CARTESIAN_POINT ( 'NONE',  ( -9.390093949354151093, -14.19700018541476005, 19.47784884541372463 ) ) ;
#27411=VERTEX_POINT ( 'NONE', #11362 ) ;
#27413=DIRECTION ( 'NONE',  ( -0.4154150130018973153, -0.9096319953545134451, 0.000000000000000000 ) ) ;
#27419=CARTESIAN_POINT ( 'NONE',  ( -5.800828033945498063, 16.03801949172214591, 18.34938820207544907 ) ) ;
#27423=DIRECTION ( 'NONE',  ( -0.000000000000000000, -0.000000000000000000, 1.000000000000000000 ) ) ;
#27424=CARTESIAN_POINT ( 'NONE',  ( 18.33599632111990019, -7.986941774664177096, 7.652108011868850035 ) ) ;
#27425=CARTESIAN_POINT ( 'NONE',  ( 14.87898868866547097, 13.36471831362574747, 5.652196082369964181 ) ) ;
#27428=FACE_OUTER_BOUND ( 'NONE', #17572, .T. ) ;
#27432=ORIENTED_EDGE ( 'NONE', *, *, #5385, .F. ) ;
#27433=CARTESIAN_POINT ( 'NONE',  ( 6.974883619896790954, 5.687793815610376669, 1.500000000000001332 ) ) ;
#27436=CARTESIAN_POINT ( 'NONE',  ( -8.487288213245033575, -14.78455279991285387, 20.34789198813115263 ) ) ;
#27438=CARTESIAN_POINT ( 'NONE',  ( -9.069887158786405834, -14.41355491436599046, 5.848946451764559740 ) ) ;
#27439=CARTESIAN_POINT ( 'NONE',  ( 9.169883732660084164, -9.268939115642975679, 24.50000000000000000 ) ) ;
#27440=EDGE_LOOP ( 'NONE', ( #12553, #2438, #22302, #19012 ) ) ;
#27441=DIRECTION ( 'NONE',  ( 0.2817325568414296710, -0.9594929736144973687, 0.000000000000000000 ) ) ;
#27443=LINE ( 'NONE', #6064, #10600 ) ;
#27447=DIRECTION ( 'NONE',  ( -0.000000000000000000, -0.000000000000000000, 1.000000000000000000 ) ) ;
#27448=CARTESIAN_POINT ( 'NONE',  ( -5.055631408663416870, 19.36903233965647786, 6.310736198168394928 ) ) ;
#27449=VERTEX_POINT ( 'NONE', #6811 ) ;
#27450=DIRECTION ( 'NONE',  ( 0.000000000000000000, 0.000000000000000000, 1.000000000000000000 ) ) ;
#27451=VECTOR ( 'NONE', #3090, 1000.000000000000000 ) ;
#27454=B_SPLINE_CURVE_WITH_KNOTS ( 'NONE', 3,
 ( #6373, #4173, #11050, #23187, #11365, #29773, #13245, #25084, #29931, #20858, #9023, #30225, #15407, #1540, #6057, #13090 ),
 .UNSPECIFIED., .F., .F.,
 ( 4, 2, 2, 2, 2, 2, 2, 4 ),
 ( 0.4999999999999999445, 0.6250000000000012212, 0.6875000000000018874, 0.7187500000000022204, 0.7500000000000026645, 0.8125000000000016653, 0.8750000000000006661, 1.000000000000000000 ),
 .UNSPECIFIED. ) ;
#27456=DIRECTION ( 'NONE',  ( 0.000000000000000000, 0.000000000000000000, 1.000000000000000000 ) ) ;
#27457=CARTESIAN_POINT ( 'NONE',  ( 11.65818676052303182, 12.48028922388247786, 6.560937769032974209 ) ) ;
#27458=CARTESIAN_POINT ( 'NONE',  ( 16.76146518920504391, 3.081792779576176589, 7.652108011868850035 ) ) ;
#27460=DIRECTION ( 'NONE',  ( 0.000000000000000000, 0.000000000000000000, 1.000000000000000000 ) ) ;
#27461=ORIENTED_EDGE ( 'NONE', *, *, #19665, .F. ) ;
#27462=CARTESIAN_POINT ( 'NONE',  ( -13.93204262645545377, 9.869472133065979591, 19.85459532544248518 ) ) ;
#27465=CARTESIAN_POINT ( 'NONE',  ( 4.537370253389202190, 19.49663512434673507, 7.280727868105637768 ) ) ;
#27466=CARTESIAN_POINT ( 'NONE',  ( 5.889883548616668740, 19.11329876149440565, 20.14992337338002670 ) ) ;
#27474=CARTESIAN_POINT ( 'NONE',  ( -19.70934530863873491, 3.501268498360766923, 19.45164628100866722 ) ) ;
#27475=CARTESIAN_POINT ( 'NONE',  ( 15.76678477342441731, -6.469363178373289891, 7.652108011868850035 ) ) ;
#27476=CARTESIAN_POINT ( 'NONE',  ( -15.35797660355606986, 12.83915183367558832, 18.34798005862662507 ) ) ;
#27477=CARTESIAN_POINT ( 'NONE',  ( 4.523123428450326777, 19.49994255397358600, 18.73743063545763121 ) ) ;
#27478=ORIENTED_EDGE ( 'NONE', *, *, #803, .T. ) ;
#27484=CARTESIAN_POINT ( 'NONE',  ( -4.850186825639134724, 16.32197540402032487, 20.05479082170252525 ) ) ;
#27486=FACE_OUTER_BOUND ( 'NONE', #1668, .T. ) ;
#27488=CARTESIAN_POINT ( 'NONE',  ( 4.390207617113956573, -7.856594496258208160, 21.50000000000000000 ) ) ;
#27490=CARTESIAN_POINT ( 'NONE',  ( 16.83255095306759586, 2.584307790288491891, 5.848946451764563292 ) ) ;
#27494=ORIENTED_EDGE ( 'NONE', *, *, #20023, .T. ) ;
#27500=LINE ( 'NONE', #6120, #29473 ) ;
#27502=CARTESIAN_POINT ( 'NONE',  ( 0.09286997694517430679, -20.00015982525766489, 5.676722608126684833 ) ) ;
#27505=EDGE_CURVE ( 'NONE', #4071, #13536, #16096, .T. ) ;
#27507=EDGE_CURVE ( 'NONE', #13582, #1637, #12627, .T. ) ;
#27513=EDGE_CURVE ( 'NONE', #29598, #18738, #21551, .T. ) ;
#27514=AXIS2_PLACEMENT_3D ( 'NONE', #18215, #25541, #18381 ) ;
#27515=CARTESIAN_POINT ( 'NONE',  ( -10.72135862580927146, -16.90494006806149940, 20.32842677360128292 ) ) ;
#27516=CARTESIAN_POINT ( 'NONE',  ( -14.92657760816262424, -8.264136099378397660, 7.500147780736496017 ) ) ;
#27518=CARTESIAN_POINT ( 'NONE',  ( -6.185259412586024297, 19.03819474808296874, 7.627891251804737927 ) ) ;
#27519=CARTESIAN_POINT ( 'NONE',  ( 10.62299781869221960, -13.36838230995977206, 6.233981582756856987 ) ) ;
#27524=ORIENTED_EDGE ( 'NONE', *, *, #24076, .T. ) ;
#27530=VERTEX_POINT ( 'NONE', #20015 ) ;
#27531=DIRECTION ( 'NONE',  ( 0.000000000000000000, 0.000000000000000000, 1.000000000000000000 ) ) ;
#27533=CARTESIAN_POINT ( 'NONE',  ( -9.223046300750478821, -14.31106556781055694, 7.272049892295485485 ) ) ;
#27535=ORIENTED_EDGE ( 'NONE', *, *, #19665, .T. ) ;
#27541=ADVANCED_FACE ( 'NONE', ( #5674 ), #14873, .F. ) ;
#27548=CARTESIAN_POINT ( 'NONE',  ( 16.19472973927114268, -5.422090571236383383, 6.588756557121048907 ) ) ;
#27551=CARTESIAN_POINT ( 'NONE',  ( -17.06630883447662583, 0.6398751886020394020, 6.588756557121049795 ) ) ;
#27554=DIRECTION ( 'NONE',  ( 0.000000000000000000, 0.000000000000000000, -1.000000000000000000 ) ) ;
#27564=CARTESIAN_POINT ( 'NONE',  ( -9.454746441592954298, 0.7220001660363460916, 21.50000000000000000 ) ) ;
#27567=EDGE_CURVE ( 'NONE', #30087, #2787, #8331, .T. ) ;
#27570=AXIS2_PLACEMENT_3D ( 'NONE', #17471, #3263, #12791 ) ;
#27571=CARTESIAN_POINT ( 'NONE',  ( -10.73812863781238036, -16.87327681817511049, 20.32243167357988867 ) ) ;
#27573=CARTESIAN_POINT ( 'NONE',  ( 15.45664188325221744, 12.69231265181876367, 7.156831654632818562 ) ) ;
#27576=CARTESIAN_POINT ( 'NONE',  ( -5.423201225924849211, 16.15625638780175066, 18.34727598691067740 ) ) ;
#27578=ORIENTED_EDGE ( 'NONE', *, *, #19867, .F. ) ;
#27579=CARTESIAN_POINT ( 'NONE',  ( -14.72786953156476386, -8.642539778695532249, 6.329955581934036069 ) ) ;
#27580=CARTESIAN_POINT ( 'NONE',  ( -16.81375614428661791, 2.649924382790542765, 19.21496526180054332 ) ) ;
#27582=CARTESIAN_POINT ( 'NONE',  ( -6.458857079296002723, 18.92875833827540788, 18.47531940416306284 ) ) ;
#27584=B_SPLINE_SURFACE_WITH_KNOTS ( 'NONE', 3, 1, ( 
 ( #13010, #20167 ),
 ( #27363, #17527 ),
 ( #29688, #24688 ),
 ( #17679, #3330 ),
 ( #8332, #998 ),
 ( #17846, #7716 ),
 ( #17213, #26736 ),
 ( #14874, #24386 ),
 ( #1470, #13633 ),
 ( #19021, #27658 ),
 ( #29828, #18301 ),
 ( #11847, #9501 ),
 ( #27822, #28531 ),
 ( #3798, #16518 ),
 ( #25153, #13483 ),
 ( #14329, #28384 ),
 ( #3963, #8947 ),
 ( #23111, #26184 ),
 ( #10981, #15796 ),
 ( #1619, #20480 ),
 ( #21344, #22964 ),
 ( #15641, #7008 ),
 ( #26034, #2319 ),
 ( #7165, #1758 ),
 ( #30000, #16676 ),
 ( #4816, #23841 ),
 ( #11274, #20771 ),
 ( #8638, #20627 ),
 ( #13320, #30299 ),
 ( #18870, #4667 ),
 ( #14169, #18149 ) ),
 .UNSPECIFIED., .F., .F., .F.,
 ( 4, 3, 3, 3, 3, 3, 3, 3, 3, 3, 4 ),
 ( 2, 2 ),
 ( 0.4999999998345682761, 0.5360336730431942698, 0.5907651151589017324, 0.6456034593241839481, 0.6998270958050443191, 0.7529536536315944995, 0.8052385063053264513, 0.8575343587103996246, 0.9106564858195047574, 0.9648414833209688624, 1.000000006602610014 ),
 ( 0.000000000000000000, 1.000000000000000000 ),
 .UNSPECIFIED. ) ;
#27585=CARTESIAN_POINT ( 'NONE',  ( 19.58381725123993888, 4.144794415032111878, 6.341840715582230281 ) ) ;
#27586=CARTESIAN_POINT ( 'NONE',  ( -15.35797807371378987, 12.83915352957770750, 18.34798005862930736 ) ) ;
#27587=AXIS2_PLACEMENT_3D ( 'NONE', #11938, #24073, #21730 ) ;
#27588=CARTESIAN_POINT ( 'NONE',  ( 1.305293688651088413, -17.01213356653430964, 7.545655578832111132 ) ) ;
#27590=VECTOR ( 'NONE', #19031, 1000.000000000000000 ) ;
#27591=CARTESIAN_POINT ( 'NONE',  ( -19.88823125026085492, 2.273432466552574027, 18.37415474056476938 ) ) ;
#27592=CARTESIAN_POINT ( 'NONE',  ( 1.000000000000008438, 13.00000000000001421, 24.50000000000000000 ) ) ;
#27593=VERTEX_POINT ( 'NONE', #19869 ) ;
#27596=CARTESIAN_POINT ( 'NONE',  ( 9.928183626064978284, -13.85837025666176281, 18.34838970509067479 ) ) ;
#27598=ORIENTED_EDGE ( 'NONE', *, *, #27638, .T. ) ;
#27601=DIRECTION ( 'NONE',  ( -1.000000000000000000, 0.000000000000000000, 0.000000000000000000 ) ) ;
#27602=CARTESIAN_POINT ( 'NONE',  ( -5.869193111140222463, 19.13804834536701804, 5.657991946698900598 ) ) ;
#27607=VERTEX_POINT ( 'NONE', #17526 ) ;
#27608=CARTESIAN_POINT ( 'NONE',  ( -10.39781135303994830, -17.08517550777068195, 18.34869673959212122 ) ) ;
#27616=ORIENTED_EDGE ( 'NONE', *, *, #10327, .F. ) ;
#27617=ORIENTED_EDGE ( 'NONE', *, *, #30393, .F. ) ;
#27618=CARTESIAN_POINT ( 'NONE',  ( 4.414161002286807189, 19.52491365267160717, 7.098451512883313441 ) ) ;
#27623=CARTESIAN_POINT ( 'NONE',  ( 11.05488513857797450, -16.68841100269527544, 18.34969686940296185 ) ) ;
#27624=CARTESIAN_POINT ( 'NONE',  ( 16.87846183053956395, 2.201534687727671802, 19.22654678686458141 ) ) ;
#27626=CARTESIAN_POINT ( 'NONE',  ( -19.80066175015358709, 2.942692509523778366, 20.25336174263950184 ) ) ;
#27627=CARTESIAN_POINT ( 'NONE',  ( 18.30570112562006102, -8.101025642224000123, 7.652108011868850035 ) ) ;
#27628=CARTESIAN_POINT ( 'NONE',  ( -15.97838715008243682, 12.05808207567198487, 6.447548852708279377 ) ) ;
#27629=CARTESIAN_POINT ( 'NONE',  ( 3.613053539807236536, 16.67204840528143350, 18.44527579819791185 ) ) ;
#27631=ORIENTED_EDGE ( 'NONE', *, *, #26972, .F. ) ;
#27635=CARTESIAN_POINT ( 'NONE',  ( 15.21452331804151115, 12.98203751624683733, 18.47110296274025742 ) ) ;
#27636=CARTESIAN_POINT ( 'NONE',  ( 13.00948632770315960, 10.97642674697307896, 6.782064869129509788 ) ) ;
#27638=EDGE_CURVE ( 'NONE', #22510, #23120, #7627, .T. ) ;
#27643=CARTESIAN_POINT ( 'NONE',  ( 14.73074142449663881, 5.627958522269737252, -0.6213203435596476032 ) ) ;
#27647=CARTESIAN_POINT ( 'NONE',  ( -19.69223482763159083, 3.495123391383815559, 6.518927109361852601 ) ) ;
#27649=CYLINDRICAL_SURFACE ( 'NONE', #5550, 20.00000000000000355 ) ;
#27650=ORIENTED_EDGE ( 'NONE', *, *, #16635, .T. ) ;
#27652=AXIS2_PLACEMENT_3D ( 'NONE', #16731, #25946, #18776 ) ;
#27653=DIRECTION ( 'NONE',  ( 0.000000000000000000, 0.000000000000000000, 1.000000000000000000 ) ) ;
#27658=CARTESIAN_POINT ( 'NONE',  ( 1.583371619456037438, -16.99707458536920157, 6.041646659195333058 ) ) ;
#27663=CARTESIAN_POINT ( 'NONE',  ( -4.950721362152968652, 16.29421905978776053, 7.453286057244488561 ) ) ;
#27676=DIRECTION ( 'NONE',  ( 1.000000000000000000, 0.000000000000000000, 0.000000000000000000 ) ) ;
#27678=CARTESIAN_POINT ( 'NONE',  ( -11.32740345151499994, -16.50481001894685917, 6.310736198168394928 ) ) ;
#27692=CARTESIAN_POINT ( 'NONE',  ( 11.66432357650553087, 12.47412091822526392, 19.21769074125273136 ) ) ;
#27697=DIRECTION ( 'NONE',  ( 0.000000000000000000, 0.000000000000000000, -1.000000000000000000 ) ) ;
#27698=CIRCLE ( 'NONE', #1801, 9.482273699623480212 ) ;
#27699=CARTESIAN_POINT ( 'NONE',  ( -15.37836256580256311, -7.321964739906460018, 20.22273502201483453 ) ) ;
#27700=DIRECTION ( 'NONE',  ( 1.000000000000000000, 0.000000000000000000, 0.000000000000000000 ) ) ;
#27702=DIRECTION ( 'NONE',  ( 0.2817325568414296710, 0.9594929736144973687, 0.000000000000000000 ) ) ;
#27704=CARTESIAN_POINT ( 'NONE',  ( -9.353104432054360373, -14.22246372585392038, 19.66962785902261857 ) ) ;
#27705=AXIS2_PLACEMENT_3D ( 'NONE', #11015, #22399, #20369 ) ;
#27709=CARTESIAN_POINT ( 'NONE',  ( -4.340342926365017284, -8.430595340551244377, 1.500000000000001332 ) ) ;
#27713=ORIENTED_EDGE ( 'NONE', *, *, #17599, .T. ) ;
#27714=LINE ( 'NONE', #20220, #26342 ) ;
#27715=EDGE_CURVE ( 'NONE', #23890, #19511, #1618, .T. ) ;
#27718=ORIENTED_EDGE ( 'NONE', *, *, #12771, .T. ) ;
#27720=CARTESIAN_POINT ( 'NONE',  ( -11.19063532726251964, -16.57644352599301030, 18.72886616302735519 ) ) ;
#27721=CIRCLE ( 'NONE', #24718, 1.000000000000000888 ) ;
#27731=CARTESIAN_POINT ( 'NONE',  ( -15.17592917621934490, 13.02713289664471397, 5.676722608126686609 ) ) ;
#27733=EDGE_LOOP ( 'NONE', ( #16310, #13987, #28333, #28642 ) ) ;
#27735=CARTESIAN_POINT ( 'NONE',  ( 16.78403870106610185, 2.933703390186591875, 20.32222155561919053 ) ) ;
#27742=CARTESIAN_POINT ( 'NONE',  ( -9.369089179312702242, -14.21146650728334038, 6.910395520694542881 ) ) ;
#27743=FACE_OUTER_BOUND ( 'NONE', #7965, .T. ) ;
#27744=ORIENTED_EDGE ( 'NONE', *, *, #24444, .F. ) ;
#27745=EDGE_CURVE ( 'NONE', #11023, #24333, #26775, .T. ) ;
#27748=CARTESIAN_POINT ( 'NONE',  ( 11.64616783614241058, -16.28139325077859922, 18.56793045041961321 ) ) ;
#27749=CIRCLE ( 'NONE', #11312, 0.7500000000000006661 ) ;
#27751=VERTEX_POINT ( 'NONE', #11127 ) ;
#27752=ORIENTED_EDGE ( 'NONE', *, *, #5162, .T. ) ;
#27754=CARTESIAN_POINT ( 'NONE',  ( -15.43151021478632323, 12.72345061513106579, 5.652912763329820400 ) ) ;
#27758=DIRECTION ( 'NONE',  ( -0.000000000000000000, -0.000000000000000000, -1.000000000000000000 ) ) ;
#27759=CIRCLE ( 'NONE', #9304, 9.482273699623480212 ) ;
#27760=CARTESIAN_POINT ( 'NONE',  ( -12.74661400764364139, 11.28197093996912415, 6.973843882838226094 ) ) ;
#27769=DIRECTION ( 'NONE',  ( 0.000000000000000000, 0.000000000000000000, 1.000000000000000000 ) ) ;
#27772=EDGE_LOOP ( 'NONE', ( #17732, #18005, #3736, #29826 ) ) ;
#27773=CARTESIAN_POINT ( 'NONE',  ( 3.518760595952259873, 16.69517982287621649, 5.810767894563978686 ) ) ;
#27774=CARTESIAN_POINT ( 'NONE',  ( 7.869584159753955532, 10.39565510934977333, 24.50000000000000000 ) ) ;
#27775=DIRECTION ( 'NONE',  ( -0.000000000000000000, -0.000000000000000000, 1.000000000000000000 ) ) ;
#27780=CARTESIAN_POINT ( 'NONE',  ( 9.014152831625308337, -14.43863835250231098, 19.22654678686458141 ) ) ;
#27782=VERTEX_POINT ( 'NONE', #8498 ) ;
#27783=AXIS2_PLACEMENT_3D ( 'NONE', #5318, #5014, #29498 ) ;
#27785=CARTESIAN_POINT ( 'NONE',  ( 15.45343642833786646, -7.142940632752242891, 6.111214848085761986 ) ) ;
#27787=CARTESIAN_POINT ( 'NONE',  ( -13.95900029477594906, 9.834024558217738132, 6.233981582756856987 ) ) ;
#27788=CARTESIAN_POINT ( 'NONE',  ( 4.339153914952778912, 19.54170514621187138, 19.58863275299554019 ) ) ;
#27793=CARTESIAN_POINT ( 'NONE',  ( 12.35522425158189108, 11.74279415389956505, 5.652196082368482699 ) ) ;
#27796=CARTESIAN_POINT ( 'NONE',  ( -5.450136891332535427, 19.26184010647176237, 20.19668224736330941 ) ) ;
#27802=ORIENTED_EDGE ( 'NONE', *, *, #5575, .T. ) ;
#27804=CARTESIAN_POINT ( 'NONE',  ( 0.8643805006890358245, -19.98168094404550033, 5.779535427900761135 ) ) ;
#27808=CARTESIAN_POINT ( 'NONE',  ( 4.082218581380954170, 16.54825969530612895, 18.34777357837151612 ) ) ;
#27809=VERTEX_POINT ( 'NONE', #6129 ) ;
#27810=CARTESIAN_POINT ( 'NONE',  ( -6.437683520590121056, 6.962021646281599807, 1.500000000000001332 ) ) ;
#27817=CARTESIAN_POINT ( 'NONE',  ( 3.685570353517261477, -16.10136545388692397, -0.6213203435596476032 ) ) ;
#27822=CARTESIAN_POINT ( 'NONE',  ( 1.315538599303260447, -19.97434797600632805, 6.341840715582230281 ) ) ;
#27826=DIRECTION ( 'NONE',  ( -0.000000000000000000, -0.000000000000000000, 1.000000000000000000 ) ) ;
#27829=CARTESIAN_POINT ( 'NONE',  ( -15.16307466679258553, -7.786257835066843214, 18.34798005862662507 ) ) ;
#27832=CIRCLE ( 'NONE', #14366, 1.000000000000004441 ) ;
#27834=CARTESIAN_POINT ( 'NONE',  ( -0.6570508600772855257, -19.98920419113419200, 19.21471108562414898 ) ) ;
#27838=ORIENTED_EDGE ( 'NONE', *, *, #2199, .T. ) ;
#27841=CARTESIAN_POINT ( 'NONE',  ( -14.58213539500865785, 7.758783772730382111, -0.6213203435596476032 ) ) ;
#27845=AXIS2_PLACEMENT_3D ( 'NONE', #13056, #3840, #5713 ) ;
#27848=VERTEX_POINT ( 'NONE', #8946 ) ;
#27853=ORIENTED_EDGE ( 'NONE', *, *, #21958, .F. ) ;
#27854=CARTESIAN_POINT ( 'NONE',  ( -7.730328572437709767, 4.608906612435681005, 1.500000000000001332 ) ) ;
#27855=CARTESIAN_POINT ( 'NONE',  ( 16.58239702337846566, 4.066005520140572038, 7.158811349119580392 ) ) ;
#27858=EDGE_CURVE ( 'NONE', #11886, #16236, #1367, .T. ) ;
#27864=CARTESIAN_POINT ( 'NONE',  ( -18.37726663805288396, -7.892083924814675910, 19.96302680909624883 ) ) ;
#27865=EDGE_CURVE ( 'NONE', #357, #3146, #30593, .T. ) ;
#27866=CARTESIAN_POINT ( 'NONE',  ( -18.24831633358133942, -8.229495485092105156, 20.25336174263950184 ) ) ;
#27867=CARTESIAN_POINT ( 'NONE',  ( -8.975220329042040035, -14.47597657772637447, 18.47056384035244037 ) ) ;
#27875=ORIENTED_EDGE ( 'NONE', *, *, #12819, .T. ) ;
#27878=CARTESIAN_POINT ( 'NONE',  ( -4.163336342344337027E-14, 1.387778780781445676E-14, 24.50000000000000000 ) ) ;
#27883=CARTESIAN_POINT ( 'NONE',  ( -19.71887672257058810, 3.447422735172819497, 6.310736198168394928 ) ) ;
#27885=DIRECTION ( 'NONE',  ( 0.9898214418809327952, -0.1423148382732850048, 0.000000000000000000 ) ) ;
#27889=CARTESIAN_POINT ( 'NONE',  ( 0.7788148816922458861, -17.02744011591804707, 20.34789198813115263 ) ) ;
#27901=CARTESIAN_POINT ( 'NONE',  ( -8.661893131359024167, -14.67663382386235149, 7.652108011868851811 ) ) ;
#27902=CARTESIAN_POINT ( 'NONE',  ( -7.856594496258223259, -4.390207617113929039, 1.500000000000001332 ) ) ;
#27904=EDGE_CURVE ( 'NONE', #4157, #5507, #23418, .T. ) ;
#27907=ORIENTED_EDGE ( 'NONE', *, *, #6134, .F. ) ;
#27911=CARTESIAN_POINT ( 'NONE',  ( -4.594331223478845594, 16.38995132059639914, 6.420335371522007506 ) ) ;
#27912=ORIENTED_EDGE ( 'NONE', *, *, #19011, .F. ) ;
#27914=DIRECTION ( 'NONE',  ( -0.000000000000000000, -0.000000000000000000, 1.000000000000000000 ) ) ;
#27915=VERTEX_POINT ( 'NONE', #18751 ) ;
#27917=AXIS2_PLACEMENT_3D ( 'NONE', #9712, #17194, #29056 ) ;
#27919=ORIENTED_EDGE ( 'NONE', *, *, #24594, .T. ) ;
#27920=DIRECTION ( 'NONE',  ( 0.000000000000000000, 0.000000000000000000, 1.000000000000000000 ) ) ;
#27923=CYLINDRICAL_SURFACE ( 'NONE', #2965, 0.7500000000000006661 ) ;
#27929=CARTESIAN_POINT ( 'NONE',  ( 0.6479391101829744537, -17.02974303764626640, 20.34789198813115974 ) ) ;
#27931=DIRECTION ( 'NONE',  ( -0.000000000000000000, -0.000000000000000000, 1.000000000000000000 ) ) ;
#27932=CARTESIAN_POINT ( 'NONE',  ( 16.79425489945616334, 2.861376016183142745, 20.29090034784956131 ) ) ;
#27934=CARTESIAN_POINT ( 'NONE',  ( -16.81771903218351483, 2.627522578025004663, 19.56050940960062690 ) ) ;
#27937=CARTESIAN_POINT ( 'NONE',  ( -15.92677741484699006, 12.12620433921148688, 7.098451512883313441 ) ) ;
#27938=CARTESIAN_POINT ( 'NONE',  ( 5.151948548241253256, 19.34356600583523544, 18.35718225375110180 ) ) ;
#27941=DIRECTION ( 'NONE',  ( 0.000000000000000000, 0.000000000000000000, 1.000000000000000000 ) ) ;
#27943=CARTESIAN_POINT ( 'NONE',  ( 15.53731853391909112, 12.59332096006129831, 19.47728749465736442 ) ) ;
#27944=CARTESIAN_POINT ( 'NONE',  ( 13.01334791338954489, 10.97165762312714143, 6.519181285484535238 ) ) ;
#27946=CARTESIAN_POINT ( 'NONE',  ( 7.869584159753955532, 10.39565510934977333, 1.500000000000001332 ) ) ;
#27949=CARTESIAN_POINT ( 'NONE',  ( -1.195154792889456363, -9.406652940105981742, 21.50000000000000000 ) ) ;
#27951=CARTESIAN_POINT ( 'NONE',  ( -19.96096598928918908, 1.505335854884786828, 6.447548852708279377 ) ) ;
#27952=CARTESIAN_POINT ( 'NONE',  ( 14.87898868866547097, 13.36471831362575102, 18.34798005863227388 ) ) ;
#27953=CARTESIAN_POINT ( 'NONE',  ( 11.11118051879628155, -16.62953239715190534, 18.34798005863227388 ) ) ;
#27957=LINE ( 'NONE', #16, #23875 ) ;
#27960=CARTESIAN_POINT ( 'NONE',  ( -19.94482228061659512, 1.484609193405911132, 19.21940439362674624 ) ) ;
#27961=EDGE_LOOP ( 'NONE', ( #7929, #25495, #27212, #25023 ) ) ;
#27969=ORIENTED_EDGE ( 'NONE', *, *, #16569, .F. ) ;
#27970=DIRECTION ( 'NONE',  ( 1.000000000000000000, 0.000000000000000000, 0.000000000000000000 ) ) ;
#27971=CARTESIAN_POINT ( 'NONE',  ( 12.86767874445214055, -1.850092897552706894, 1.500000000000001332 ) ) ;
#27975=VECTOR ( 'NONE', #8680, 1000.000000000000000 ) ;
#27977=ORIENTED_EDGE ( 'NONE', *, *, #13249, .T. ) ;
#27978=FACE_BOUND ( 'NONE', #13, .T. ) ;
#27981=FACE_BOUND ( 'NONE', #7380, .T. ) ;
#27983=CARTESIAN_POINT ( 'NONE',  ( -13.97970881677065158, 9.806700574782176716, 6.329955581934036069 ) ) ;
#27989=ORIENTED_EDGE ( 'NONE', *, *, #1382, .T. ) ;
#27990=CARTESIAN_POINT ( 'NONE',  ( 11.32565050298867781, -16.48467196965851045, 7.626218077512944227 ) ) ;
#27991=CARTESIAN_POINT ( 'NONE',  ( -8.257638164125266300, -14.92340941578111746, 5.704143890883081269 ) ) ;
#27996=CARTESIAN_POINT ( 'NONE',  ( 0.000000000000000000, 0.000000000000000000, 1.500000000000001332 ) ) ;
#27997=DIRECTION ( 'NONE',  ( 0.1423148382732746797, -0.9898214418809342385, 0.000000000000000000 ) ) ;
#28006=CARTESIAN_POINT ( 'NONE',  ( -18.47348503376730022, -7.710222065540593306, 19.45164628100866722 ) ) ;
#28008=EDGE_LOOP ( 'NONE', ( #6503, #13959 ) ) ;
#28010=CARTESIAN_POINT ( 'NONE',  ( 9.131494062835614045, 2.555255504830995061, 13.00000000000000178 ) ) ;
#28012=CARTESIAN_POINT ( 'NONE',  ( 11.80555446153501897, -11.55276080277260320, -0.6213203435596476032 ) ) ;
#28014=CARTESIAN_POINT ( 'NONE',  ( 17.92455701194924700, -8.912206770388250376, 19.45164628100866722 ) ) ;
#28017=ORIENTED_EDGE ( 'NONE', *, *, #23066, .T. ) ;
#28018=CARTESIAN_POINT ( 'NONE',  ( -19.78695419347076623, 3.033347482080934299, 5.796888747622817029 ) ) ;
#28019=CYLINDRICAL_SURFACE ( 'NONE', #10329, 1.000000000000000888 ) ;
#28023=CARTESIAN_POINT ( 'NONE',  ( 5.291486201320592109, 19.28729773841935469, 18.34798005863227388 ) ) ;
#28025=AXIS2_PLACEMENT_3D ( 'NONE', #25435, #3920, #18255 ) ;
#28029=CYLINDRICAL_SURFACE ( 'NONE', #29273, 0.7499999999999997780 ) ;
#28031=CARTESIAN_POINT ( 'NONE',  ( 16.86493654369872175, 2.320966539700319853, 19.85270094495841775 ) ) ;
#28034=CARTESIAN_POINT ( 'NONE',  ( -0.6129396130214317395, -20.00853051056088816, 6.974106381145714018 ) ) ;
#28039=CARTESIAN_POINT ( 'NONE',  ( -19.96222469201676475, 1.488090962520938865, 19.25672174529527325 ) ) ;
#28040=DIRECTION ( 'NONE',  ( 1.000000000000000000, 0.000000000000000000, 0.000000000000000000 ) ) ;
#28041=EDGE_LOOP ( 'NONE', ( #8894, #28802, #25174, #7158 ) ) ;
#28043=ORIENTED_EDGE ( 'NONE', *, *, #836, .T. ) ;
#28048=LINE ( 'NONE', #20870, #15351 ) ;
#28053=DIRECTION ( 'NONE',  ( 1.000000000000000000, 0.000000000000000000, 0.000000000000000000 ) ) ;
#28054=VERTEX_POINT ( 'NONE', #19659 ) ;
#28060=DIRECTION ( 'NONE',  ( -0.000000000000000000, -0.000000000000000000, 1.000000000000000000 ) ) ;
#28063=FACE_OUTER_BOUND ( 'NONE', #19375, .T. ) ;
#28064=ADVANCED_FACE ( 'NONE', ( #20135 ), #1441, .T. ) ;
#28067=ADVANCED_FACE ( 'NONE', ( #4064 ), #13445, .F. ) ;
#28077=CARTESIAN_POINT ( 'NONE',  ( 16.74250592919979752, 3.198927888535952668, 18.34798005862930736 ) ) ;
#28079=CARTESIAN_POINT ( 'NONE',  ( 10.58066667298599661, -16.99307187112385620, 7.429667576816606278 ) ) ;
#28081=CARTESIAN_POINT ( 'NONE',  ( -15.45023549775890004, 12.72816703665372984, 20.33971507717571114 ) ) ;
#28082=CARTESIAN_POINT ( 'NONE',  ( 4.469338653509383974, 19.51245501789046344, 19.89182036555910571 ) ) ;
#28084=EDGE_LOOP ( 'NONE', ( #13411, #19316, #9876, #9698 ) ) ;
#28085=CARTESIAN_POINT ( 'NONE',  ( -18.04365185506138047, -8.627086862512674870, 7.652108011868850035 ) ) ;
#28089=CARTESIAN_POINT ( 'NONE',  ( -5.332709978455694610, 16.18357461815304532, 18.36582235739946611 ) ) ;
#28090=LINE ( 'NONE', #18888, #23062 ) ;
#28097=AXIS2_PLACEMENT_3D ( 'NONE', #25116, #16065, #1713 ) ;
#28100=CARTESIAN_POINT ( 'NONE',  ( 0.9714284548196548963, -19.97661650614235995, 7.454606537396340826 ) ) ;
#28110=CARTESIAN_POINT ( 'NONE',  ( 0.3567147238643512130, -19.99681861211370659, 5.652196082369963293 ) ) ;
#28115=CARTESIAN_POINT ( 'NONE',  ( -5.686690470302443678, 16.07334902597871462, 20.33971507717571114 ) ) ;
#28116=VECTOR ( 'NONE', #10567, 1000.000000000000000 ) ;
#28124=CARTESIAN_POINT ( 'NONE',  ( -14.92167319134950176, -8.273715889511853661, 18.50655187082627862 ) ) ;
#28127=EDGE_CURVE ( 'NONE', #16284, #19910, #3362, .T. ) ;
#28129=ORIENTED_EDGE ( 'NONE', *, *, #29040, .F. ) ;
#28130=FACE_OUTER_BOUND ( 'NONE', #12382, .T. ) ;
#28133=CARTESIAN_POINT ( 'NONE',  ( -4.163336342344337027E-14, 1.387778780781445676E-14, 24.50000000000000000 ) ) ;
#28138=CARTESIAN_POINT ( 'NONE',  ( -19.84344116185557283, 2.497567387674354489, 7.652108011868850035 ) ) ;
#28142=CARTESIAN_POINT ( 'NONE',  ( 7.856594496258195726, 4.390207617113981442, 1.500000000000001332 ) ) ;
#28143=CARTESIAN_POINT ( 'NONE',  ( 1.750000000000008660, 16.48749217771910125, -0.6213203435596476032 ) ) ;
#28145=CARTESIAN_POINT ( 'NONE',  ( 18.67280747382545769, -7.164419611389377884, 6.149077423860698666 ) ) ;
#28146=CARTESIAN_POINT ( 'NONE',  ( -5.976018955020172108, 19.08630078664910812, 18.34798005863227388 ) ) ;
#28149=ORIENTED_EDGE ( 'NONE', *, *, #16290, .T. ) ;
#28150=CARTESIAN_POINT ( 'NONE',  ( -7.869584159753960861, 10.39565510934976977, 24.50000000000000000 ) ) ;
#28151=DIRECTION ( 'NONE',  ( -0.000000000000000000, -0.000000000000000000, -1.000000000000000000 ) ) ;
#28155=FACE_OUTER_BOUND ( 'NONE', #12686, .T. ) ;
#28156=CARTESIAN_POINT ( 'NONE',  ( -4.102102735472396233, 8.549050687778207092, 13.00000000000000178 ) ) ;
#28158=VERTEX_POINT ( 'NONE', #4669 ) ;
#28160=CARTESIAN_POINT ( 'NONE',  ( -7.671759676023399699, -15.25818751172876198, 6.783738457429058677 ) ) ;
#28164=CARTESIAN_POINT ( 'NONE',  ( 15.51722275458701894, -7.010743380608707831, 18.63641924841378028 ) ) ;
#28166=CARTESIAN_POINT ( 'NONE',  ( 4.270667257859593668, 16.49544336893745111, 7.632642797338977658 ) ) ;
#28168=CARTESIAN_POINT ( 'NONE',  ( -19.73562743738981951, 3.350138464993958287, 6.111214848085761986 ) ) ;
#28169=CARTESIAN_POINT ( 'NONE',  ( 11.66141461333273810, 12.47704237144458084, 6.782048567692550378 ) ) ;
#28174=B_SPLINE_CURVE_WITH_KNOTS ( 'NONE', 3,
 ( #20375, #3541, #1659, #1350, #25200, #3844, #18505, #27704, #6333, #27410, #15848, #25365, #3998, #8379, #8830, #30192, #27867, #20209, #11329, #6028 ),
 .UNSPECIFIED., .F., .F.,
 ( 4, 2, 2, 2, 2, 2, 2, 2, 2, 4 ),
 ( 0.000000000000000000, 0.06250000000000163758, 0.1250000000000032752, 0.1875000000000049127, 0.2187500000000050793, 0.2500000000000052736, 0.3125000000000039413, 0.3750000000000026645, 0.4375000000000013323, 0.5000000000000000000 ),
 .UNSPECIFIED. ) ;
#28177=CARTESIAN_POINT ( 'NONE',  ( 7.856594496258195726, 4.390207617113981442, 1.500000000000001332 ) ) ;
#28178=ORIENTED_EDGE ( 'NONE', *, *, #4837, .T. ) ;
#28179=CARTESIAN_POINT ( 'NONE',  ( 16.87925085231059796, 2.194398682741037554, 19.21496526180053621 ) ) ;
#28180=PLANE ( 'NONE',  #17775 ) ;
#28182=CARTESIAN_POINT ( 'NONE',  ( -0.09481216811183805493, -20.01790837231453679, 7.557577766377196582 ) ) ;
#28186=CARTESIAN_POINT ( 'NONE',  ( -17.06158983937614337, 0.7019473037495057577, 19.69140814234746273 ) ) ;
#28188=ORIENTED_EDGE ( 'NONE', *, *, #26145, .F. ) ;
#28189=CARTESIAN_POINT ( 'NONE',  ( -6.476765594709835483, 15.80122980073540084, 6.392658652357120275 ) ) ;
#28193=VECTOR ( 'NONE', #10236, 1000.000000000000000 ) ;
#28195=CARTESIAN_POINT ( 'NONE',  ( -15.66344362052393002, 12.43669181132026580, 7.528076282304597022 ) ) ;
#28202=CARTESIAN_POINT ( 'NONE',  ( 8.999114229549594057, -0.1262659238204522361, 1.500000000000001332 ) ) ;
#28206=CARTESIAN_POINT ( 'NONE',  ( 16.91972452348793610, -3.442972353390052920, 24.50000000000000000 ) ) ;
#28210=VERTEX_POINT ( 'NONE', #18568 ) ;
#28211=CIRCLE ( 'NONE', #24219, 0.7500000000000006661 ) ;
#28212=AXIS2_PLACEMENT_3D ( 'NONE', #10398, #17886, #24423 ) ;
#28213=CYLINDRICAL_SURFACE ( 'NONE', #3651, 10.00000000000000000 ) ;
#28217=CARTESIAN_POINT ( 'NONE',  ( -14.71865621670870894, -8.659590923294997467, 19.08844262864050023 ) ) ;
#28218=CARTESIAN_POINT ( 'NONE',  ( 1.590931199639277205, -16.99685872686718824, 18.73314399819311760 ) ) ;
#28219=CARTESIAN_POINT ( 'NONE',  ( 16.77777292147013810, 2.975267875541937723, 18.36582235739946611 ) ) ;
#28220=EDGE_CURVE ( 'NONE', #22179, #25840, #22295, .T. ) ;
#28222=ADVANCED_FACE ( 'NONE', ( #28689 ), #26352, .F. ) ;
#28223=CARTESIAN_POINT ( 'NONE',  ( -16.81737828845395910, 2.629481162813160910, 19.11611934778430921 ) ) ;
#28225=CARTESIAN_POINT ( 'NONE',  ( -15.85879827683067944, 12.21494667905097131, 6.041646659195333058 ) ) ;
#28227=CARTESIAN_POINT ( 'NONE',  ( 10.47960520055065992, -7.757439966934453146, 1.500000000000001332 ) ) ;
#28235=CARTESIAN_POINT ( 'NONE',  ( 15.52089561533224504, 12.61365839305098646, 19.60917204426169747 ) ) ;
#28236=DIRECTION ( 'NONE',  ( 0.000000000000000000, 0.000000000000000000, 1.000000000000000000 ) ) ;
#28237=CARTESIAN_POINT ( 'NONE',  ( 8.999114229549594057, -0.1262659238204522361, 1.500000000000001332 ) ) ;
#28242=EDGE_CURVE ( 'NONE', #950, #15032, #373, .T. ) ;
#28243=ORIENTED_EDGE ( 'NONE', *, *, #24861, .T. ) ;
#28245=CARTESIAN_POINT ( 'NONE',  ( -16.98316914218901985, 1.504314895146021236, 7.643931100913408550 ) ) ;
#28247=CARTESIAN_POINT ( 'NONE',  ( 14.53924466656745018, 13.73408656550489937, 20.22386025856689074 ) ) ;
#28249=ORIENTED_EDGE ( 'NONE', *, *, #13973, .T. ) ;
#28253=CARTESIAN_POINT ( 'NONE',  ( 18.70304204834580020, -7.134633872344111616, 6.233981582756856987 ) ) ;
#28254=AXIS2_PLACEMENT_3D ( 'NONE', #13159, #22651, #1303 ) ;
#28255=CYLINDRICAL_SURFACE ( 'NONE', #10540, 0.7500000000000002220 ) ;
#28258=ORIENTED_EDGE ( 'NONE', *, *, #414, .T. ) ;
#28260=VECTOR ( 'NONE', #27775, 1000.000000000000000 ) ;
#28265=CARTESIAN_POINT ( 'NONE',  ( -6.789382699754180628, 18.83122862112907470, 19.89182036555910571 ) ) ;
#28267=DIRECTION ( 'NONE',  ( 1.000000000000000000, 0.000000000000000000, 0.000000000000000000 ) ) ;
#28268=DIRECTION ( 'NONE',  ( 0.6548607339452890974, 0.7557495743542548272, 0.000000000000000000 ) ) ;
#28271=VERTEX_POINT ( 'NONE', #23421 ) ;
#28279=DIRECTION ( 'NONE',  ( -0.000000000000000000, -0.000000000000000000, 1.000000000000000000 ) ) ;
#28280=DIRECTION ( 'NONE',  ( 0.000000000000000000, 0.000000000000000000, -1.000000000000000000 ) ) ;
#28281=CIRCLE ( 'NONE', #30761, 9.482273699623480212 ) ;
#28283=ADVANCED_FACE ( 'NONE', ( #25483 ), #20631, .F. ) ;
#28285=AXIS2_PLACEMENT_3D ( 'NONE', #18154, #30597, #2059 ) ;
#28288=VERTEX_POINT ( 'NONE', #15800 ) ;
#28293=DIRECTION ( 'NONE',  ( -0.4154150130018860465, -0.9096319953545185522, 0.000000000000000000 ) ) ;
#28295=CARTESIAN_POINT ( 'NONE',  ( -13.88720712120798240, 9.928229803729504255, 6.037360021877314686 ) ) ;
#28299=VECTOR ( 'NONE', #13352, 1000.000000000000000 ) ;
#28300=ORIENTED_EDGE ( 'NONE', *, *, #18240, .T. ) ;
#28304=CARTESIAN_POINT ( 'NONE',  ( -0.6388627779519727712, -20.00771244368417712, 19.11611934778430921 ) ) ;
#28307=CARTESIAN_POINT ( 'NONE',  ( -7.726154291500659355, -15.22816856119838924, 6.995624166085161910 ) ) ;
#28308=EDGE_CURVE ( 'NONE', #5896, #17481, #6744, .T. ) ;
#28309=CARTESIAN_POINT ( 'NONE',  ( 16.17735844207722806, -3.336236224685152685, 24.50000000000000000 ) ) ;
#28310=CARTESIAN_POINT ( 'NONE',  ( 1.638502901550995761, -16.99392728441679878, 19.89182036555910571 ) ) ;
#28315=LINE ( 'NONE', #23310, #283 ) ;
#28317=EDGE_LOOP ( 'NONE', ( #10471, #9725, #9261, #19496 ) ) ;
#28320=CARTESIAN_POINT ( 'NONE',  ( -13.29453093330978319, 10.66243031780445527, 20.34789198813115974 ) ) ;
#28323=CARTESIAN_POINT ( 'NONE',  ( -18.30192086700451881, -8.065271870204643534, 20.14992337338002315 ) ) ;
#28324=CARTESIAN_POINT ( 'NONE',  ( -15.39438215884103478, -7.285634741961048988, 20.19668224736330941 ) ) ;
#28331=DIRECTION ( 'NONE',  ( -0.000000000000000000, -0.000000000000000000, 1.000000000000000000 ) ) ;
#28332=CARTESIAN_POINT ( 'NONE',  ( -7.548823014270604759, 5.738360882150024267, 21.50000000000000000 ) ) ;
#28333=ORIENTED_EDGE ( 'NONE', *, *, #28242, .F. ) ;
#28335=CARTESIAN_POINT ( 'NONE',  ( 15.42605794595426971, -7.198932956632622115, 19.77662771831109367 ) ) ;
#28336=CARTESIAN_POINT ( 'NONE',  ( 6.249808329856143985, 19.01727106391103916, 6.420335371522007506 ) ) ;
#28338=CARTESIAN_POINT ( 'NONE',  ( 6.071284049926378934, 19.07508289763275400, 19.96783386855779341 ) ) ;
#28341=LINE ( 'NONE', #14122, #9344 ) ;
#28346=CARTESIAN_POINT ( 'NONE',  ( -14.69412328735588069, 13.56780452301002526, 6.913388067999404640 ) ) ;
#28347=EDGE_CURVE ( 'NONE', #24333, #12567, #2904, .T. ) ;
#28349=CARTESIAN_POINT ( 'NONE',  ( -15.46558767506644116, -7.123678207069781720, 7.359006845440219102 ) ) ;
#28351=CARTESIAN_POINT ( 'NONE',  ( 16.74250988114177474, 3.198928528055117404, 18.34798005863078885 ) ) ;
#28355=CARTESIAN_POINT ( 'NONE',  ( -0.4512825100096616859, -20.01288639008904724, 7.272049892295485485 ) ) ;
#28356=AXIS2_PLACEMENT_3D ( 'NONE', #12634, #19628, #24470 ) ;
#28359=CARTESIAN_POINT ( 'NONE',  ( -16.96496223448354357, 1.652369715233089176, 20.34789198813115263 ) ) ;
#28361=ORIENTED_EDGE ( 'NONE', *, *, #27865, .F. ) ;
#28366=EDGE_LOOP ( 'NONE', ( #308, #2490, #12028, #29654 ) ) ;
#28367=CARTESIAN_POINT ( 'NONE',  ( 5.035381156335493991, 19.35612728853641329, 18.37545668562167478 ) ) ;
#28372=ORIENTED_EDGE ( 'NONE', *, *, #16623, .F. ) ;
#28373=CARTESIAN_POINT ( 'NONE',  ( 16.18635831298871963, -5.444400941729615973, 19.58863275299554019 ) ) ;
#28374=FACE_OUTER_BOUND ( 'NONE', #4588, .T. ) ;
#28377=VERTEX_POINT ( 'NONE', #16111 ) ;
#28382=CARTESIAN_POINT ( 'NONE',  ( 0.6517800496514684072, -17.02970683165549914, 18.34727598691068096 ) ) ;
#28383=AXIS2_PLACEMENT_3D ( 'NONE', #20215, #17899, #27413 ) ;
#28384=CARTESIAN_POINT ( 'NONE',  ( 1.795183039316615270, -16.98367886218520795, 6.672349528511551497 ) ) ;
#28385=CARTESIAN_POINT ( 'NONE',  ( -15.16517293421788537, -7.781889191988407006, 20.34789198813115263 ) ) ;
#28386=CARTESIAN_POINT ( 'NONE',  ( 5.687793815610356241, -6.974883619896809606, 1.500000000000001332 ) ) ;
#28387=CARTESIAN_POINT ( 'NONE',  ( 16.76050819728944319, 3.085824932809439591, 18.35377592296120497 ) ) ;
#28389=CARTESIAN_POINT ( 'NONE',  ( -19.71887672257059165, 3.447422735172823050, 19.00652017443069752 ) ) ;
#28393=EDGE_LOOP ( 'NONE', ( #5877, #27912, #14164, #14886 ) ) ;
#28397=DIRECTION ( 'NONE',  ( -0.000000000000000000, -0.000000000000000000, 1.000000000000000000 ) ) ;
#28399=DIRECTION ( 'NONE',  ( 0.000000000000000000, 0.000000000000000000, -1.000000000000000000 ) ) ;
#28404=CARTESIAN_POINT ( 'NONE',  ( -19.94392260440443110, 1.716525891962611183, 7.280727868105637768 ) ) ;
#28406=DIRECTION ( 'NONE',  ( 1.000000000000000000, 0.000000000000000000, 0.000000000000000000 ) ) ;
#28410=DIRECTION ( 'NONE',  ( 0.5406408174555974444, 0.8412535328311813165, 0.000000000000000000 ) ) ;
#28411=DIRECTION ( 'NONE',  ( -0.000000000000000000, -0.000000000000000000, 1.000000000000000000 ) ) ;
#28420=CARTESIAN_POINT ( 'NONE',  ( -6.065925884476026653, 15.94726461227263847, 18.50655187082627862 ) ) ;
#28421=CARTESIAN_POINT ( 'NONE',  ( -10.51100353655187192, -17.01524272303503338, 5.652196082369963293 ) ) ;
#28423=ORIENTED_EDGE ( 'NONE', *, *, #29545, .F. ) ;
#28425=EDGE_CURVE ( 'NONE', #1760, #22306, #1396, .T. ) ;
#28427=DIRECTION ( 'NONE',  ( -0.000000000000000000, -0.000000000000000000, -1.000000000000000000 ) ) ;
#28431=LINE ( 'NONE', #28580, #21762 ) ;
#28432=CARTESIAN_POINT ( 'NONE',  ( 12.72536390617885438, -2.839914339433650348, 24.50000000000000000 ) ) ;
#28433=CARTESIAN_POINT ( 'NONE',  ( 5.009972004274191093, 16.26741710164063548, 6.782064869129510676 ) ) ;
#28436=CARTESIAN_POINT ( 'NONE',  ( -0.6573828633908636032, -19.98919327533018020, 19.47728749465737863 ) ) ;
#28443=CARTESIAN_POINT ( 'NONE',  ( -14.00715867683510751, 9.770345079980357283, 6.521906765011494578 ) ) ;
#28444=FACE_OUTER_BOUND ( 'NONE', #837, .T. ) ;
#28450=ADVANCED_FACE ( 'NONE', ( #24503 ), #18120, .T. ) ;
#28455=CARTESIAN_POINT ( 'NONE',  ( -0.5107318660475972383, -20.01137538934480631, 19.87181966307587544 ) ) ;
#28457=CARTESIAN_POINT ( 'NONE',  ( -8.423436389728856000, -14.82351904252669250, 7.643931100913408550 ) ) ;
#28458=DIRECTION ( 'NONE',  ( 0.000000000000000000, 0.000000000000000000, -1.000000000000000000 ) ) ;
#28459=CARTESIAN_POINT ( 'NONE',  ( 1.367976436446960209, -19.97081545247030476, 19.25672174529527325 ) ) ;
#28464=CARTESIAN_POINT ( 'NONE',  ( 14.52517991353747107, 13.77415465259964655, 18.50655187082627862 ) ) ;
#28466=ADVANCED_FACE ( 'NONE', ( #22782 ), #13401, .T. ) ;
#28472=CARTESIAN_POINT ( 'NONE',  ( -18.15420570657826005, -8.392844156286328072, 18.37250658438898654 ) ) ;
#28475=ORIENTED_EDGE ( 'NONE', *, *, #13014, .T. ) ;
#28476=CARTESIAN_POINT ( 'NONE',  ( 7.869584159753955532, 10.39565510934977333, 24.50000000000000000 ) ) ;
#28484=CARTESIAN_POINT ( 'NONE',  ( -17.20435420003449423, -1.463329469628170898, 1.500000000000000000 ) ) ;
#28485=CARTESIAN_POINT ( 'NONE',  ( 5.517068924551614906, 19.24285362756905471, 5.670038381137163519 ) ) ;
#28486=EDGE_CURVE ( 'NONE', #15211, #2038, #29807, .T. ) ;
#28488=FACE_OUTER_BOUND ( 'NONE', #14396, .T. ) ;
#28492=CARTESIAN_POINT ( 'NONE',  ( 9.749114229549594057, -0.1262659238204522361, 1.500000000000001332 ) ) ;
#28501=CARTESIAN_POINT ( 'NONE',  ( -0.2808233399669959884, -20.01605574108312524, 5.862424720655265098 ) ) ;
#28503=CARTESIAN_POINT ( 'NONE',  ( 2.703030265324084080, -12.75514121382991384, 1.500000000000001332 ) ) ;
#28509=LINE ( 'NONE', #9633, #16549 ) ;
#28511=ORIENTED_EDGE ( 'NONE', *, *, #19304, .F. ) ;
#28512=CARTESIAN_POINT ( 'NONE',  ( -15.95879822657219194, 12.05485308878816397, 6.919864475265776527 ) ) ;
#28513=EDGE_CURVE ( 'NONE', #10973, #24160, #16275, .T. ) ;
#28514=DIRECTION ( 'NONE',  ( 0.000000000000000000, 0.000000000000000000, 1.000000000000000000 ) ) ;
#28522=CARTESIAN_POINT ( 'NONE',  ( 18.68320837179354044, -7.186693706611503529, 18.82680253904184298 ) ) ;
#28523=CARTESIAN_POINT ( 'NONE',  ( 16.56823697822719055, 4.133291823432034384, 19.69140814234746273 ) ) ;
#28526=CARTESIAN_POINT ( 'NONE',  ( 15.47699552840392734, -7.094814489915346911, 18.72771030977187223 ) ) ;
#28528=VERTEX_POINT ( 'NONE', #6570 ) ;
#28531=CARTESIAN_POINT ( 'NONE',  ( 1.745046693156363071, -16.98705356654486209, 6.341840715582230281 ) ) ;
#28538=CARTESIAN_POINT ( 'NONE',  ( -16.95096719779282068, 1.761153487549138585, 18.35377592296120497 ) ) ;
#28539=CARTESIAN_POINT ( 'NONE',  ( 18.35307960222155899, -7.992235168165439774, 5.652196082367003882 ) ) ;
#28543=EDGE_LOOP ( 'NONE', ( #12776, #29017, #28188, #5190 ) ) ;
#28558=CIRCLE ( 'NONE', #26079, 20.00000000000000000 ) ;
#28561=AXIS2_PLACEMENT_3D ( 'NONE', #23858, #17148, #24323 ) ;
#28564=ORIENTED_EDGE ( 'NONE', *, *, #23044, .T. ) ;
#28567=CARTESIAN_POINT ( 'NONE',  ( 10.58714538945784867, -13.39479915613590499, 19.85459532544248162 ) ) ;
#28572=CARTESIAN_POINT ( 'NONE',  ( 15.40878509683846431, -7.233835689978969974, 6.973843882838225205 ) ) ;
#28573=CIRCLE ( 'NONE', #24580, 9.482273699623480212 ) ;
#28577=ORIENTED_EDGE ( 'NONE', *, *, #2777, .F. ) ;
#28578=DIRECTION ( 'NONE',  ( -0.000000000000000000, -0.000000000000000000, 1.000000000000000000 ) ) ;
#28580=CARTESIAN_POINT ( 'NONE',  ( 7.974144905643786529, 5.130938270761634890, 13.00000000000000178 ) ) ;
#28583=CARTESIAN_POINT ( 'NONE',  ( 4.989870534578006556, 16.27408959345230954, 6.385774490351134425 ) ) ;
#28586=CARTESIAN_POINT ( 'NONE',  ( 0.2238118478526132105, -19.99918941848005005, 18.34726407865098707 ) ) ;
#28587=FACE_OUTER_BOUND ( 'NONE', #25433, .T. ) ;
#28589=ADVANCED_FACE ( 'NONE', ( #7177 ), #19179, .F. ) ;
#28593=EDGE_LOOP ( 'NONE', ( #11729, #5145, #24340, #12132 ) ) ;
#28594=CARTESIAN_POINT ( 'NONE',  ( 12.35522425158188931, 11.74279415389956327, 18.34798005863078885 ) ) ;
#28598=CARTESIAN_POINT ( 'NONE',  ( 8.499586724479435418, 2.959227181723830036, 1.500000000000001332 ) ) ;
#28603=CARTESIAN_POINT ( 'NONE',  ( -0.2861250491275360575, -20.01582202454545367, 20.12545155307891065 ) ) ;
#28605=CIRCLE ( 'NONE', #7182, 0.7500000000000006661 ) ;
#28612=CARTESIAN_POINT ( 'NONE',  ( 14.19710122452049106, 14.11195047426184601, 19.25672174529527325 ) ) ;
#28613=CARTESIAN_POINT ( 'NONE',  ( -10.47960520055065636, -7.757439966934454034, 1.500000000000001332 ) ) ;
#28618=LINE ( 'NONE', #7241, #20784 ) ;
#28619=CARTESIAN_POINT ( 'NONE',  ( -19.92837724392305532, 1.693712106646815929, 7.272192800924334399 ) ) ;
#28620=CARTESIAN_POINT ( 'NONE',  ( 19.76423196911359881, 3.064691114365036828, 7.652108011868850923 ) ) ;
#28621=ADVANCED_FACE ( 'NONE', ( #1 ), #16690, .F. ) ;
#28622=EDGE_CURVE ( 'NONE', #3110, #28626, #21666, .T. ) ;
#28626=VERTEX_POINT ( 'NONE', #23855 ) ;
#28627=CARTESIAN_POINT ( 'NONE',  ( -10.47960520055065636, -7.757439966934454034, 24.50000000000000000 ) ) ;
#28629=CARTESIAN_POINT ( 'NONE',  ( -14.72004833196315765, 13.56602982695842030, 6.974106381145714018 ) ) ;
#28631=CARTESIAN_POINT ( 'NONE',  ( 11.91798344328409875, -16.06126763266894386, 19.08830981656265280 ) ) ;
#28634=CARTESIAN_POINT ( 'NONE',  ( 17.96497429814991875, -8.830595420483337676, 19.77662771831109367 ) ) ;
#28635=CARTESIAN_POINT ( 'NONE',  ( 4.731053074881898191, 16.35701261131972473, 5.940635272151477686 ) ) ;
#28637=ORIENTED_EDGE ( 'NONE', *, *, #6228, .T. ) ;
#28638=CARTESIAN_POINT ( 'NONE',  ( 14.84769773172387630, 13.42619037096054413, 7.652108011868850035 ) ) ;
#28640=PLANE ( 'NONE',  #18818 ) ;
#28642=ORIENTED_EDGE ( 'NONE', *, *, #20439, .T. ) ;
#28643=CARTESIAN_POINT ( 'NONE',  ( -0.9307681286967859347, 9.436481611552762772, 13.00000000000000178 ) ) ;
#28647=ORIENTED_EDGE ( 'NONE', *, *, #28622, .F. ) ;
#28648=CARTESIAN_POINT ( 'NONE',  ( -18.32390295431234861, -8.059524160852179264, 5.862424720655265098 ) ) ;
#28651=CARTESIAN_POINT ( 'NONE',  ( 14.79453494486352483, 13.45878767717418789, 7.652108011868850035 ) ) ;
#28652=CARTESIAN_POINT ( 'NONE',  ( 0.2430132208050684306, -17.02994525543105908, 5.796888747622817029 ) ) ;
#28654=CARTESIAN_POINT ( 'NONE',  ( -6.962021646281576714, -6.437683520590145037, 1.500000000000001332 ) ) ;
#28660=CARTESIAN_POINT ( 'NONE',  ( 11.55802067824463464, -16.34381896053850625, 20.19593175699879595 ) ) ;
#28663=EDGE_CURVE ( 'NONE', #4676, #7304, #25691, .T. ) ;
#28669=VERTEX_POINT ( 'NONE', #4319 ) ;
#28675=FACE_OUTER_BOUND ( 'NONE', #8760, .T. ) ;
#28676=CARTESIAN_POINT ( 'NONE',  ( -15.66344362052393002, 12.43669181132025514, 20.22386025856689784 ) ) ;
#28679=CARTESIAN_POINT ( 'NONE',  ( 15.76152542338162377, -6.481515897793713066, 18.34727598691068096 ) ) ;
#28685=EDGE_CURVE ( 'NONE', #24319, #21410, #25544, .T. ) ;
#28687=AXIS2_PLACEMENT_3D ( 'NONE', #38, #2538, #9408 ) ;
#28688=FACE_OUTER_BOUND ( 'NONE', #28366, .T. ) ;
#28689=FACE_OUTER_BOUND ( 'NONE', #7254, .T. ) ;
#28692=CARTESIAN_POINT ( 'NONE',  ( -19.83214989528428163, 2.722369515932096640, 18.36582235739946611 ) ) ;
#28695=CARTESIAN_POINT ( 'NONE',  ( -13.37849590052435111, 10.56201291103764106, 7.652108011868850035 ) ) ;
#28698=ORIENTED_EDGE ( 'NONE', *, *, #12074, .T. ) ;
#28700=CARTESIAN_POINT ( 'NONE',  ( -8.743977807160096205, -3.668292057955974350, 13.00000000000000178 ) ) ;
#28703=DIRECTION ( 'NONE',  ( -0.6548607339452852116, 0.7557495743542581579, 0.000000000000000000 ) ) ;
#28705=DIRECTION ( 'NONE',  ( 0.000000000000000000, 0.000000000000000000, -1.000000000000000000 ) ) ;
#28709=DIRECTION ( 'NONE',  ( -0.000000000000000000, -0.000000000000000000, -1.000000000000000000 ) ) ;
#28715=CARTESIAN_POINT ( 'NONE',  ( 15.81223571690236440, -6.365019318618790223, 7.652108011868850035 ) ) ;
#28718=AXIS2_PLACEMENT_3D ( 'NONE', #17360, #26721, #15160 ) ;
#28719=CARTESIAN_POINT ( 'NONE',  ( 14.88222593340887023, 13.36111339922579866, 7.652108011868850035 ) ) ;
#28720=VERTEX_POINT ( 'NONE', #30516 ) ;
#28723=DIRECTION ( 'NONE',  ( 1.000000000000000000, 0.000000000000000000, 0.000000000000000000 ) ) ;
#28724=CARTESIAN_POINT ( 'NONE',  ( -18.44536497093016791, -7.731176935556637986, 6.386539667786092167 ) ) ;
#28726=AXIS2_PLACEMENT_3D ( 'NONE', #27336, #972, #29362 ) ;
#28737=LINE ( 'NONE', #28895, #26741 ) ;
#28748=ORIENTED_EDGE ( 'NONE', *, *, #9021, .F. ) ;
#28751=CARTESIAN_POINT ( 'NONE',  ( 0.000000000000000000, 0.000000000000000000, 1.500000000000001332 ) ) ;
#28754=LINE ( 'NONE', #19690, #13781 ) ;
#28757=VERTEX_POINT ( 'NONE', #1835 ) ;
#28758=CARTESIAN_POINT ( 'NONE',  ( 0.1433833641520081137, -17.02852539342428884, 20.12545155307891065 ) ) ;
#28759=DIRECTION ( 'NONE',  ( 0.000000000000000000, 0.000000000000000000, 1.000000000000000000 ) ) ;
#28760=CARTESIAN_POINT ( 'NONE',  ( 1.583371619456036994, -16.99707458536919802, 18.73743063545763121 ) ) ;
#28763=DIRECTION ( 'NONE',  ( -0.000000000000000000, -0.000000000000000000, 1.000000000000000000 ) ) ;
#28764=CARTESIAN_POINT ( 'NONE',  ( 14.53258460577763067, 13.76634464516646972, 20.19593175699879595 ) ) ;
#28765=PLANE ( 'NONE',  #27587 ) ;
#28770=CARTESIAN_POINT ( 'NONE',  ( -17.59999711780629283, -9.536506973003668008, 6.782048567692550378 ) ) ;
#28772=CARTESIAN_POINT ( 'NONE',  ( 5.881244434206234217, 6.812559277181991391, 21.50000000000000000 ) ) ;
#28774=CARTESIAN_POINT ( 'NONE',  ( -15.17962487735951527, -7.751670534285732828, 18.34777357837151968 ) ) ;
#28780=DIRECTION ( 'NONE',  ( 0.000000000000000000, 0.000000000000000000, 1.000000000000000000 ) ) ;
#28781=DIRECTION ( 'NONE',  ( 0.000000000000000000, 0.000000000000000000, 1.000000000000000000 ) ) ;
#28782=CARTESIAN_POINT ( 'NONE',  ( -12.72741959552008773, 11.30275801665550617, 6.864725433338323413 ) ) ;
#28785=CARTESIAN_POINT ( 'NONE',  ( 16.18505772754830119, -5.447928388648084486, 19.61324152429827095 ) ) ;
#28787=ORIENTED_EDGE ( 'NONE', *, *, #16224, .F. ) ;
#28788=CARTESIAN_POINT ( 'NONE',  ( 4.270667257859590116, 16.49544336893744045, 20.32842677360128292 ) ) ;
#28790=CARTESIAN_POINT ( 'NONE',  ( 11.99367014178017321, 12.13468339478709979, 7.500147780736496017 ) ) ;
#28794=ORIENTED_EDGE ( 'NONE', *, *, #8848, .F. ) ;
#28796=EDGE_CURVE ( 'NONE', #8561, #19541, #18167, .T. ) ;
#28799=DIRECTION ( 'NONE',  ( 1.000000000000000000, 0.000000000000000000, 0.000000000000000000 ) ) ;
#28802=ORIENTED_EDGE ( 'NONE', *, *, #19112, .F. ) ;
#28803=AXIS2_PLACEMENT_3D ( 'NONE', #26584, #363, #7552 ) ;
#28804=CARTESIAN_POINT ( 'NONE',  ( -18.39183130958318557, -7.903152449895378240, 7.272049892295485485 ) ) ;
#28815=ADVANCED_FACE ( 'NONE', ( #26781, #5409 ), #16789, .F. ) ;
#28817=CARTESIAN_POINT ( 'NONE',  ( -6.045292009791579879, 15.95527889494839968, 7.545655578832111132 ) ) ;
#28822=ORIENTED_EDGE ( 'NONE', *, *, #8469, .T. ) ;
#28824=LINE ( 'NONE', #27098, #3180 ) ;
#28830=CARTESIAN_POINT ( 'NONE',  ( 18.62671295915898639, -7.331958482175751968, 20.06253562465620632 ) ) ;
#28831=CARTESIAN_POINT ( 'NONE',  ( -15.89566665641789456, 12.13797781250046626, 19.85730954408919047 ) ) ;
#28833=ORIENTED_EDGE ( 'NONE', *, *, #2266, .F. ) ;
#28834=DIRECTION ( 'NONE',  ( 0.000000000000000000, 0.000000000000000000, 1.000000000000000000 ) ) ;
#28836=VERTEX_POINT ( 'NONE', #22077 ) ;
#28838=ADVANCED_FACE ( 'NONE', ( #26144 ), #21620, .F. ) ;
#28840=VECTOR ( 'NONE', #5957, 1000.000000000000114 ) ;
#28842=EDGE_CURVE ( 'NONE', #19044, #2106, #15355, .T. ) ;
#28846=CARTESIAN_POINT ( 'NONE',  ( -7.796062812047480861, -15.18940472835274669, 18.82680253904184298 ) ) ;
#28848=CYLINDRICAL_SURFACE ( 'NONE', #16512, 9.482273699623480212 ) ;
#28849=LINE ( 'NONE', #3414, #18012 ) ;
#28853=FACE_OUTER_BOUND ( 'NONE', #24735, .T. ) ;
#28858=VERTEX_POINT ( 'NONE', #19740 ) ;
#28859=B_SPLINE_CURVE_WITH_KNOTS ( 'NONE', 3,
 ( #18283, #21053, #1738, #27804, #6430, #15946, #4086, #13614, #18589, #20909, #9072, #23094, #18732, #28100, #13901, #16696, #17313, #10136 ),
 .UNSPECIFIED., .F., .F.,
 ( 4, 2, 2, 2, 2, 2, 2, 2, 4 ),
 ( 0.000000000000000000, 0.0003967869494442877220, 0.0007935738988885754439, 0.001190360848332863274, 0.001587147797777150888, 0.001983934747221438501, 0.002380721696665726549, 0.002777508646110014162, 0.003174295595554301776 ),
 .UNSPECIFIED. ) ;
#28863=CARTESIAN_POINT ( 'NONE',  ( -5.450136891332532763, 19.26184010647175882, 7.500898271101006820 ) ) ;
#28864=CARTESIAN_POINT ( 'NONE',  ( -15.57492749417239253, -6.866608492817582565, 6.782064869129510676 ) ) ;
#28866=EDGE_CURVE ( 'NONE', #21892, #26251, #10396, .T. ) ;
#28867=ORIENTED_EDGE ( 'NONE', *, *, #13732, .F. ) ;
#28869=ORIENTED_EDGE ( 'NONE', *, *, #29811, .F. ) ;
#28872=CARTESIAN_POINT ( 'NONE',  ( -17.76782356872499946, -9.182228809334535669, 20.15039051365864253 ) ) ;
#28875=CARTESIAN_POINT ( 'NONE',  ( 12.35846532919128826, 11.73919094318043577, 7.652108011868850035 ) ) ;
#28876=ORIENTED_EDGE ( 'NONE', *, *, #12606, .T. ) ;
#28877=CARTESIAN_POINT ( 'NONE',  ( 18.52307105101189677, -7.590397700845933571, 7.559636331181775581 ) ) ;
#28879=AXIS2_PLACEMENT_3D ( 'NONE', #15592, #27151, #24955 ) ;
#28881=EDGE_CURVE ( 'NONE', #4157, #29398, #23809, .T. ) ;
#28883=CARTESIAN_POINT ( 'NONE',  ( 3.826954525806324448, 16.61697297626112046, 5.678370764302467677 ) ) ;
#28886=CARTESIAN_POINT ( 'NONE',  ( -18.15420570657826360, -8.392844156286336954, 5.676722608126685721 ) ) ;
#28895=CARTESIAN_POINT ( 'NONE',  ( -12.72536390617885260, -2.839914339433650348, 24.50000000000000000 ) ) ;
#28896=DIRECTION ( 'NONE',  ( -1.000000000000000000, 0.000000000000000000, 0.000000000000000000 ) ) ;
#28900=CYLINDRICAL_SURFACE ( 'NONE', #5931, 0.7500000000000002220 ) ;
#28906=ORIENTED_EDGE ( 'NONE', *, *, #20517, .F. ) ;
#28907=DIRECTION ( 'NONE',  ( 1.000000000000000000, 0.000000000000000000, 0.000000000000000000 ) ) ;
#28908=DIRECTION ( 'NONE',  ( -0.000000000000000000, -0.000000000000000000, 1.000000000000000000 ) ) ;
#28911=CARTESIAN_POINT ( 'NONE',  ( -9.636724589035630117, -17.52522580332708202, 6.788986777570690023 ) ) ;
#28912=ORIENTED_EDGE ( 'NONE', *, *, #15478, .T. ) ;
#28913=AXIS2_PLACEMENT_3D ( 'NONE', #18734, #13616, #23097 ) ;
#28915=ORIENTED_EDGE ( 'NONE', *, *, #7895, .T. ) ;
#28916=CARTESIAN_POINT ( 'NONE',  ( -0.2229293267576271109, -17.01997447887395509, 19.22654678686458141 ) ) ;
#28918=CARTESIAN_POINT ( 'NONE',  ( -9.702532784345955008, -17.50903092980014009, 6.995624166085161910 ) ) ;
#28919=CARTESIAN_POINT ( 'NONE',  ( 4.172444469959711633, 16.52351170757476950, 18.34727598691068096 ) ) ;
#28920=CARTESIAN_POINT ( 'NONE',  ( 0.9820204223201484117, -19.99380624802880035, 20.13759033520874908 ) ) ;
#28921=ORIENTED_EDGE ( 'NONE', *, *, #28945, .F. ) ;
#28924=CARTESIAN_POINT ( 'NONE',  ( 0.3518703668723784928, -19.99690444156084723, 20.34789198813115263 ) ) ;
#28925=DIRECTION ( 'NONE',  ( 1.000000000000000000, 0.000000000000000000, 0.000000000000000000 ) ) ;
#28928=CARTESIAN_POINT ( 'NONE',  ( -17.62281152098609027, -9.494300025206930727, 6.341840715582230281 ) ) ;
#28929=CARTESIAN_POINT ( 'NONE',  ( -6.294089901980526314, 15.86740633010675516, 7.280727868105637768 ) ) ;
#28930=CARTESIAN_POINT ( 'NONE',  ( -19.94291556179615910, 1.510882595598290079, 6.392525840300333329 ) ) ;
#28941=CARTESIAN_POINT ( 'NONE',  ( 0.5152247662762403646, -17.03071091119059233, 7.626437579292365321 ) ) ;
#28945=EDGE_CURVE ( 'NONE', #18617, #12232, #10384, .T. ) ;
#28946=CARTESIAN_POINT ( 'NONE',  ( -8.072557715923444732, 14.41080185948837311, -0.6213203435596476032 ) ) ;
#28952=CARTESIAN_POINT ( 'NONE',  ( -6.630478080506957639, -6.778663211761441154, 13.00000000000000178 ) ) ;
#28956=CARTESIAN_POINT ( 'NONE',  ( -18.43827498451961944, -7.794211480880298915, 7.080843742048788414 ) ) ;
#28957=DIRECTION ( 'NONE',  ( 1.000000000000000000, 0.000000000000000000, 0.000000000000000000 ) ) ;
#28959=CARTESIAN_POINT ( 'NONE',  ( -0.2229293267576251125, -17.01997447887395509, 6.530762810602277924 ) ) ;
#28968=ORIENTED_EDGE ( 'NONE', *, *, #2144, .F. ) ;
#28970=EDGE_CURVE ( 'NONE', #26160, #16362, #13309, .T. ) ;
#28975=CARTESIAN_POINT ( 'NONE',  ( 15.25015041412931183, 12.96756205105604920, 18.49267272388512140 ) ) ;
#28976=CARTESIAN_POINT ( 'NONE',  ( -10.97902775627723493, -16.73874854128740353, 5.796888747622817029 ) ) ;
#28977=ORIENTED_EDGE ( 'NONE', *, *, #30202, .T. ) ;
#28978=EDGE_CURVE ( 'NONE', #3062, #19423, #1913, .T. ) ;
#28980=CARTESIAN_POINT ( 'NONE',  ( 19.73572331631237731, 3.349230485916621980, 18.35718225375110180 ) ) ;
#28983=CARTESIAN_POINT ( 'NONE',  ( 15.60593903839447982, -6.823719261784396473, 18.47056384035244037 ) ) ;
#28984=ORIENTED_EDGE ( 'NONE', *, *, #11138, .T. ) ;
#28988=CARTESIAN_POINT ( 'NONE',  ( -6.670428619809866788, 18.87372120578244150, 18.64703902303423178 ) ) ;
#28990=AXIS2_PLACEMENT_3D ( 'NONE', #7983, #7811, #5477 ) ;
#28991=CARTESIAN_POINT ( 'NONE',  ( -7.685008110482988819, -15.25093183970989763, 19.14333282897057842 ) ) ;
#28993=LINE ( 'NONE', #9976, #5529 ) ;
#28995=ORIENTED_EDGE ( 'NONE', *, *, #23501, .F. ) ;
#28996=CARTESIAN_POINT ( 'NONE',  ( 9.014152831625311890, -14.43863835250231809, 6.530762810602277924 ) ) ;
#28998=CARTESIAN_POINT ( 'NONE',  ( 9.343263424913798687, -14.23786665604193047, 5.848946451764561516 ) ) ;
#29006=CARTESIAN_POINT ( 'NONE',  ( 18.44003002641402134, -7.744679585886133033, 20.32200205377524682 ) ) ;
#29007=CARTESIAN_POINT ( 'NONE',  ( -15.55757656137109457, -6.908027829072596937, 6.973843882838224317 ) ) ;
#29008=CARTESIAN_POINT ( 'NONE',  ( -13.83213539500865785, 7.758783772730382111, -0.6213203435596476032 ) ) ;
#29012=DIRECTION ( 'NONE',  ( -0.000000000000000000, -0.000000000000000000, 1.000000000000000000 ) ) ;
#29016=LINE ( 'NONE', #314, #26785 ) ;
#29017=ORIENTED_EDGE ( 'NONE', *, *, #16635, .F. ) ;
#29018=EDGE_CURVE ( 'NONE', #18473, #29885, #23713, .T. ) ;
#29019=CARTESIAN_POINT ( 'NONE',  ( -8.430595340551226613, 4.340342926365046594, 1.500000000000001332 ) ) ;
#29020=CARTESIAN_POINT ( 'NONE',  ( 16.56617216130194237, 4.143135851892797206, 19.02573955821369012 ) ) ;
#29023=EDGE_CURVE ( 'NONE', #23911, #22510, #21834, .T. ) ;
#29026=FACE_OUTER_BOUND ( 'NONE', #1457, .T. ) ;
#29030=CARTESIAN_POINT ( 'NONE',  ( 9.824744466605370263, -8.513189541288715745, 1.500000000000001332 ) ) ;
#29040=EDGE_CURVE ( 'NONE', #27397, #5492, #6481, .T. ) ;
#29041=DIRECTION ( 'NONE',  ( -0.000000000000000000, -0.000000000000000000, 1.000000000000000000 ) ) ;
#29042=EDGE_CURVE ( 'NONE', #7938, #28720, #6628, .T. ) ;
#29043=DIRECTION ( 'NONE',  ( -1.000000000000000000, 0.000000000000000000, 0.000000000000000000 ) ) ;
#29053=DIRECTION ( 'NONE',  ( 1.000000000000000000, 0.000000000000000000, 0.000000000000000000 ) ) ;
#29055=FACE_OUTER_BOUND ( 'NONE', #116, .T. ) ;
#29056=DIRECTION ( 'NONE',  ( 1.000000000000000000, 0.000000000000000000, 0.000000000000000000 ) ) ;
#29058=ORIENTED_EDGE ( 'NONE', *, *, #30854, .F. ) ;
#29059=CARTESIAN_POINT ( 'NONE',  ( -10.28466407052217413, -17.15343732189305115, 5.679672709359373073 ) ) ;
#29060=ORIENTED_EDGE ( 'NONE', *, *, #9192, .T. ) ;
#29065=CARTESIAN_POINT ( 'NONE',  ( -3.662523238938586001, -12.47340865698848056, 24.50000000000000000 ) ) ;
#29067=CARTESIAN_POINT ( 'NONE',  ( 4.533306948338440279, 16.41820958405265785, 18.47056384035244037 ) ) ;
#29069=ORIENTED_EDGE ( 'NONE', *, *, #11867, .F. ) ;
#29070=CIRCLE ( 'NONE', #16624, 20.00000000000000000 ) ;
#29072=CARTESIAN_POINT ( 'NONE',  ( 0.000000000000000000, 0.000000000000000000, 21.50000000000000000 ) ) ;
#29073=CARTESIAN_POINT ( 'NONE',  ( 14.25941570111288037, 14.04905143479254725, 18.92976555901915603 ) ) ;
#29074=DIRECTION ( 'NONE',  ( 1.000000000000000000, 0.000000000000000000, 0.000000000000000000 ) ) ;
#29077=AXIS2_PLACEMENT_3D ( 'NONE', #21982, #3121, #12641 ) ;
#29078=EDGE_CURVE ( 'NONE', #23147, #21713, #26734, .T. ) ;
#29079=CARTESIAN_POINT ( 'NONE',  ( -8.647361814388506929, -14.68561526379590809, 20.34789198813115263 ) ) ;
#29081=CARTESIAN_POINT ( 'NONE',  ( -5.549074438232170614, 16.11683645458454706, 5.652196082364320695 ) ) ;
#29082=CARTESIAN_POINT ( 'NONE',  ( -4.163336342344337027E-14, 1.387778780781445676E-14, 24.50000000000000000 ) ) ;
#29083=CARTESIAN_POINT ( 'NONE',  ( -18.35575104603287500, -7.986347210076461423, 18.63641924841378028 ) ) ;
#29084=CARTESIAN_POINT ( 'NONE',  ( 6.974883619896790954, 5.687793815610376669, 1.500000000000001332 ) ) ;
#29085=VERTEX_POINT ( 'NONE', #14091 ) ;
#29089=CARTESIAN_POINT ( 'NONE',  ( -14.82920317518825470, 13.44671003463071735, 7.272049892295485485 ) ) ;
#29090=CARTESIAN_POINT ( 'NONE',  ( 0.6517800498974439805, -17.02970683165111154, 5.651492010659112886 ) ) ;
#29093=CARTESIAN_POINT ( 'NONE',  ( 16.17629920998172821, -5.470921186992126373, 19.02573955821369722 ) ) ;
#29094=LINE ( 'NONE', #24250, #21648 ) ;
#29096=VERTEX_POINT ( 'NONE', #2568 ) ;
#29097=CARTESIAN_POINT ( 'NONE',  ( 4.263339901971998636, 16.49757000336417789, 18.36582235739946611 ) ) ;
#29099=CARTESIAN_POINT ( 'NONE',  ( -7.677470532982090035, -15.25505107808950278, 19.21769074125272780 ) ) ;
#29101=ORIENTED_EDGE ( 'NONE', *, *, #18735, .F. ) ;
#29104=DIRECTION ( 'NONE',  ( -0.000000000000000000, -0.000000000000000000, 1.000000000000000000 ) ) ;
#29105=LINE ( 'NONE', #7746, #860 ) ;
#29109=CARTESIAN_POINT ( 'NONE',  ( 14.79007711409979819, 13.46370387462956586, 5.652912763329819512 ) ) ;
#29110=CARTESIAN_POINT ( 'NONE',  ( -0.6660349346848389862, -20.00682905350634755, 6.641371103590088865 ) ) ;
#29113=ADVANCED_FACE ( 'NONE', ( #368 ), #26588, .F. ) ;
#29114=CARTESIAN_POINT ( 'NONE',  ( -10.47960520055065636, -7.757439966934454034, 1.500000000000001332 ) ) ;
#29115=ADVANCED_FACE ( 'NONE', ( #9583 ), #14419, .F. ) ;
#29119=ORIENTED_EDGE ( 'NONE', *, *, #8454, .T. ) ;
#29122=B_SPLINE_CURVE_WITH_KNOTS ( 'NONE', 3,
 ( #11395, #9195, #21175, #2483, #16674, #12000, #30699, #8902, #18425, #9049, #25884, #18707, #4515, #5127, #14640, #23984, #2957, #24611 ),
 .UNSPECIFIED., .F., .F.,
 ( 4, 2, 2, 2, 2, 2, 2, 2, 4 ),
 ( 0.000000000000000000, 0.0003967869494442914082, 0.0007935738988885828165, 0.001190360848332874116, 0.001587147797777165633, 0.001983934747221457150, 0.002380721696665748233, 0.002777508646110039749, 0.003174295595554331266 ),
 .UNSPECIFIED. ) ;
#29127=FACE_OUTER_BOUND ( 'NONE', #29458, .T. ) ;
#29129=CARTESIAN_POINT ( 'NONE',  ( 15.31102578509455903, 12.89549683364648835, 18.55820869691756769 ) ) ;
#29130=CARTESIAN_POINT ( 'NONE',  ( -10.81179434590808697, -16.84691785479785864, 7.595116371587256054 ) ) ;
#29132=B_SPLINE_CURVE_WITH_KNOTS ( 'NONE', 3,
 ( #30241, #25565, #20424, #8886, #29946, #8582, #23368, #27760, #10755, #18410, #15735, #20266, #4188, #25254, #3901, #23200, #6390, #22906, #1557, #11066 ),
 .UNSPECIFIED., .F., .F.,
 ( 4, 2, 2, 2, 2, 2, 2, 2, 2, 4 ),
 ( 0.000000000000000000, 0.06250000000000030531, 0.1250000000000006106, 0.1875000000000009159, 0.2187500000000009714, 0.2500000000000010547, 0.3125000000000007772, 0.3750000000000005551, 0.4375000000000002776, 0.5000000000000000000 ),
 .UNSPECIFIED. ) ;
#29133=CARTESIAN_POINT ( 'NONE',  ( -16.86183147812084115, 2.368508504629202260, 7.359006845440219102 ) ) ;
#29134=B_SPLINE_CURVE_WITH_KNOTS ( 'NONE', 3,
 ( #18223, #6056, #1388, #8567, #17605, #3566, #29615, #6372, #10905, #20406, #22579, #18071, #25400, #27588, #12770, #22272 ),
 .UNSPECIFIED., .F., .F.,
 ( 4, 2, 2, 2, 2, 2, 2, 4 ),
 ( 0.4999999999999997224, 0.6249999999999997780, 0.6874999999999997780, 0.7187499999999997780, 0.7499999999999997780, 0.8124999999999997780, 0.8749999999999997780, 1.000000000000000000 ),
 .UNSPECIFIED. ) ;
#29135=DIRECTION ( 'NONE',  ( 1.000000000000000000, 0.000000000000000000, 0.000000000000000000 ) ) ;
#29139=CIRCLE ( 'NONE', #24652, 0.7499999999999997780 ) ;
#29142=CARTESIAN_POINT ( 'NONE',  ( -6.737371319102178902, 18.84978071134531419, 18.73743063545763121 ) ) ;
#29143=CARTESIAN_POINT ( 'NONE',  ( 3.474270935886293987, -15.38174572367601911, -0.6213203435596476032 ) ) ;
#29144=AXIS2_PLACEMENT_3D ( 'NONE', #23904, #26713, #16895 ) ;
#29148=DIRECTION ( 'NONE',  ( -0.1423148382732853101, 0.9898214418809327952, 0.000000000000000000 ) ) ;
#29151=CARTESIAN_POINT ( 'NONE',  ( 10.38931136226422325, -17.11076273665786118, 7.176035686813569292 ) ) ;
#29156=DIRECTION ( 'NONE',  ( 0.7557495743542582689, -0.6548607339452849896, 0.000000000000000000 ) ) ;
#29159=CARTESIAN_POINT ( 'NONE',  ( -15.16517293421789070, -7.781889191988407894, 7.652108011868850923 ) ) ;
#29164=VECTOR ( 'NONE', #29925, 1000.000000000000000 ) ;
#29165=CARTESIAN_POINT ( 'NONE',  ( -17.64439154790314390, -9.416908767371243272, 19.85730954408918691 ) ) ;
#29166=CARTESIAN_POINT ( 'NONE',  ( 16.86235748570416249, 2.342382300094909553, 7.176035686813569292 ) ) ;
#29168=CARTESIAN_POINT ( 'NONE',  ( 15.51850634784529959, 12.64495090725178983, 6.310736198168394928 ) ) ;
#29169=ORIENTED_EDGE ( 'NONE', *, *, #5934, .T. ) ;
#29170=CARTESIAN_POINT ( 'NONE',  ( 16.13887868878510190, -5.569097860077081741, 7.196036389296800451 ) ) ;
#29171=DIRECTION ( 'NONE',  ( 1.000000000000000000, 0.000000000000000000, 0.000000000000000000 ) ) ;
#29178=LINE ( 'NONE', #17327, #6114 ) ;
#29183=CARTESIAN_POINT ( 'NONE',  ( 9.766261594859264150, -13.96654203752514256, 20.34789198813115263 ) ) ;
#29189=DIRECTION ( 'NONE',  ( 0.000000000000000000, 0.000000000000000000, 1.000000000000000000 ) ) ;
#29190=ORIENTED_EDGE ( 'NONE', *, *, #7636, .T. ) ;
#29201=CARTESIAN_POINT ( 'NONE',  ( -2.352830851074180440, -9.185733585337901630, 21.50000000000000000 ) ) ;
#29204=CIRCLE ( 'NONE', #7786, 0.7500000000000006661 ) ;
#29205=DIRECTION ( 'NONE',  ( 0.000000000000000000, 0.000000000000000000, 1.000000000000000000 ) ) ;
#29207=DIRECTION ( 'NONE',  ( 1.000000000000000000, 0.000000000000000000, 0.000000000000000000 ) ) ;
#29211=FACE_BOUND ( 'NONE', #27187, .T. ) ;
#29212=ORIENTED_EDGE ( 'NONE', *, *, #12004, .T. ) ;
#29223=ORIENTED_EDGE ( 'NONE', *, *, #8693, .F. ) ;
#29225=CIRCLE ( 'NONE', #18278, 9.482273699623480212 ) ;
#29227=CARTESIAN_POINT ( 'NONE',  ( -7.322557715923444732, 14.41080185948837311, -0.6213203435596476032 ) ) ;
#29228=LINE ( 'NONE', #14716, #3672 ) ;
#29229=ORIENTED_EDGE ( 'NONE', *, *, #25615, .F. ) ;
#29234=CARTESIAN_POINT ( 'NONE',  ( 10.23384659304339372, -13.64843352988230230, 5.749491821935610147 ) ) ;
#29235=EDGE_CURVE ( 'NONE', #17226, #4417, #7897, .T. ) ;
#29237=VECTOR ( 'NONE', #20927, 1000.000000000000000 ) ;
#29238=EDGE_LOOP ( 'NONE', ( #21513, #12993, #20087, #16435 ) ) ;
#29239=ORIENTED_EDGE ( 'NONE', *, *, #11905, .T. ) ;
#29242=CARTESIAN_POINT ( 'NONE',  ( -15.30875331599080091, 12.89789204219718854, 5.653912893140659257 ) ) ;
#29246=CARTESIAN_POINT ( 'NONE',  ( 16.19239463133111911, -5.428304825925631683, 19.21769074125273491 ) ) ;
#29247=CIRCLE ( 'NONE', #10314, 0.7499999999999997780 ) ;
#29253=DIRECTION ( 'NONE',  ( 1.000000000000000000, 0.000000000000000000, 0.000000000000000000 ) ) ;
#29254=EDGE_CURVE ( 'NONE', #4883, #8580, #22196, .T. ) ;
#29260=VECTOR ( 'NONE', #2209, 1000.000000000000000 ) ;
#29264=DIRECTION ( 'NONE',  ( -0.000000000000000000, 0.000000000000000000, -1.000000000000000000 ) ) ;
#29267=CYLINDRICAL_SURFACE ( 'NONE', #15295, 20.00000000000000355 ) ;
#29268=CARTESIAN_POINT ( 'NONE',  ( 16.01802636632491428, -5.877265577664587681, 5.759928666072748449 ) ) ;
#29273=AXIS2_PLACEMENT_3D ( 'NONE', #554, #12430, #28799 ) ;
#29275=DIRECTION ( 'NONE',  ( -0.000000000000000000, -0.000000000000000000, -1.000000000000000000 ) ) ;
#29276=CYLINDRICAL_SURFACE ( 'NONE', #9400, 9.482273699623480212 ) ;
#29281=ORIENTED_EDGE ( 'NONE', *, *, #26299, .T. ) ;
#29287=VERTEX_POINT ( 'NONE', #22650 ) ;
#29289=CARTESIAN_POINT ( 'NONE',  ( 15.41319392345653938, 12.77323265862689183, 18.71435384576123440 ) ) ;
#29291=CARTESIAN_POINT ( 'NONE',  ( 15.89967663190787839, -6.161197767010743398, 20.32367522806703874 ) ) ;
#29298=CARTESIAN_POINT ( 'NONE',  ( -17.20435420003449423, -1.463329469628170898, 24.50000000000000000 ) ) ;
#29299=ORIENTED_EDGE ( 'NONE', *, *, #1002, .T. ) ;
#29301=EDGE_LOOP ( 'NONE', ( #23772, #14273, #2832, #22403 ) ) ;
#29302=CARTESIAN_POINT ( 'NONE',  ( -6.908049759614255159, 18.76916546752685733, 19.61564845152807379 ) ) ;
#29305=B_SPLINE_SURFACE_WITH_KNOTS ( 'NONE', 3, 1, ( 
 ( #23061, #14280 ),
 ( #4773, #2451 ),
 ( #30825, #19439 ),
 ( #2280, #21139 ),
 ( #21619, #19281 ),
 ( #9472, #2758 ),
 ( #255, #21462 ),
 ( #410, #28349 ),
 ( #28804, #26002 ),
 ( #26622, #18833 ),
 ( #28956, #7441 ),
 ( #12271, #26464 ),
 ( #4631, #18988 ),
 ( #23799, #1711 ),
 ( #21773, #7130 ),
 ( #11800, #6975 ),
 ( #14129, #9622 ),
 ( #21306, #9928 ),
 ( #17095, #23635 ),
 ( #16641, #5249 ),
 ( #104, #11970 ),
 ( #11226, #19132 ),
 ( #28648, #7274 ),
 ( #4940, #24269 ),
 ( #19739, #2916 ),
 ( #3367, #12736 ),
 ( #7748, #17561 ),
 ( #26780, #27080 ),
 ( #5704, #17253 ),
 ( #29573, #17707 ),
 ( #10691, #24418 ) ),
 .UNSPECIFIED., .F., .F., .F.,
 ( 4, 3, 3, 3, 3, 3, 3, 3, 3, 3, 4 ),
 ( 2, 2 ),
 ( 0.000000000000000000, 0.05425176834609633791, 0.1085332949128352958, 0.1623767749169382768, 0.2157504826133063158, 0.2688657508888171455, 0.3218907763505476360, 0.3749548578363336993, 0.4282048033836242107, 0.4818374082110501444, 0.4999999999131651274 ),
 ( 0.000000000000000000, 1.000000000000000000 ),
 .UNSPECIFIED. ) ;
#29306=CARTESIAN_POINT ( 'NONE',  ( 19.61965483366450158, 3.971857776421113595, 7.280727868105637768 ) ) ;
#29307=CARTESIAN_POINT ( 'NONE',  ( -14.70245401545668962, 13.58508552794529400, 19.11611934778430921 ) ) ;
#29309=CARTESIAN_POINT ( 'NONE',  ( -8.481700458822087896, -14.78796854237962322, 18.34838970509067479 ) ) ;
#29314=CARTESIAN_POINT ( 'NONE',  ( 10.34995923732865286, -17.13460031806512873, 6.211014596808754007 ) ) ;
#29317=DIRECTION ( 'NONE',  ( 0.000000000000000000, 0.000000000000000000, 1.000000000000000000 ) ) ;
#29318=CARTESIAN_POINT ( 'NONE',  ( 19.86493687747363168, 2.320961355260795944, 7.156831654632821227 ) ) ;
#29319=VERTEX_POINT ( 'NONE', #29386 ) ;
#29320=ORIENTED_EDGE ( 'NONE', *, *, #25034, .T. ) ;
#29321=DIRECTION ( 'NONE',  ( -1.000000000000000000, 0.000000000000000000, 0.000000000000000000 ) ) ;
#29322=CARTESIAN_POINT ( 'NONE',  ( 18.70859934877967135, -7.070433808158456124, 19.61564845152809511 ) ) ;
#29323=ORIENTED_EDGE ( 'NONE', *, *, #8243, .T. ) ;
#29325=B_SPLINE_CURVE_WITH_KNOTS ( 'NONE', 3,
 ( #12079, #24068, #367, #21577, #14238, #26107, #28145, #6938, #16448, #6770, #4737, #21105, #16295, #25813, #23755, #23920, #2409, #21427 ),
 .UNSPECIFIED., .F., .F.,
 ( 4, 2, 2, 2, 2, 2, 2, 2, 4 ),
 ( 0.000000000000000000, 0.0003967869494442890772, 0.0007935738988885781544, 0.001190360848332867177, 0.001587147797777156309, 0.001983934747221445440, 0.002380721696665734355, 0.002777508646110023703, 0.003174295595554312618 ),
 .UNSPECIFIED. ) ;
#29327=DIRECTION ( 'NONE',  ( 1.000000000000000000, 0.000000000000000000, 0.000000000000000000 ) ) ;
#29331=CARTESIAN_POINT ( 'NONE',  ( -9.982956658368040692, -17.33059308371926122, 20.15039051365864253 ) ) ;
#29332=CARTESIAN_POINT ( 'NONE',  ( 14.25941570111287682, 14.04905143479254548, 6.233981582756856987 ) ) ;
#29333=CARTESIAN_POINT ( 'NONE',  ( 19.89797503522100541, 2.188012981718273853, 6.641371103590088865 ) ) ;
#29337=CARTESIAN_POINT ( 'NONE',  ( -13.71169828459619389, 10.15410312392310033, 20.24143955528809613 ) ) ;
#29340=CARTESIAN_POINT ( 'NONE',  ( -10.51513057463695411, -17.01270198993486460, 20.34789198813115263 ) ) ;
#29342=DIRECTION ( 'NONE',  ( -0.000000000000000000, -0.000000000000000000, -1.000000000000000000 ) ) ;
#29355=CARTESIAN_POINT ( 'NONE',  ( -15.81542570303655637, 12.27127866024201985, 18.64703902303423178 ) ) ;
#29361=CARTESIAN_POINT ( 'NONE',  ( -6.187077094091591789, 11.47693674426096955, 1.500000000000001332 ) ) ;
#29362=DIRECTION ( 'NONE',  ( 1.000000000000000000, 0.000000000000000000, 0.000000000000000000 ) ) ;
#29364=VECTOR ( 'NONE', #11707, 1000.000000000000000 ) ;
#29367=CARTESIAN_POINT ( 'NONE',  ( 19.56075217167572688, 4.168887357664727844, 6.392525840300342210 ) ) ;
#29373=ORIENTED_EDGE ( 'NONE', *, *, #1783, .F. ) ;
#29374=DIRECTION ( 'NONE',  ( 0.9096319953545183301, 0.4154150130018865461, 0.000000000000000000 ) ) ;
#29376=ORIENTED_EDGE ( 'NONE', *, *, #16255, .T. ) ;
#29385=EDGE_CURVE ( 'NONE', #10771, #24660, #15168, .T. ) ;
#29386=CARTESIAN_POINT ( 'NONE',  ( 3.896869771148438577, -16.82098518409776489, 24.50000000000000000 ) ) ;
#29388=DIRECTION ( 'NONE',  ( -0.000000000000000000, -0.000000000000000000, 1.000000000000000000 ) ) ;
#29390=ORIENTED_EDGE ( 'NONE', *, *, #11644, .T. ) ;
#29391=AXIS2_PLACEMENT_3D ( 'NONE', #536, #7883, #26601 ) ;
#29392=CARTESIAN_POINT ( 'NONE',  ( -11.35279153858833290, -16.48728705952963480, 19.56050940960062690 ) ) ;
#29393=CARTESIAN_POINT ( 'NONE',  ( -17.96415918337694251, -8.831719996762307900, 7.627891251804737927 ) ) ;
#29394=CARTESIAN_POINT ( 'NONE',  ( -6.587417658830999834, 18.90298706665743822, 5.872146474157316831 ) ) ;
#29396=CARTESIAN_POINT ( 'NONE',  ( 1.000000000000008438, 15.73749217771910125, 1.500000000000001332 ) ) ;
#29397=DIRECTION ( 'NONE',  ( 0.6548607339452782172, -0.7557495743542642641, 0.000000000000000000 ) ) ;
#29398=VERTEX_POINT ( 'NONE', #17525 ) ;
#29401=CARTESIAN_POINT ( 'NONE',  ( -5.196396160405778453, 19.31337320890706266, 19.96302680909623462 ) ) ;
#29403=CARTESIAN_POINT ( 'NONE',  ( 15.41296542101254552, 5.939519782021115191, -0.6213203435596476032 ) ) ;
#29404=EDGE_CURVE ( 'NONE', #28377, #7591, #24857, .T. ) ;
#29405=CARTESIAN_POINT ( 'NONE',  ( 0.1595703638607181285, -17.02896808597062162, 7.453286057244485008 ) ) ;
#29409=CARTESIAN_POINT ( 'NONE',  ( -11.40980092660686829, 6.310027164379044429, 1.500000000000001332 ) ) ;
#29413=CARTESIAN_POINT ( 'NONE',  ( 5.298970182598334411, 19.30368537022594211, 18.34798005862930026 ) ) ;
#29419=EDGE_CURVE ( 'NONE', #10573, #357, #12139, .T. ) ;
#29420=DIRECTION ( 'NONE',  ( 0.000000000000000000, 0.000000000000000000, -1.000000000000000000 ) ) ;
#29421=ADVANCED_FACE ( 'NONE', ( #21855 ), #21219, .F. ) ;
#29423=DIRECTION ( 'NONE',  ( -0.000000000000000000, -0.000000000000000000, 1.000000000000000000 ) ) ;
#29424=ORIENTED_EDGE ( 'NONE', *, *, #13176, .F. ) ;
#29426=CARTESIAN_POINT ( 'NONE',  ( 12.53355205340454681, 11.54212474482388195, 20.32222155561919408 ) ) ;
#29429=AXIS2_PLACEMENT_3D ( 'NONE', #9647, #16820, #14476 ) ;
#29437=CARTESIAN_POINT ( 'NONE',  ( 4.434078574240013282, 19.50234843602376955, 6.149077423860704883 ) ) ;
#29441=ADVANCED_FACE ( 'NONE', ( #26540 ), #17018, .F. ) ;
#29445=CARTESIAN_POINT ( 'NONE',  ( 12.38084545251366642, 11.71426794001388316, 18.34777357837152323 ) ) ;
#29448=DIRECTION ( 'NONE',  ( 1.000000000000000000, 0.000000000000000000, 0.000000000000000000 ) ) ;
#29450=CARTESIAN_POINT ( 'NONE',  ( 18.33793066653144521, -7.982499537706466697, 5.652196082369965069 ) ) ;
#29455=DIRECTION ( 'NONE',  ( -0.000000000000000000, -0.000000000000000000, 1.000000000000000000 ) ) ;
#29458=EDGE_LOOP ( 'NONE', ( #20017, #20185, #21488, #30674 ) ) ;
#29462=CARTESIAN_POINT ( 'NONE',  ( 19.60578376704636483, 4.040313317649105507, 7.196036389296800451 ) ) ;
#29463=CARTESIAN_POINT ( 'NONE',  ( -15.28428954155913289, 12.92682542062231121, 18.35377592296120497 ) ) ;
#29469=EDGE_CURVE ( 'NONE', #17832, #14781, #4550, .T. ) ;
#29470=CARTESIAN_POINT ( 'NONE',  ( 9.186411229153641500, -14.33460949872162260, 7.272049892295485485 ) ) ;
#29473=VECTOR ( 'NONE', #1461, 1000.000000000000000 ) ;
#29474=DIRECTION ( 'NONE',  ( 0.2817325568414296710, -0.9594929736144973687, 0.000000000000000000 ) ) ;
#29476=ORIENTED_EDGE ( 'NONE', *, *, #9431, .T. ) ;
#29477=CARTESIAN_POINT ( 'NONE',  ( 18.28362707703099233, -8.107168301167737567, 20.34789198813115618 ) ) ;
#29479=LINE ( 'NONE', #19341, #8384 ) ;
#29480=ORIENTED_EDGE ( 'NONE', *, *, #29543, .T. ) ;
#29485=AXIS2_PLACEMENT_3D ( 'NONE', #30701, #14484, #26351 ) ;
#29487=CARTESIAN_POINT ( 'NONE',  ( 14.59199839715917513, 13.70371665158259766, 5.749491821935610147 ) ) ;
#29488=CARTESIAN_POINT ( 'NONE',  ( 16.84421249428844192, 2.491431357970654403, 5.940635272151477686 ) ) ;
#29491=ORIENTED_EDGE ( 'NONE', *, *, #29469, .F. ) ;
#29494=CIRCLE ( 'NONE', #6579, 9.482273699623480212 ) ;
#29496=CARTESIAN_POINT ( 'NONE',  ( 3.122919890997790215, 16.78802993858288772, 6.995624166085161910 ) ) ;
#29498=DIRECTION ( 'NONE',  ( 1.000000000000000000, 0.000000000000000000, 0.000000000000000000 ) ) ;
#29501=CARTESIAN_POINT ( 'NONE',  ( 10.25620417238948257, -17.19090129355371488, 19.33715507985239412 ) ) ;
#29506=CARTESIAN_POINT ( 'NONE',  ( -15.94999985682714971, 12.09556989559485629, 19.69140814234746273 ) ) ;
#29511=DIRECTION ( 'NONE',  ( 0.000000000000000000, 0.000000000000000000, 1.000000000000000000 ) ) ;
#29519=ORIENTED_EDGE ( 'NONE', *, *, #5159, .F. ) ;
#29527=CARTESIAN_POINT ( 'NONE',  ( -9.471281197126605989, -0.4564504349074081091, 13.00000000000000178 ) ) ;
#29528=AXIS2_PLACEMENT_3D ( 'NONE', #19787, #29317, #19954 ) ;
#29530=CARTESIAN_POINT ( 'NONE',  ( 0.7836603915001300047, -17.02734626464551226, 18.34798005862930381 ) ) ;
#29533=CARTESIAN_POINT ( 'NONE',  ( 12.86767874445214055, -1.850092897552706894, 24.50000000000000000 ) ) ;
#29536=CARTESIAN_POINT ( 'NONE',  ( 14.67322144252663918, 13.61684651386558542, 20.29915277494337644 ) ) ;
#29537=CARTESIAN_POINT ( 'NONE',  ( -16.46198811862381817, -1.356593340923033075, -0.6213203435596476032 ) ) ;
#29539=CARTESIAN_POINT ( 'NONE',  ( -11.35443157991641172, -16.48616348260577524, 19.11611934778430921 ) ) ;
#29541=CARTESIAN_POINT ( 'NONE',  ( -6.116198564155505224, 19.06064343544019835, 7.643931100913408550 ) ) ;
#29543=EDGE_CURVE ( 'NONE', #17560, #22179, #24345, .T. ) ;
#29544=CARTESIAN_POINT ( 'NONE',  ( 10.30429258806635495, -13.59853737800767881, 7.500147780736496017 ) ) ;
#29545=EDGE_CURVE ( 'NONE', #20124, #7938, #7919, .T. ) ;
#29553=CARTESIAN_POINT ( 'NONE',  ( -12.86036580545043684, 11.15762522838069337, 6.018569869498933578 ) ) ;
#29559=VERTEX_POINT ( 'NONE', #20134 ) ;
#29561=B_SPLINE_SURFACE_WITH_KNOTS ( 'NONE', 3, 1, ( 
 ( #20094, #10899 ),
 ( #18069, #15563 ),
 ( #15235, #24928 ),
 ( #17920, #1230 ),
 ( #3244, #29612 ),
 ( #3725, #22114 ),
 ( #3409, #29766 ),
 ( #3879, #12768 ),
 ( #22428, #20404 ),
 ( #10732, #22728 ),
 ( #10430, #5902 ),
 ( #8408, #8245 ),
 ( #27585, #26974 ),
 ( #13240, #6211 ),
 ( #24763, #741 ),
 ( #15714, #17751 ),
 ( #20242, #22269 ),
 ( #1385, #10260 ),
 ( #19774, #27271 ),
 ( #913, #5598 ),
 ( #29462, #15093 ),
 ( #29306, #7947 ),
 ( #17452, #15403 ),
 ( #5743, #8096 ),
 ( #1072, #10582 ),
 ( #3564, #27120 ),
 ( #13087, #25399 ),
 ( #20997, #9161 ),
 ( #4170, #8709 ),
 ( #23184, #20549 ),
 ( #9311, #15883 ) ),
 .UNSPECIFIED., .F., .F., .F.,
 ( 4, 3, 3, 3, 3, 3, 3, 3, 3, 3, 4 ),
 ( 2, 2 ),
 ( 0.4999999998345681651, 0.5360336730431942698, 0.5907651151589017324, 0.6456034593241839481, 0.6998270958050443191, 0.7529536536315944995, 0.8052385063053264513, 0.8575343587103996246, 0.9106564858195047574, 0.9648414833209688624, 1.000000006602610014 ),
 ( 0.000000000000000000, 1.000000000000000000 ),
 .UNSPECIFIED. ) ;
#29566=CARTESIAN_POINT ( 'NONE',  ( 11.11118388262826251, -16.62953976291647962, 5.652196082369964181 ) ) ;
#29569=LINE ( 'NONE', #866, #23985 ) ;
#29571=CYLINDRICAL_SURFACE ( 'NONE', #12855, 20.00000000000000000 ) ;
#29572=VERTEX_POINT ( 'NONE', #7820 ) ;
#29573=CARTESIAN_POINT ( 'NONE',  ( -18.07538971572904174, -8.601943808150394943, 5.651989602109218858 ) ) ;
#29576=EDGE_CURVE ( 'NONE', #17226, #10643, #5418, .T. ) ;
#29577=CYLINDRICAL_SURFACE ( 'NONE', #28212, 0.7500000000000006661 ) ;
#29579=FACE_OUTER_BOUND ( 'NONE', #26426, .T. ) ;
#29584=DIRECTION ( 'NONE',  ( 1.000000000000000000, 0.000000000000000000, 0.000000000000000000 ) ) ;
#29585=CARTESIAN_POINT ( 'NONE',  ( 4.335955696074043075, 19.52440042691175393, 6.919864475265786297 ) ) ;
#29592=CIRCLE ( 'NONE', #16137, 9.482273699623480212 ) ;
#29593=FACE_OUTER_BOUND ( 'NONE', #18900, .T. ) ;
#29595=CARTESIAN_POINT ( 'NONE',  ( 15.54774248266353176, 12.60889669900781129, 19.22654678686458141 ) ) ;
#29598=VERTEX_POINT ( 'NONE', #20727 ) ;
#29599=CARTESIAN_POINT ( 'NONE',  ( 15.87141697993282463, -6.228091237695521976, 20.33971507717571114 ) ) ;
#29600=CARTESIAN_POINT ( 'NONE',  ( 18.23136487193859523, -8.223889151412006271, 5.676722608126685721 ) ) ;
#29603=CARTESIAN_POINT ( 'NONE',  ( 11.40980092660686118, 6.310027164379057751, 24.50000000000000000 ) ) ;
#29604=ORIENTED_EDGE ( 'NONE', *, *, #20952, .T. ) ;
#29608=EDGE_CURVE ( 'NONE', #22425, #4518, #30258, .T. ) ;
#29610=EDGE_CURVE ( 'NONE', #12232, #10944, #15996, .T. ) ;
#29612=CARTESIAN_POINT ( 'NONE',  ( 16.68596330270456818, 3.532048315275338357, 5.704143890883081269 ) ) ;
#29615=CARTESIAN_POINT ( 'NONE',  ( 1.762690206872143728, -16.98588469933382683, 6.392658652357122051 ) ) ;
#29621=CARTESIAN_POINT ( 'NONE',  ( 11.39819190923272529, -16.45610177916888262, 18.39992786714538298 ) ) ;
#29625=CARTESIAN_POINT ( 'NONE',  ( 17.90972305382299368, -8.901787470106558686, 19.47728749465736797 ) ) ;
#29634=CARTESIAN_POINT ( 'NONE',  ( 5.888181818956391034, 19.11381997051147152, 5.849008070840538309 ) ) ;
#29637=CARTESIAN_POINT ( 'NONE',  ( 14.20930976959225411, 14.09970620734104330, 6.447548852708279377 ) ) ;
#29645=CARTESIAN_POINT ( 'NONE',  ( -8.824744466605359605, -8.513189541288717521, 1.500000000000001332 ) ) ;
#29650=CYLINDRICAL_SURFACE ( 'NONE', #7361, 9.482273699623480212 ) ;
#29651=DIRECTION ( 'NONE',  ( -1.000000000000000000, 0.000000000000000000, 0.000000000000000000 ) ) ;
#29652=CARTESIAN_POINT ( 'NONE',  ( 11.11463893384431323, -16.64861865631835158, 20.34789198813115263 ) ) ;
#29653=CARTESIAN_POINT ( 'NONE',  ( 16.85539258114950556, 2.401441585233817566, 19.96783386855779341 ) ) ;
#29654=ORIENTED_EDGE ( 'NONE', *, *, #8669, .F. ) ;
#29656=CARTESIAN_POINT ( 'NONE',  ( 17.93514094173302453, -8.890850898656898593, 6.864725433338323413 ) ) ;
#29657=CARTESIAN_POINT ( 'NONE',  ( -15.93537878762122872, 12.11488692681953694, 18.92976555901915603 ) ) ;
#29660=ORIENTED_EDGE ( 'NONE', *, *, #836, .F. ) ;
#29673=VERTEX_POINT ( 'NONE', #14424 ) ;
#29676=DIRECTION ( 'NONE',  ( 0.000000000000000000, 0.000000000000000000, -1.000000000000000000 ) ) ;
#29680=EDGE_CURVE ( 'NONE', #24939, #23193, #25340, .T. ) ;
#29683=DIRECTION ( 'NONE',  ( 0.9096319953545185522, -0.4154150130018859910, -0.000000000000000000 ) ) ;
#29686=CARTESIAN_POINT ( 'NONE',  ( -10.94076559809103699, -16.74260033555411553, 5.775318986477953942 ) ) ;
#29688=CARTESIAN_POINT ( 'NONE',  ( 0.5064538767941907382, -20.01148730445865098, 5.661398277488801867 ) ) ;
#29692=CARTESIAN_POINT ( 'NONE',  ( -4.623640074070403116, 16.38233772743116390, 6.973843882838226094 ) ) ;
#29696=CIRCLE ( 'NONE', #2277, 0.7500000000000006661 ) ;
#29699=ORIENTED_EDGE ( 'NONE', *, *, #7531, .F. ) ;
#29700=APPLICATION_CONTEXT ( 'automotive_design' ) ;
#29704=DIRECTION ( 'NONE',  ( -1.000000000000000000, 0.000000000000000000, 0.000000000000000000 ) ) ;
#29713=CARTESIAN_POINT ( 'NONE',  ( 19.65528207207771061, 3.699272045506084350, 18.47531940416305929 ) ) ;
#29715=CARTESIAN_POINT ( 'NONE',  ( 11.93908819109400099, -16.04550321516296663, 6.523620417364445423 ) ) ;
#29716=AXIS2_PLACEMENT_3D ( 'NONE', #22398, #22237, #8370 ) ;
#29717=LINE ( 'NONE', #22533, #12054 ) ;
#29720=DIRECTION ( 'NONE',  ( -0.4154150130018840481, 0.9096319953545194403, 0.000000000000000000 ) ) ;
#29722=DIRECTION ( 'NONE',  ( 0.000000000000000000, 0.000000000000000000, -1.000000000000000000 ) ) ;
#29728=AXIS2_PLACEMENT_3D ( 'NONE', #9473, #26146, #23801 ) ;
#29729=DIRECTION ( 'NONE',  ( -0.000000000000000000, -0.000000000000000000, -1.000000000000000000 ) ) ;
#29742=AXIS2_PLACEMENT_3D ( 'NONE', #17068, #18961, #5374 ) ;
#29748=CARTESIAN_POINT ( 'NONE',  ( 18.35115018089978633, -7.996680568998191241, 20.34789198813115263 ) ) ;
#29749=DIRECTION ( 'NONE',  ( -0.000000000000000000, -0.000000000000000000, 1.000000000000000000 ) ) ;
#29755=CARTESIAN_POINT ( 'NONE',  ( -4.600690885580802636, 16.38836304891080786, 19.08155846658118904 ) ) ;
#29760=CARTESIAN_POINT ( 'NONE',  ( -16.81926493917334042, 2.618766740937769288, 19.60617949693493500 ) ) ;
#29762=ORIENTED_EDGE ( 'NONE', *, *, #21763, .F. ) ;
#29763=CARTESIAN_POINT ( 'NONE',  ( -6.560142022084716196, 18.89374015187015843, 20.15039051365864253 ) ) ;
#29766=CARTESIAN_POINT ( 'NONE',  ( 16.64821571380338838, 3.734651121118246042, 5.810767894563978686 ) ) ;
#29773=CARTESIAN_POINT ( 'NONE',  ( -17.06238204535245018, 0.6919203014575876498, 19.02573955821369012 ) ) ;
#29774=CARTESIAN_POINT ( 'NONE',  ( -17.03551135121415783, 1.010186107319478888, 18.56793045041961321 ) ) ;
#29775=LINE ( 'NONE', #27592, #23305 ) ;
#29780=CARTESIAN_POINT ( 'NONE',  ( 11.90564931213029531, -16.09225693709295513, 19.03762469184452755 ) ) ;
#29786=CARTESIAN_POINT ( 'NONE',  ( 0.000000000000000000, 13.00000000000001421, 24.50000000000000000 ) ) ;
#29787=CARTESIAN_POINT ( 'NONE',  ( -4.619434794156391355, 16.38343285047924880, 6.974106381145714018 ) ) ;
#29789=DIRECTION ( 'NONE',  ( 1.000000000000000000, 0.000000000000000000, 0.000000000000000000 ) ) ;
#29790=CIRCLE ( 'NONE', #21802, 20.00000000000000000 ) ;
#29794=CARTESIAN_POINT ( 'NONE',  ( -1.000000000000008438, 13.00000000000001421, 24.50000000000000000 ) ) ;
#29795=ORIENTED_EDGE ( 'NONE', *, *, #23266, .F. ) ;
#29797=ADVANCED_FACE ( 'NONE', ( #26592 ), #17419, .T. ) ;
#29799=CARTESIAN_POINT ( 'NONE',  ( 12.12755608862869039, 11.99246096336393030, 5.704143890883081269 ) ) ;
#29800=CARTESIAN_POINT ( 'NONE',  ( 19.81227057857146434, 2.861376016183142745, 7.595116371587256054 ) ) ;
#29801=EDGE_LOOP ( 'NONE', ( #20827, #10602, #16899, #16316 ) ) ;
#29802=CARTESIAN_POINT ( 'NONE',  ( 12.71123406193363437, 11.33589958720537005, 5.796888747622817029 ) ) ;
#29807=CIRCLE ( 'NONE', #10360, 20.00000000000000000 ) ;
#29811=EDGE_CURVE ( 'NONE', #19771, #12217, #11818, .T. ) ;
#29812=EDGE_CURVE ( 'NONE', #12979, #23779, #6556, .T. ) ;
#29813=CARTESIAN_POINT ( 'NONE',  ( 3.269395338272006235, 16.75466097144276745, 6.041646659195333058 ) ) ;
#29819=CARTESIAN_POINT ( 'NONE',  ( 16.87938398529692918, 2.193321724558643382, 19.45164628100866722 ) ) ;
#29820=ORIENTED_EDGE ( 'NONE', *, *, #23991, .F. ) ;
#29822=CARTESIAN_POINT ( 'NONE',  ( 15.51722275458702960, -7.010743380608710495, 5.940635272151477686 ) ) ;
#29823=CARTESIAN_POINT ( 'NONE',  ( -15.75339717617904611, 12.35099711776840792, 20.13759033520874908 ) ) ;
#29826=ORIENTED_EDGE ( 'NONE', *, *, #29404, .T. ) ;
#29828=CARTESIAN_POINT ( 'NONE',  ( 1.224038712338732404, -19.98030457043140018, 6.131018562779544823 ) ) ;
#29829=ADVANCED_FACE ( 'NONE', ( #30058 ), #28019, .F. ) ;
#29830=B_SPLINE_SURFACE_WITH_KNOTS ( 'NONE', 3, 1, ( 
 ( #7975, #17478 ),
 ( #5772, #27458 ),
 ( #8443, #10291 ),
 ( #29800, #7802 ),
 ( #21990, #20120 ),
 ( #943, #1254 ),
 ( #15266, #24797 ),
 ( #3436, #12957 ),
 ( #26847, #27301 ),
 ( #5932, #29166 ),
 ( #12651, #8272 ),
 ( #10455, #15121 ),
 ( #22450, #15588 ),
 ( #17629, #24638 ),
 ( #29333, #1098 ),
 ( #22299, #22143 ),
 ( #10609, #27000 ),
 ( #19969, #3271 ),
 ( #12800, #3128 ),
 ( #2979, #15429 ),
 ( #17786, #5470 ),
 ( #24951, #29488 ),
 ( #13112, #8123 ),
 ( #27146, #22603 ),
 ( #10761, #14971 ),
 ( #20272, #17948 ),
 ( #6078, #12496 ),
 ( #621, #10138 ),
 ( #19644, #17315 ),
 ( #24484, #20878 ),
 ( #30245, #6234 ) ),
 .UNSPECIFIED., .F., .F., .F.,
 ( 4, 3, 3, 3, 3, 3, 3, 3, 3, 3, 4 ),
 ( 2, 2 ),
 ( 0.000000000000000000, 0.05425176834609633791, 0.1085332949128352958, 0.1623767749169382768, 0.2157504826133063158, 0.2688657508888171455, 0.3218907763505476360, 0.3749548578363336993, 0.4282048033836242107, 0.4818374082110501444, 0.4999999999131654604 ),
 ( 0.000000000000000000, 1.000000000000000000 ),
 .UNSPECIFIED. ) ;
#29831=CARTESIAN_POINT ( 'NONE',  ( 12.44336852755150424, 11.64466880993055398, 5.651492010659111109 ) ) ;
#29833=VECTOR ( 'NONE', #27997, 1000.000000000000000 ) ;
#29837=FACE_OUTER_BOUND ( 'NONE', #24793, .T. ) ;
#29838=EDGE_CURVE ( 'NONE', #20491, #28528, #24917, .T. ) ;
#29839=CARTESIAN_POINT ( 'NONE',  ( 16.85625572096651226, 2.395390699250522726, 7.267659094423557953 ) ) ;
#29841=DIRECTION ( 'NONE',  ( 1.000000000000000000, 0.000000000000000000, 0.000000000000000000 ) ) ;
#29848=CARTESIAN_POINT ( 'NONE',  ( -19.92877566111874899, 1.688993080932616353, 18.73377938172347612 ) ) ;
#29849=ORIENTED_EDGE ( 'NONE', *, *, #8671, .T. ) ;
#29852=DIRECTION ( 'NONE',  ( -0.4154150130018840481, 0.9096319953545194403, 0.000000000000000000 ) ) ;
#29863=CARTESIAN_POINT ( 'NONE',  ( -9.213835811784830909, -14.31736145455815290, 18.71435384576123440 ) ) ;
#29866=CARTESIAN_POINT ( 'NONE',  ( 11.18191171624325797, -16.60365183919259380, 5.652605728828375753 ) ) ;
#29869=VECTOR ( 'NONE', #29676, 1000.000000000000000 ) ;
#29872=ORIENTED_EDGE ( 'NONE', *, *, #12436, .T. ) ;
#29875=CARTESIAN_POINT ( 'NONE',  ( -15.00589365688690435, 13.24944937571967429, 5.796888747622817029 ) ) ;
#29880=CARTESIAN_POINT ( 'NONE',  ( -10.62006778255435435, -16.96839658127461803, 5.657991946698900598 ) ) ;
#29885=VERTEX_POINT ( 'NONE', #20228 ) ;
#29886=CARTESIAN_POINT ( 'NONE',  ( 0.000000000000000000, 0.000000000000000000, 1.500000000000001332 ) ) ;
#29887=CARTESIAN_POINT ( 'NONE',  ( -8.416592248870403026, -14.82768166143396726, 5.661398277488802755 ) ) ;
#29891=DIRECTION ( 'NONE',  ( 0.000000000000000000, 0.000000000000000000, 1.000000000000000000 ) ) ;
#29897=CARTESIAN_POINT ( 'NONE',  ( -8.478038329015333829, 15.04174200911163517, 1.500000000000000000 ) ) ;
#29899=CARTESIAN_POINT ( 'NONE',  ( 19.83281414115337782, 2.582324728781452361, 7.454139397117725885 ) ) ;
#29904=ORIENTED_EDGE ( 'NONE', *, *, #26145, .T. ) ;
#29907=DIRECTION ( 'NONE',  ( 0.000000000000000000, 0.000000000000000000, -1.000000000000000000 ) ) ;
#29911=CARTESIAN_POINT ( 'NONE',  ( 9.644751206715060476, -14.04611738690534573, 18.37259980046033903 ) ) ;
#29913=ORIENTED_EDGE ( 'NONE', *, *, #7744, .T. ) ;
#29914=CARTESIAN_POINT ( 'NONE',  ( -11.25470158702820811, -16.53282404628956925, 19.85261563089511583 ) ) ;
#29916=CARTESIAN_POINT ( 'NONE',  ( -8.611567383417474630, -14.70762963579928417, 18.34969686940295830 ) ) ;
#29923=CARTESIAN_POINT ( 'NONE',  ( -16.83567995170645304, 2.524450606588025448, 19.85270094495841775 ) ) ;
#29925=DIRECTION ( 'NONE',  ( -0.8412535328311884220, -0.5406408174555862312, 0.000000000000000000 ) ) ;
#29926=DIRECTION ( 'NONE',  ( 0.000000000000000000, 0.000000000000000000, -1.000000000000000000 ) ) ;
#29927=DIRECTION ( 'NONE',  ( -1.000000000000000000, 0.000000000000000000, 0.000000000000000000 ) ) ;
#29928=CARTESIAN_POINT ( 'NONE',  ( -12.91351154505913179, 11.09846585523631823, 18.63641924841378028 ) ) ;
#29929=CARTESIAN_POINT ( 'NONE',  ( -9.846411740200890605, -17.42855948811279276, 19.97651184436794125 ) ) ;
#29931=CARTESIAN_POINT ( 'NONE',  ( -17.06630883447662583, 0.6398751886020307422, 19.28454053338348473 ) ) ;
#29932=CARTESIAN_POINT ( 'NONE',  ( -16.98411243466783560, 1.496360031252971456, 18.35718225375110180 ) ) ;
#29933=DIRECTION ( 'NONE',  ( -1.000000000000000000, 0.000000000000000000, 0.000000000000000000 ) ) ;
#29934=VERTEX_POINT ( 'NONE', #28492 ) ;
#29936=CARTESIAN_POINT ( 'NONE',  ( 10.16054539467770113, 13.96046037420044961, -0.6213203435596476032 ) ) ;
#29937=ORIENTED_EDGE ( 'NONE', *, *, #15246, .T. ) ;
#29940=ADVANCED_FACE ( 'NONE', ( #16631 ), #9758, .F. ) ;
#29941=AXIS2_PLACEMENT_3D ( 'NONE', #18338, #11006, #1791 ) ;
#29942=CARTESIAN_POINT ( 'NONE',  ( -5.557658336892894901, 19.23087281213772570, 5.749228751562096562 ) ) ;
#29943=ORIENTED_EDGE ( 'NONE', *, *, #26687, .F. ) ;
#29944=CARTESIAN_POINT ( 'NONE',  ( 5.291489565152560637, 19.28730510418394317, 5.652196082369965069 ) ) ;
#29945=VECTOR ( 'NONE', #18841, 1000.000000000000000 ) ;
#29946=CARTESIAN_POINT ( 'NONE',  ( -12.97413174825823390, 11.03100730454233336, 7.453286057244485008 ) ) ;
#29948=EDGE_LOOP ( 'NONE', ( #19890, #16657 ) ) ;
#29950=CARTESIAN_POINT ( 'NONE',  ( 11.91933518721470264, 12.21304923692660971, 5.872146474157316831 ) ) ;
#29953=EDGE_CURVE ( 'NONE', #15672, #29287, #23482, .T. ) ;
#29957=ORIENTED_EDGE ( 'NONE', *, *, #13184, .F. ) ;
#29958=ORIENTED_EDGE ( 'NONE', *, *, #12043, .T. ) ;
#29961=CIRCLE ( 'NONE', #8055, 0.7500000000000006661 ) ;
#29963=CARTESIAN_POINT ( 'NONE',  ( 19.81227057857146434, 2.861376016183142745, 20.29090034784956131 ) ) ;
#29968=CARTESIAN_POINT ( 'NONE',  ( 0.3567147238643519902, -19.99681861211371370, 18.34798005863226678 ) ) ;
#29969=CARTESIAN_POINT ( 'NONE',  ( -15.45532977000708108, 12.72198496171735371, 5.661398277488802755 ) ) ;
#29970=CARTESIAN_POINT ( 'NONE',  ( 4.606472074292930152, 19.48056636435423528, 20.06253562465620632 ) ) ;
#29971=ORIENTED_EDGE ( 'NONE', *, *, #21784, .F. ) ;
#29972=VERTEX_POINT ( 'NONE', #4621 ) ;
#29977=CARTESIAN_POINT ( 'NONE',  ( -5.010690217951877301, 19.38064900392119583, 19.22654678686458141 ) ) ;
#29978=DIRECTION ( 'NONE',  ( 1.000000000000000000, 0.000000000000000000, 0.000000000000000000 ) ) ;
#29979=EDGE_CURVE ( 'NONE', #10914, #19423, #28341, .T. ) ;
#29988=ORIENTED_EDGE ( 'NONE', *, *, #4449, .T. ) ;
#29989=EDGE_CURVE ( 'NONE', #11886, #11902, #26135, .T. ) ;
#29990=ORIENTED_EDGE ( 'NONE', *, *, #13036, .T. ) ;
#29994=CARTESIAN_POINT ( 'NONE',  ( -9.436481611552759219, -0.9307681286968215728, 13.00000000000000178 ) ) ;
#29997=CARTESIAN_POINT ( 'NONE',  ( 1.000000000000008438, 13.00000000000001421, 24.50000000000000000 ) ) ;
#30000=CARTESIAN_POINT ( 'NONE',  ( 0.8870900849372825858, -19.99803318816114484, 7.500147780736496017 ) ) ;
#30001=CARTESIAN_POINT ( 'NONE',  ( -16.81371235015666699, 2.650171115930315846, 6.714907520933426355 ) ) ;
#30004=ADVANCED_FACE ( 'NONE', ( #97 ), #28640, .F. ) ;
#30008=CARTESIAN_POINT ( 'NONE',  ( -5.686690470302443678, 16.07334902597871817, 7.643931100913408550 ) ) ;
#30009=CARTESIAN_POINT ( 'NONE',  ( 9.984725267469517718, -13.82013960671583241, 7.643931100913408550 ) ) ;
#30018=VECTOR ( 'NONE', #12096, 1000.000000000000000 ) ;
#30019=VERTEX_POINT ( 'NONE', #17086 ) ;
#30022=CARTESIAN_POINT ( 'NONE',  ( -11.24862133554823274, -16.55851774953666222, 7.176035686813569292 ) ) ;
#30024=DIRECTION ( 'NONE',  ( 0.000000000000000000, 0.000000000000000000, 1.000000000000000000 ) ) ;
#30025=CARTESIAN_POINT ( 'NONE',  ( 19.55517958221000185, 4.194633687229719854, 19.21940439362674624 ) ) ;
#30029=EDGE_CURVE ( 'NONE', #12655, #4949, #12342, .T. ) ;
#30032=CARTESIAN_POINT ( 'NONE',  ( 2.703030265324084080, -12.75514121382991384, 24.50000000000000000 ) ) ;
#30033=AXIS2_PLACEMENT_3D ( 'NONE', #3029, #22500, #13009 ) ;
#30034=CARTESIAN_POINT ( 'NONE',  ( 16.70031948179167003, 3.459335817989516393, 5.653604225791663218 ) ) ;
#30037=CARTESIAN_POINT ( 'NONE',  ( -17.05632420042165265, 0.7692048344871257326, 6.147510495896842286 ) ) ;
#30041=CARTESIAN_POINT ( 'NONE',  ( 19.87632233081031075, 2.221350112303686952, 6.386539667786102825 ) ) ;
#30044=ORIENTED_EDGE ( 'NONE', *, *, #8031, .F. ) ;
#30046=CARTESIAN_POINT ( 'NONE',  ( 0.000000000000000000, 0.000000000000000000, 1.500000000000001332 ) ) ;
#30048=DIRECTION ( 'NONE',  ( 0.000000000000000000, 0.000000000000000000, 1.000000000000000000 ) ) ;
#30050=CARTESIAN_POINT ( 'NONE',  ( -10.47960520055065636, -7.757439966934454034, 1.500000000000001332 ) ) ;
#30051=CARTESIAN_POINT ( 'NONE',  ( 11.82521593960875173, 5.400395169024529984, 24.50000000000000000 ) ) ;
#30055=AXIS2_PLACEMENT_3D ( 'NONE', #17772, #27138, #20423 ) ;
#30056=CARTESIAN_POINT ( 'NONE',  ( -16.81358047026921199, 2.650995224496061731, 6.755862304746362845 ) ) ;
#30058=FACE_OUTER_BOUND ( 'NONE', #21709, .T. ) ;
#30059=DIRECTION ( 'NONE',  ( -1.000000000000000000, 0.000000000000000000, 0.000000000000000000 ) ) ;
#30064=CARTESIAN_POINT ( 'NONE',  ( -16.81371235015666699, 2.650171115930294974, 19.41069149716887310 ) ) ;
#30066=ORIENTED_EDGE ( 'NONE', *, *, #27513, .T. ) ;
#30068=CARTESIAN_POINT ( 'NONE',  ( 11.40980092660686118, 6.310027164379057751, 1.500000000000001332 ) ) ;
#30072=CARTESIAN_POINT ( 'NONE',  ( -7.671865949551461838, -15.25812906914210032, 19.36813350477385143 ) ) ;
#30074=CARTESIAN_POINT ( 'NONE',  ( -5.544451647051929832, 16.11829164193972019, 7.652108011868850923 ) ) ;
#30075=AXIS2_PLACEMENT_3D ( 'NONE', #11375, #20869, #27601 ) ;
#30076=CARTESIAN_POINT ( 'NONE',  ( 1.438332125858173605, -8.884323311075778662, 1.500000000000001332 ) ) ;
#30080=CARTESIAN_POINT ( 'NONE',  ( 10.39243974596413089, -13.53611166824775935, 18.56793045041961321 ) ) ;
#30085=CARTESIAN_POINT ( 'NONE',  ( 13.00999358272542850, -0.8602714556717643291, 1.500000000000001332 ) ) ;
#30086=CARTESIAN_POINT ( 'NONE',  ( -5.512483845762028878, 16.12829592175436488, 5.651989602109218858 ) ) ;
#30087=VERTEX_POINT ( 'NONE', #12727 ) ;
#30090=DIRECTION ( 'NONE',  ( -0.000000000000000000, -0.000000000000000000, -1.000000000000000000 ) ) ;
#30102=ORIENTED_EDGE ( 'NONE', *, *, #1798, .F. ) ;
#30103=CARTESIAN_POINT ( 'NONE',  ( 3.529212228261832340, 16.69261290539734688, 7.500147780736496017 ) ) ;
#30105=CARTESIAN_POINT ( 'NONE',  ( 6.236311564447698075, 19.00292092786887110, 19.08232364404840453 ) ) ;
#30106=ORIENTED_EDGE ( 'NONE', *, *, #13942, .T. ) ;
#30109=CARTESIAN_POINT ( 'NONE',  ( 16.83479397774491915, 2.565335765644451094, 20.12545155307891065 ) ) ;
#30113=CARTESIAN_POINT ( 'NONE',  ( 15.38564065975360506, -7.280544306537537480, 6.755862304746362845 ) ) ;
#30114=CARTESIAN_POINT ( 'NONE',  ( -15.40675500887359028, 12.78077869785447440, 5.652605728828375753 ) ) ;
#30115=CARTESIAN_POINT ( 'NONE',  ( 3.064607854149369981, 16.80099270350294915, 19.47783254395485031 ) ) ;
#30120=CARTESIAN_POINT ( 'NONE',  ( -4.594331223478842929, 16.38995132059639204, 19.11611934778430921 ) ) ;
#30122=DIRECTION ( 'NONE',  ( 1.000000000000000000, 0.000000000000000000, 0.000000000000000000 ) ) ;
#30127=CARTESIAN_POINT ( 'NONE',  ( -16.96496223448355067, 1.652369715233091396, 7.652108011868850035 ) ) ;
#30129=CARTESIAN_POINT ( 'NONE',  ( 19.85631519639700215, 2.394924755340394285, 19.96302680909623817 ) ) ;
#30131=DIRECTION ( 'NONE',  ( 1.000000000000000000, 0.000000000000000000, 0.000000000000000000 ) ) ;
#30134=LINE ( 'NONE', #29527, #26213 ) ;
#30137=LINE ( 'NONE', #20474, #1354 ) ;
#30141=EDGE_CURVE ( 'NONE', #26457, #9428, #6844, .T. ) ;
#30143=DIRECTION ( 'NONE',  ( -0.2817325568414296710, 0.9594929736144973687, -0.000000000000000000 ) ) ;
#30147=EDGE_CURVE ( 'NONE', #1290, #11660, #15829, .T. ) ;
#30152=CARTESIAN_POINT ( 'NONE',  ( -4.574230723433014845, 16.39514892286268832, 6.519181285484531685 ) ) ;
#30162=CARTESIAN_POINT ( 'NONE',  ( -4.163336342344337027E-14, 1.387778780781445676E-14, 24.50000000000000000 ) ) ;
#30163=ORIENTED_EDGE ( 'NONE', *, *, #11319, .F. ) ;
#30167=CARTESIAN_POINT ( 'NONE',  ( 18.58529988941438305, 7.388276390372289448, 1.500000000000001332 ) ) ;
#30168=EDGE_CURVE ( 'NONE', #13757, #4954, #20357, .T. ) ;
#30169=ORIENTED_EDGE ( 'NONE', *, *, #6125, .T. ) ;
#30174=CARTESIAN_POINT ( 'NONE',  ( 19.72232476070952956, 3.323723214581398633, 20.34789198813115263 ) ) ;
#30176=CARTESIAN_POINT ( 'NONE',  ( 11.21631477658333687, -16.55933310271405645, 7.652108011868850923 ) ) ;
#30180=DIRECTION ( 'NONE',  ( 1.000000000000000000, 0.000000000000000000, 0.000000000000000000 ) ) ;
#30187=CARTESIAN_POINT ( 'NONE',  ( 16.17735844207722806, -3.336236224685152685, 1.500000000000000000 ) ) ;
#30188=DIRECTION ( 'NONE',  ( 0.9898214418809327952, -0.1423148382732850048, 0.000000000000000000 ) ) ;
#30189=LINE ( 'NONE', #27236, #17010 ) ;
#30190=CARTESIAN_POINT ( 'NONE',  ( 19.62935297797556089, -3.832558109936518687, 24.50000000000000000 ) ) ;
#30191=CARTESIAN_POINT ( 'NONE',  ( -18.29014699721057724, -8.135908015825712880, 20.19668224736330941 ) ) ;
#30192=CARTESIAN_POINT ( 'NONE',  ( -9.069887158720549181, -14.41355491440999437, 18.54473042795394377 ) ) ;
#30194=ORIENTED_EDGE ( 'NONE', *, *, #23991, .T. ) ;
#30195=ORIENTED_EDGE ( 'NONE', *, *, #19817, .F. ) ;
#30200=VERTEX_POINT ( 'NONE', #11155 ) ;
#30202=EDGE_CURVE ( 'NONE', #19910, #23254, #9839, .T. ) ;
#30206=ORIENTED_EDGE ( 'NONE', *, *, #25241, .F. ) ;
#30207=CARTESIAN_POINT ( 'NONE',  ( -11.33851205691660979, -16.47545820588254273, 19.60917204426170457 ) ) ;
#30209=AXIS2_PLACEMENT_3D ( 'NONE', #24373, #2556, #5047 ) ;
#30210=CARTESIAN_POINT ( 'NONE',  ( -10.80882669148404851, -16.84912922860908679, 18.39701043959520987 ) ) ;
#30213=ORIENTED_EDGE ( 'NONE', *, *, #4955, .F. ) ;
#30214=CARTESIAN_POINT ( 'NONE',  ( -14.70309389971832204, -8.688337726274227180, 6.783738457429057789 ) ) ;
#30215=CARTESIAN_POINT ( 'NONE',  ( -14.76283269969004230, 13.49301113316031042, 7.156831654632813233 ) ) ;
#30216=AXIS2_PLACEMENT_3D ( 'NONE', #3966, #1626, #13772 ) ;
#30221=CARTESIAN_POINT ( 'NONE',  ( 0.7788148826605766351, -17.02744010918315709, 7.652108011868850035 ) ) ;
#30222=VECTOR ( 'NONE', #3522, 1000.000000000000000 ) ;
#30225=CARTESIAN_POINT ( 'NONE',  ( -17.05621956093628810, 0.7704973847275167209, 19.85459532544247097 ) ) ;
#30227=CARTESIAN_POINT ( 'NONE',  ( -2.352830851074180440, -9.185733585337901630, 13.00000000000000178 ) ) ;
#30230=CARTESIAN_POINT ( 'NONE',  ( 10.05214800432092304, -13.77402237313446420, 18.37415474056476938 ) ) ;
#30233=ORIENTED_EDGE ( 'NONE', *, *, #4224, .F. ) ;
#30237=CARTESIAN_POINT ( 'NONE',  ( -5.655446062488478809, 19.20259930434394491, 5.701226463332907279 ) ) ;
#30238=ORIENTED_EDGE ( 'NONE', *, *, #11693, .T. ) ;
#30241=CARTESIAN_POINT ( 'NONE',  ( -13.37849590498012908, 10.56201291617988147, 7.652108011868850923 ) ) ;
#30245=CARTESIAN_POINT ( 'NONE',  ( 19.76052160831509852, 3.198927888535953112, 5.652196082367002994 ) ) ;
#30246=ORIENTED_EDGE ( 'NONE', *, *, #24041, .T. ) ;
#30247=CIRCLE ( 'NONE', #27268, 0.7500000000000015543 ) ;
#30249=EDGE_LOOP ( 'NONE', ( #20554, #1217, #25351, #3332 ) ) ;
#30251=ORIENTED_EDGE ( 'NONE', *, *, #1710, .T. ) ;
#30257=CIRCLE ( 'NONE', #18341, 9.482273699623480212 ) ;
#30258=LINE ( 'NONE', #8824, #24772 ) ;
#30259=CARTESIAN_POINT ( 'NONE',  ( 9.496768069075219643, -14.14083042221133368, 18.44501272782439827 ) ) ;
#30260=CARTESIAN_POINT ( 'NONE',  ( 19.79689803950977378, 2.967719242317201633, 20.32842677360128292 ) ) ;
#30264=CARTESIAN_POINT ( 'NONE',  ( 15.42605794595427682, -7.198932956632624780, 7.080843742048788414 ) ) ;
#30265=CIRCLE ( 'NONE', #13820, 20.00000000000000000 ) ;
#30266=CARTESIAN_POINT ( 'NONE',  ( -15.98738144660409866, 12.04609795553196960, 6.672349528511551497 ) ) ;
#30267=CARTESIAN_POINT ( 'NONE',  ( 4.365174083970718932, 19.53587658871429156, 19.03762469184452755 ) ) ;
#30268=ORIENTED_EDGE ( 'NONE', *, *, #7292, .F. ) ;
#30270=CIRCLE ( 'NONE', #15821, 9.482273699623480212 ) ;
#30271=CARTESIAN_POINT ( 'NONE',  ( 0.000000000000000000, 0.000000000000000000, 1.500000000000001332 ) ) ;
#30280=VECTOR ( 'NONE', #25395, 1000.000000000000114 ) ;
#30281=CARTESIAN_POINT ( 'NONE',  ( -17.02496544227784980, 1.117683430491698271, 7.500147780736496017 ) ) ;
#30285=ORIENTED_EDGE ( 'NONE', *, *, #7466, .T. ) ;
#30286=DIRECTION ( 'NONE',  ( 1.000000000000000000, 0.000000000000000000, 0.000000000000000000 ) ) ;
#30287=EDGE_LOOP ( 'NONE', ( #6474, #14553, #4891, #24413 ) ) ;
#30292=CARTESIAN_POINT ( 'NONE',  ( -0.6312581325461305015, -19.99009984789270433, 6.913388067999412634 ) ) ;
#30297=FACE_OUTER_BOUND ( 'NONE', #3696, .T. ) ;
#30299=CARTESIAN_POINT ( 'NONE',  ( 0.9279538312821420387, -17.02439129904410819, 7.643931100913408550 ) ) ;
#30305=ADVANCED_FACE ( 'NONE', ( #3524 ), #27388, .T. ) ;
#30307=CARTESIAN_POINT ( 'NONE',  ( -17.96015518819251255, -8.839856506746547993, 18.37415474056476938 ) ) ;
#30312=CARTESIAN_POINT ( 'NONE',  ( 7.730328572437743517, -4.608906612435629491, 1.500000000000001332 ) ) ;
#30316=DIRECTION ( 'NONE',  ( -0.4154150130018840481, 0.9096319953545194403, 0.000000000000000000 ) ) ;
#30318=FACE_OUTER_BOUND ( 'NONE', #21575, .T. ) ;
#30323=B_SPLINE_SURFACE_WITH_KNOTS ( 'NONE', 3, 1, ( 
 ( #11048, #30221 ),
 ( #2136, #6520 ),
 ( #6979, #11514 ),
 ( #1538, #6663 ),
 ( #28182, #16030 ),
 ( #25547, #20855 ),
 ( #30381, #4487 ),
 ( #11654, #18837 ),
 ( #28355, #16490 ),
 ( #26007, #13402 ),
 ( #9019, #18531 ),
 ( #28034, #25694 ),
 ( #4322, #18991 ),
 ( #14283, #12123 ),
 ( #29110, #560 ),
 ( #21776, #28959 ),
 ( #24271, #7594 ),
 ( #24112, #16792 ),
 ( #19286, #17255 ),
 ( #10080, #30828 ),
 ( #9625, #19136 ),
 ( #21623, #106 ),
 ( #28501, #12274 ),
 ( #9474, #28652 ),
 ( #415, #21465 ),
 ( #23958, #7751 ),
 ( #7444, #16644 ),
 ( #26466, #5098 ),
 ( #17099, #19442 ),
 ( #7133, #19593 ),
 ( #9933, #14456 ) ),
 .UNSPECIFIED., .F., .F., .F.,
 ( 4, 3, 3, 3, 3, 3, 3, 3, 3, 3, 4 ),
 ( 2, 2 ),
 ( 0.000000000000000000, 0.05425176834609633791, 0.1085332949128352958, 0.1623767749169382768, 0.2157504826133063158, 0.2688657508888171455, 0.3218907763505476360, 0.3749548578363336993, 0.4282048033836242107, 0.4818374082110501444, 0.4999999999131654604 ),
 ( 0.000000000000000000, 1.000000000000000000 ),
 .UNSPECIFIED. ) ;
#30327=CARTESIAN_POINT ( 'NONE',  ( 19.63503467057052632, 3.804509661152922106, 20.15039051365864253 ) ) ;
#30330=EDGE_CURVE ( 'NONE', #16378, #16205, #7264, .T. ) ;
#30331=CARTESIAN_POINT ( 'NONE',  ( -8.353478261420262285, -14.86569112999328901, 5.678370764302467677 ) ) ;
#30332=LINE ( 'NONE', #8672, #25311 ) ;
#30333=VECTOR ( 'NONE', #11780, 1000.000000000000227 ) ;
#30336=DIRECTION ( 'NONE',  ( 1.000000000000000000, 0.000000000000000000, 0.000000000000000000 ) ) ;
#30337=DIRECTION ( 'NONE',  ( 1.000000000000000000, 0.000000000000000000, 0.000000000000000000 ) ) ;
#30339=LINE ( 'NONE', #28150, #10297 ) ;
#30340=CIRCLE ( 'NONE', #11, 1.000000000000000888 ) ;
#30341=CARTESIAN_POINT ( 'NONE',  ( -15.56507824124931894, -6.890134373242267962, 19.60617949693493145 ) ) ;
#30344=CARTESIAN_POINT ( 'NONE',  ( 3.062151163506447116, 16.80153468414596674, 19.28454053338348828 ) ) ;
#30346=EDGE_CURVE ( 'NONE', #26457, #14352, #25784, .T. ) ;
#30351=ORIENTED_EDGE ( 'NONE', *, *, #15480, .F. ) ;
#30356=EDGE_CURVE ( 'NONE', #606, #10785, #28281, .T. ) ;
#30364=ORIENTED_EDGE ( 'NONE', *, *, #27256, .T. ) ;
#30365=CARTESIAN_POINT ( 'NONE',  ( -16.89118935510124331, 2.183074208216230883, 5.796888747622817029 ) ) ;
#30367=VECTOR ( 'NONE', #15952, 1000.000000000000000 ) ;
#30369=DIRECTION ( 'NONE',  ( -0.000000000000000000, -0.000000000000000000, 1.000000000000000000 ) ) ;
#30371=EDGE_LOOP ( 'NONE', ( #723, #1850 ) ) ;
#30376=CARTESIAN_POINT ( 'NONE',  ( -6.587096388939656322, -18.88412458026101604, 1.500000000000001332 ) ) ;
#30381=CARTESIAN_POINT ( 'NONE',  ( -0.2861250491275375563, -20.01582202454545723, 7.429667576816606278 ) ) ;
#30385=LINE ( 'NONE', #9316, #29945 ) ;
#30390=CARTESIAN_POINT ( 'NONE',  ( 10.45210396439253842, -13.49311571392156495, 20.06253562465620632 ) ) ;
#30393=EDGE_CURVE ( 'NONE', #21089, #17934, #19837, .T. ) ;
#30395=DIRECTION ( 'NONE',  ( 1.000000000000000000, 0.000000000000000000, 0.000000000000000000 ) ) ;
#30396=DIRECTION ( 'NONE',  ( 0.000000000000000000, 0.000000000000000000, 1.000000000000000000 ) ) ;
#30397=VERTEX_POINT ( 'NONE', #17503 ) ;
#30398=CARTESIAN_POINT ( 'NONE',  ( -11.64054540341807353, 16.26338533980437262, 24.50000000000000000 ) ) ;
#30399=DIRECTION ( 'NONE',  ( -0.000000000000000000, -1.000000000000000000, -0.000000000000000000 ) ) ;
#30402=VECTOR ( 'NONE', #18133, 1000.000000000000000 ) ;
#30410=EDGE_CURVE ( 'NONE', #23733, #9215, #15435, .T. ) ;
#30412=CARTESIAN_POINT ( 'NONE',  ( -15.34618562042307310, 12.82554431217321245, 5.652196082369965069 ) ) ;
#30414=CARTESIAN_POINT ( 'NONE',  ( 9.263624429760991319, -14.28705663139043125, 18.63641924841378028 ) ) ;
#30415=FACE_OUTER_BOUND ( 'NONE', #11894, .T. ) ;
#30417=CARTESIAN_POINT ( 'NONE',  ( -19.83108769839776997, 2.729924941536435945, 20.32842677360128292 ) ) ;
#30420=CARTESIAN_POINT ( 'NONE',  ( -13.91614452448631667, 9.890357823660679060, 7.196036389296800451 ) ) ;
#30421=CARTESIAN_POINT ( 'NONE',  ( 3.718735505629739091, 16.64535199026475709, 18.39992786714538298 ) ) ;
#30422=ORIENTED_EDGE ( 'NONE', *, *, #27340, .F. ) ;
#30425=CARTESIAN_POINT ( 'NONE',  ( 10.58714538947712924, -13.39479915612166572, 7.158811349119582168 ) ) ;
#30426=B_SPLINE_CURVE_WITH_KNOTS ( 'NONE', 3,
 ( #26186, #16677, #21034, #14025, #4668, #23987, #28217, #14331, #30557, #23842, #19167, #25886, #7166, #23527, #137, #28385 ),
 .UNSPECIFIED., .F., .F.,
 ( 4, 2, 2, 2, 2, 2, 2, 4 ),
 ( 0.4999999999999999445, 0.6250000000000008882, 0.6875000000000015543, 0.7187500000000019984, 0.7500000000000022204, 0.8125000000000013323, 0.8750000000000004441, 1.000000000000000000 ),
 .UNSPECIFIED. ) ;
#30427=CARTESIAN_POINT ( 'NONE',  ( -5.762218391735197898, 19.17087124927422792, 18.36582235739946611 ) ) ;
#30432=CARTESIAN_POINT ( 'NONE',  ( -17.06456206750265281, 0.6636403356599883674, 6.892848776733236704 ) ) ;
#30433=CARTESIAN_POINT ( 'NONE',  ( 14.27394986618626582, 14.00917565527016073, 18.84486140012299771 ) ) ;
#30434=CARTESIAN_POINT ( 'NONE',  ( 19.87925100141002233, 2.194397331962204767, 19.21471108562414543 ) ) ;
#30437=ORIENTED_EDGE ( 'NONE', *, *, #26181, .F. ) ;
#30438=CARTESIAN_POINT ( 'NONE',  ( 18.63200854944940232, -7.318485330915429188, 5.951255046771932733 ) ) ;
#30445=DIRECTION ( 'NONE',  ( 0.1423148382732851158, 0.9898214418809327952, 0.000000000000000000 ) ) ;
#30446=CARTESIAN_POINT ( 'NONE',  ( -5.861334694664002143, 16.01657976118487881, 20.29915277494337644 ) ) ;
#30453=CARTESIAN_POINT ( 'NONE',  ( 19.74250593591595049, 3.198927889078816644, 18.34798005863227388 ) ) ;
#30455=VECTOR ( 'NONE', #19814, 1000.000000000000000 ) ;
#30458=CYLINDRICAL_SURFACE ( 'NONE', #12924, 20.00000000000000000 ) ;
#30461=CYLINDRICAL_SURFACE ( 'NONE', #22539, 20.00000000000000000 ) ;
#30462=EDGE_LOOP ( 'NONE', ( #22809, #21150, #10954, #8422 ) ) ;
#30466=VERTEX_POINT ( 'NONE', #3774 ) ;
#30474=ORIENTED_EDGE ( 'NONE', *, *, #16757, .F. ) ;
#30475=LINE ( 'NONE', #15673, #12826 ) ;
#30476=ADVANCED_FACE ( 'NONE', ( #13294 ), #21096, .T. ) ;
#30477=DIRECTION ( 'NONE',  ( 0.000000000000000000, 0.000000000000000000, 1.000000000000000000 ) ) ;
#30482=CARTESIAN_POINT ( 'NONE',  ( -10.51513057463695233, -17.01270198993486460, 7.652108011868850035 ) ) ;
#30484=CARTESIAN_POINT ( 'NONE',  ( -13.21131958021068087, 10.75991052173289120, 18.37259980046033547 ) ) ;
#30486=CARTESIAN_POINT ( 'NONE',  ( 3.540451764476295171, 16.69076635156335797, 20.24143955528809258 ) ) ;
#30489=CARTESIAN_POINT ( 'NONE',  ( -18.43827498451963365, -7.794211480880301579, 19.77662771831109367 ) ) ;
#30491=VERTEX_POINT ( 'NONE', #4830 ) ;
#30498=CARTESIAN_POINT ( 'NONE',  ( 15.76678477342441020, -6.469363178373285450, 20.34789198813115263 ) ) ;
#30499=CARTESIAN_POINT ( 'NONE',  ( 4.049916830765392994, 16.55712665160099561, 7.652108011868850035 ) ) ;
#30501=CARTESIAN_POINT ( 'NONE',  ( -10.51513057463694523, -17.01270198993485394, 20.34789198813115263 ) ) ;
#30505=ORIENTED_EDGE ( 'NONE', *, *, #29018, .T. ) ;
#30506=CARTESIAN_POINT ( 'NONE',  ( 0.000000000000000000, 0.000000000000000000, 1.500000000000001332 ) ) ;
#30511=CIRCLE ( 'NONE', #19050, 9.482273699623480212 ) ;
#30513=DIRECTION ( 'NONE',  ( 1.000000000000000000, 0.000000000000000000, 0.000000000000000000 ) ) ;
#30515=ADVANCED_FACE ( 'NONE', ( #14346 ), #16383, .T. ) ;
#30516=CARTESIAN_POINT ( 'NONE',  ( 0.4564504349074266498, -9.471281197126616647, 1.500000000000001332 ) ) ;
#30524=VERTEX_POINT ( 'NONE', #21509 ) ;
#30525=EDGE_CURVE ( 'NONE', #24284, #17232, #16346, .T. ) ;
#30526=CARTESIAN_POINT ( 'NONE',  ( -6.312773474750901670, 15.86096687812979233, 7.269896094239230777 ) ) ;
#30531=EDGE_LOOP ( 'NONE', ( #15270, #15746, #73, #3021 ) ) ;
#30538=ORIENTED_EDGE ( 'NONE', *, *, #25270, .T. ) ;
#30539=CARTESIAN_POINT ( 'NONE',  ( 15.12016594919360557, 13.11846484362264498, 20.29090034784956131 ) ) ;
#30549=EDGE_CURVE ( 'NONE', #4276, #22425, #1689, .T. ) ;
#30552=VERTEX_POINT ( 'NONE', #17469 ) ;
#30554=ADVANCED_FACE ( 'NONE', ( #26991, #19491, #17147 ), #26667, .T. ) ;
#30556=CARTESIAN_POINT ( 'NONE',  ( 6.587096388939653657, -18.88412458026098406, 1.500000000000001332 ) ) ;
#30557=CARTESIAN_POINT ( 'NONE',  ( -14.70303524442681642, -8.688445896238670585, 19.28454053338348473 ) ) ;
#30558=CARTESIAN_POINT ( 'NONE',  ( 1.307979816482770286, -17.01201364160834117, 18.45571264222803975 ) ) ;
#30559=CARTESIAN_POINT ( 'NONE',  ( 16.79398274391851942, 2.865066961627989350, 18.39701043959520987 ) ) ;
#30562=CARTESIAN_POINT ( 'NONE',  ( -16.87659098782771494, 2.276273425076630552, 18.55820869691756769 ) ) ;
#30564=CARTESIAN_POINT ( 'NONE',  ( -13.37849590052435289, 10.56201291103764284, 20.34789198813115263 ) ) ;
#30565=CARTESIAN_POINT ( 'NONE',  ( 3.436936369909011635, 16.71530215271315711, 20.13759033520874908 ) ) ;
#30566=ORIENTED_EDGE ( 'NONE', *, *, #5575, .F. ) ;
#30567=ORIENTED_EDGE ( 'NONE', *, *, #14717, .T. ) ;
#30570=CARTESIAN_POINT ( 'NONE',  ( -5.439684697860717399, 16.15075171424583900, 18.35377592296120497 ) ) ;
#30574=DIRECTION ( 'NONE',  ( 0.000000000000000000, 0.000000000000000000, -1.000000000000000000 ) ) ;
#30575=EDGE_CURVE ( 'NONE', #22188, #8257, #611, .T. ) ;
#30578=EDGE_CURVE ( 'NONE', #4691, #22613, #7892, .T. ) ;
#30579=CARTESIAN_POINT ( 'NONE',  ( -17.04940614979728508, 0.8516807413325234721, 6.041646659195333058 ) ) ;
#30581=CARTESIAN_POINT ( 'NONE',  ( 19.86493687747362102, 2.320961355260791059, 19.85261563089511938 ) ) ;
#30585=LINE ( 'NONE', #7034, #1978 ) ;
#30591=PLANE ( 'NONE',  #2395 ) ;
#30592=CARTESIAN_POINT ( 'NONE',  ( -5.544451646083596863, 16.11829163520481956, 20.34789198813115263 ) ) ;
#30593=LINE ( 'NONE', #28421, #20781 ) ;
#30594=LINE ( 'NONE', #11728, #16833 ) ;
#30596=CARTESIAN_POINT ( 'NONE',  ( 15.70758541206079428, -6.601999697740968287, 5.676815824193229609 ) ) ;
#30597=DIRECTION ( 'NONE',  ( 0.000000000000000000, 0.000000000000000000, 1.000000000000000000 ) ) ;
#30599=ORIENTED_EDGE ( 'NONE', *, *, #9565, .F. ) ;
#30601=CARTESIAN_POINT ( 'NONE',  ( -14.96594037876677596, -8.187306180225535357, 18.44527579819791185 ) ) ;
#30605=DIRECTION ( 'NONE',  ( -0.000000000000000000, -0.000000000000000000, 1.000000000000000000 ) ) ;
#30608=CARTESIAN_POINT ( 'NONE',  ( -6.453144054752231185, 18.93070788617552580, 7.528076282304596134 ) ) ;
#30611=DIRECTION ( 'NONE',  ( 0.5406408174555974444, 0.8412535328311813165, 0.000000000000000000 ) ) ;
#30612=CARTESIAN_POINT ( 'NONE',  ( -4.163336342344337027E-14, 1.387778780781445676E-14, 24.50000000000000000 ) ) ;
#30614=AXIS2_PLACEMENT_3D ( 'NONE', #21558, #195, #29207 ) ;
#30615=EDGE_LOOP ( 'NONE', ( #17318, #28869, #60, #10243 ) ) ;
#30617=ORIENTED_EDGE ( 'NONE', *, *, #14115, .F. ) ;
#30618=CARTESIAN_POINT ( 'NONE',  ( -0.01062192699083570196, -17.02590662965304347, 18.71435384576123440 ) ) ;
#30619=CARTESIAN_POINT ( 'NONE',  ( -10.46366670609033100, -17.06541516851461182, 7.652108011868850035 ) ) ;
#30622=CARTESIAN_POINT ( 'NONE',  ( 1.230359340266123702, -17.01462811240319795, 18.44527579819791185 ) ) ;
#30623=ORIENTED_EDGE ( 'NONE', *, *, #11683, .T. ) ;
#30625=CARTESIAN_POINT ( 'NONE',  ( 16.70106355290778666, 3.455140589294515063, 7.652108011868851811 ) ) ;
#30631=CARTESIAN_POINT ( 'NONE',  ( -15.49717968187447603, -7.050617358802334422, 18.72771030977187579 ) ) ;
#30636=CARTESIAN_POINT ( 'NONE',  ( -18.45576848551221616, -7.706141034055812966, 19.21471108562414898 ) ) ;
#30638=ORIENTED_EDGE ( 'NONE', *, *, #13745, .F. ) ;
#30642=CARTESIAN_POINT ( 'NONE',  ( -3.662523238938586001, -12.47340865698848056, 1.500000000000001332 ) ) ;
#30644=CARTESIAN_POINT ( 'NONE',  ( 15.54925513364909406, -6.943479002078025708, 20.12545155307891065 ) ) ;
#30646=CARTESIAN_POINT ( 'NONE',  ( 4.971436688744669041, 16.28007576866362882, 6.974106381145714018 ) ) ;
#30648=CARTESIAN_POINT ( 'NONE',  ( 6.218621694205434203, 19.02754758079138853, 19.00652017443069752 ) ) ;
#30652=ORIENTED_EDGE ( 'NONE', *, *, #17459, .T. ) ;
#30659=DIRECTION ( 'NONE',  ( 0.000000000000000000, 0.000000000000000000, -1.000000000000000000 ) ) ;
#30660=CARTESIAN_POINT ( 'NONE',  ( 16.78337223357198482, 2.938206247954857631, 18.37259980046034258 ) ) ;
#30664=B_SPLINE_CURVE_WITH_KNOTS ( 'NONE', 3,
 ( #2689, #24359, #5335, #21400, #4872, #16724, #21547, #40, #2540, #28433, #21868, #341, #28583, #4715, #17032, #183, #14687, #10022, #14216, #17184 ),
 .UNSPECIFIED., .F., .F.,
 ( 4, 2, 2, 2, 2, 2, 2, 2, 2, 4 ),
 ( 0.000000000000000000, 0.06249999999999988898, 0.1249999999999997780, 0.1874999999999996669, 0.2187499999999995282, 0.2499999999999993339, 0.3124999999999994449, 0.3749999999999995559, 0.4374999999999996669, 0.4999999999999997780 ),
 .UNSPECIFIED. ) ;
#30668=CARTESIAN_POINT ( 'NONE',  ( 8.743977807160073112, 3.668292057956029861, 13.00000000000000178 ) ) ;
#30672=PLANE ( 'NONE',  #9762 ) ;
#30673=DIRECTION ( 'NONE',  ( -0.2817325568414292825, -0.9594929736144974797, 0.000000000000000000 ) ) ;
#30674=ORIENTED_EDGE ( 'NONE', *, *, #21356, .T. ) ;
#30675=VERTEX_POINT ( 'NONE', #26836 ) ;
#30679=CARTESIAN_POINT ( 'NONE',  ( 12.72536390617885438, -2.839914339433650348, 1.500000000000001332 ) ) ;
#30683=CARTESIAN_POINT ( 'NONE',  ( 12.58124959699792456, 11.48680237977196228, 20.29090034784956131 ) ) ;
#30686=EDGE_CURVE ( 'NONE', #17274, #4954, #12884, .T. ) ;
#30689=DIRECTION ( 'NONE',  ( 0.000000000000000000, 0.000000000000000000, -1.000000000000000000 ) ) ;
#30693=EDGE_CURVE ( 'NONE', #8468, #29572, #29479, .T. ) ;
#30694=ORIENTED_EDGE ( 'NONE', *, *, #2427, .F. ) ;
#30699=CARTESIAN_POINT ( 'NONE',  ( -17.64259547893121649, -9.420269215336073643, 6.149077423860703995 ) ) ;
#30700=AXIS2_PLACEMENT_3D ( 'NONE', #24975, #29511, #15456 ) ;
#30701=CARTESIAN_POINT ( 'NONE',  ( 15.41296542101254552, 5.939519782021115191, 1.500000000000000000 ) ) ;
#30702=CARTESIAN_POINT ( 'NONE',  ( 0.7788148816922458861, -17.02744011591804707, 20.34789198813115263 ) ) ;
#30704=EDGE_LOOP ( 'NONE', ( #3193, #4190, #27064, #12339 ) ) ;
#30705=CARTESIAN_POINT ( 'NONE',  ( -19.72724879956887278, 3.398799651952296053, 18.90679857307105749 ) ) ;
#30711=ORIENTED_EDGE ( 'NONE', *, *, #25839, .F. ) ;
#30714=ADVANCED_FACE ( 'NONE', ( #14653 ), #14135, .T. ) ;
#30726=ADVANCED_FACE ( 'NONE', ( #17769 ), #13103, .F. ) ;
#30728=CARTESIAN_POINT ( 'NONE',  ( -17.05537006572908609, 0.7816414089123764342, 6.131018562779544823 ) ) ;
#30729=CARTESIAN_POINT ( 'NONE',  ( 14.70074466696773996, 13.56107787884953630, 18.37545668562166412 ) ) ;
#30733=CYLINDRICAL_SURFACE ( 'NONE', #3872, 1.000000000000007772 ) ;
#30738=DIRECTION ( 'NONE',  ( 1.000000000000000000, 0.000000000000000000, 0.000000000000000000 ) ) ;
#30740=ORIENTED_EDGE ( 'NONE', *, *, #29385, .T. ) ;
#30744=CARTESIAN_POINT ( 'NONE',  ( 10.29773160325293979, -13.60426929937658436, 18.45571264222803975 ) ) ;
#30746=CARTESIAN_POINT ( 'NONE',  ( -4.163336342344337027E-14, 1.387778780781445676E-14, 24.50000000000000000 ) ) ;
#30751=ORIENTED_EDGE ( 'NONE', *, *, #21958, .T. ) ;
#30759=CARTESIAN_POINT ( 'NONE',  ( -14.73262409220165203, -8.633676228711859579, 19.69140814234746273 ) ) ;
#30760=EDGE_CURVE ( 'NONE', #5874, #6566, #11820, .T. ) ;
#30761=AXIS2_PLACEMENT_3D ( 'NONE', #14996, #12679, #29043 ) ;
#30762=DIRECTION ( 'NONE',  ( -0.000000000000000000, -0.000000000000000000, 1.000000000000000000 ) ) ;
#30767=ORIENTED_EDGE ( 'NONE', *, *, #9944, .T. ) ;
#30771=CARTESIAN_POINT ( 'NONE',  ( -6.962021646281573162, -6.437683520590147701, 21.50000000000000000 ) ) ;
#30774=CARTESIAN_POINT ( 'NONE',  ( 7.869584159753955532, 10.39565510934977333, 1.500000000000001332 ) ) ;
#30779=ORIENTED_EDGE ( 'NONE', *, *, #19079, .T. ) ;
#30780=CARTESIAN_POINT ( 'NONE',  ( 0.6691466709101893118, -17.02906906675068299, 18.35377592296120497 ) ) ;
#30782=CARTESIAN_POINT ( 'NONE',  ( 9.406652940105985294, -1.195154792889423057, 13.00000000000000178 ) ) ;
#30785=CARTESIAN_POINT ( 'NONE',  ( 0.3493067888074719574, -20.01473451864463371, 20.34789198813115263 ) ) ;
#30789=DIRECTION ( 'NONE',  ( -0.1423148382732853101, 0.9898214418809327952, 0.000000000000000000 ) ) ;
#30790=CARTESIAN_POINT ( 'NONE',  ( 14.20930976959225589, 14.09970620734104862, 19.14333282897057842 ) ) ;
#30791=CARTESIAN_POINT ( 'NONE',  ( 19.74250593591594694, 3.198927889078816644, 5.652196082369963293 ) ) ;
#30795=LINE ( 'NONE', #16752, #8319 ) ;
#30796=CARTESIAN_POINT ( 'NONE',  ( -13.05132497920497237, 10.94401179279849323, 18.47056384035244037 ) ) ;
#30801=ORIENTED_EDGE ( 'NONE', *, *, #16048, .T. ) ;
#30807=FACE_OUTER_BOUND ( 'NONE', #6038, .T. ) ;
#30808=EDGE_LOOP ( 'NONE', ( #5950, #1180 ) ) ;
#30810=AXIS2_PLACEMENT_3D ( 'NONE', #5065, #75, #24390 ) ;
#30811=CARTESIAN_POINT ( 'NONE',  ( 15.67520293387195807, -6.672517015027191967, 20.29090034784956131 ) ) ;
#30812=VECTOR ( 'NONE', #29729, 1000.000000000000000 ) ;
#30813=CARTESIAN_POINT ( 'NONE',  ( 4.654893560761754756, 16.38086414125081802, 5.862424720655265098 ) ) ;
#30814=ORIENTED_EDGE ( 'NONE', *, *, #1000, .F. ) ;
#30815=CARTESIAN_POINT ( 'NONE',  ( 11.73047935159229915, 12.40726572549740325, 7.098451512883313441 ) ) ;
#30820=DIRECTION ( 'NONE',  ( 0.7557495743542582689, -0.6548607339452851006, 0.000000000000000000 ) ) ;
#30825=CARTESIAN_POINT ( 'NONE',  ( -18.15888143814677136, -8.424936462863948705, 7.632642797338977658 ) ) ;
#30826=CARTESIAN_POINT ( 'NONE',  ( 16.74328841314636662, 3.194145055459935545, 20.34789198813115263 ) ) ;
#30828=CARTESIAN_POINT ( 'NONE',  ( -0.07785784566753103930, -17.02422498921964689, 6.111214848085761986 ) ) ;
#30829=CIRCLE ( 'NONE', #10928, 0.7500000000000006661 ) ;
#30830=CARTESIAN_POINT ( 'NONE',  ( -8.999114229549592281, 0.1262659238205133538, 1.500000000000001332 ) ) ;
#30832=CARTESIAN_POINT ( 'NONE',  ( -19.95437879344081011, 1.590546279198205237, 19.79423548914561692 ) ) ;
#30835=CARTESIAN_POINT ( 'NONE',  ( 11.11463800144301928, -16.64861661464430398, 20.34789198813115263 ) ) ;
#30838=ORIENTED_EDGE ( 'NONE', *, *, #6483, .F. ) ;
#30839=VERTEX_POINT ( 'NONE', #21156 ) ;
#30846=CARTESIAN_POINT ( 'NONE',  ( 18.65775367615955460, -7.252215724661033036, 18.73743063545763121 ) ) ;
#30847=CARTESIAN_POINT ( 'NONE',  ( 19.60273500773784860, 4.055073576757204812, 18.82680253904184298 ) ) ;
#30849=EDGE_LOOP ( 'NONE', ( #8609, #1737, #27578, #30801 ) ) ;
#30852=VECTOR ( 'NONE', #16279, 1000.000000000000000 ) ;
#30854=EDGE_CURVE ( 'NONE', #24660, #19294, #27331, .T. ) ;
#30856=CARTESIAN_POINT ( 'NONE',  ( -0.2239719228509424731, -17.01994463034878891, 19.47784884541372818 ) ) ;
#30908=COLOUR_RGB('Off White',0.89,0.88,0.83);
#30909=FILL_AREA_STYLE_COLOUR('',#30908);
#30910=FILL_AREA_STYLE('',(#30909));
#30911=SURFACE_STYLE_FILL_AREA(#30910);
#30912=SURFACE_SIDE_STYLE('',(#30911));
#30913=SURFACE_STYLE_USAGE(.BOTH.,#30912);
#30914=PRESENTATION_STYLE_ASSIGNMENT((#30913));
ENDSEC;
END-ISO-10303-21;
